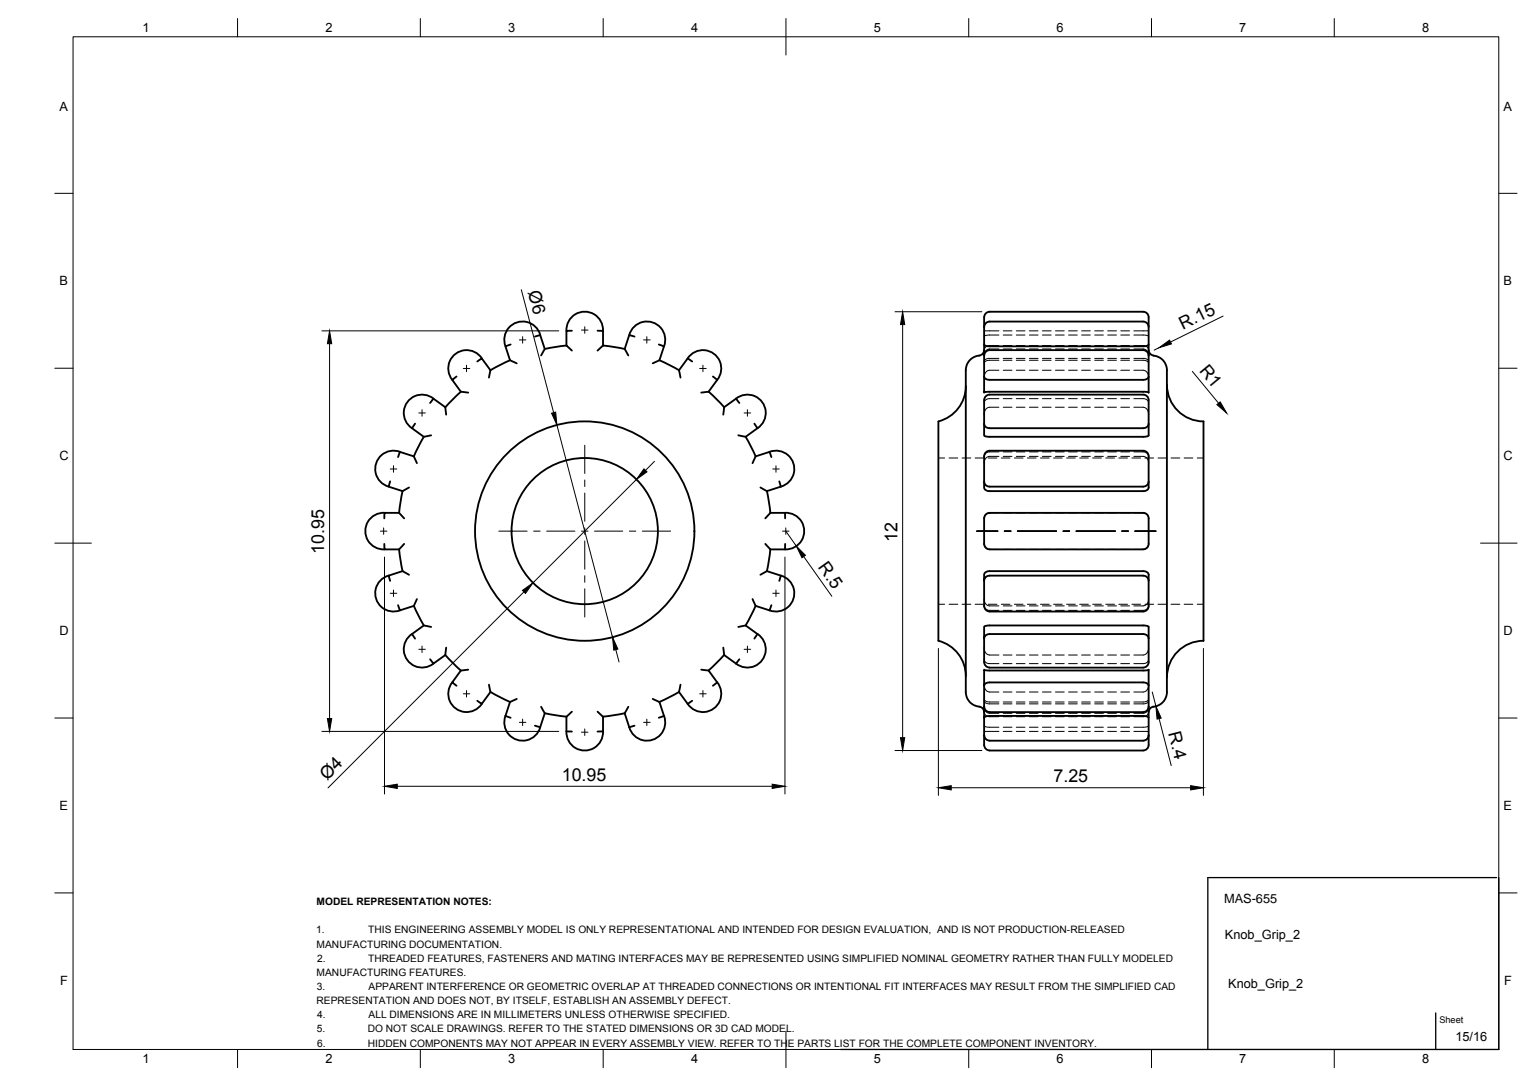
ISO-10303-21;
HEADER;
FILE_DESCRIPTION((''),'2;1');
FILE_NAME('Knob_Grip_2.step','2026-10-09T11:34:15-07:00',(''),(''),'','','');
FILE_SCHEMA (('AUTOMOTIVE_DESIGN { 1 0 10303 214 3 1 1 }'));
ENDSEC;
DATA;
#10=MECHANICAL_DESIGN_GEOMETRIC_PRESENTATION_REPRESENTATION('',(#647),#117170);
#605=SHAPE_REPRESENTATION_RELATIONSHIP('SRR','None',#117260,#626) ;
#626=ADVANCED_BREP_SHAPE_REPRESENTATION('',(#668),#117168) ;
#647=STYLED_ITEM('',(#117355),#668) ;
#668=MANIFOLD_SOLID_BREP('Body1',#49076) ;
#766=FACE_BOUND('',#16715,.T.) ;
#767=FACE_BOUND('',#16718,.T.) ;
#768=FACE_BOUND('',#16720,.T.) ;
#769=FACE_BOUND('',#16722,.T.) ;
#1529=B_SPLINE_CURVE_WITH_KNOTS('',3,(#105473,#105474,#105475,#105476,#105477,
#105478,#105479,#105480,#105481,#105482,#105483,#105484,#105485,#105486,
#105487,#105488,#105489),.UNSPECIFIED.,.T.,.F.,(4,1,1,1,1,1,1,1,1,1,1,1,
1,1,4),(-1.37470975898194,-1.17832265055595,-0.981935542129957,-0.785548433703966,
-0.589161325277974,-0.392774216851983,-0.196387108425991,0.,0.196387108425991,
0.392774216851983,0.589161325277974,0.785548433703966,0.981935542129957,
1.17832265055595,1.37470975898194),.UNSPECIFIED.) ;
#1530=B_SPLINE_CURVE_WITH_KNOTS('',3,(#105498,#105499,#105500,#105501,#105502,
#105503,#105504,#105505,#105506,#105507,#105508,#105509,#105510,#105511,
#105512,#105513,#105514),.UNSPECIFIED.,.T.,.F.,(4,1,1,1,1,1,1,1,1,1,1,1,
1,1,4),(-1.37470975898194,-1.17832265055595,-0.981935542129957,-0.785548433703966,
-0.589161325277974,-0.392774216851983,-0.196387108425991,0.,0.196387108425991,
0.392774216851983,0.589161325277974,0.785548433703966,0.981935542129957,
1.17832265055595,1.37470975898194),.UNSPECIFIED.) ;
#1531=B_SPLINE_CURVE_WITH_KNOTS('',3,(#105607,#105608,#105609,#105610,#105611),
 .UNSPECIFIED.,.F.,.F.,(4,1,4),(-1.,-0.5,0.),.UNSPECIFIED.) ;
#1532=B_SPLINE_CURVE_WITH_KNOTS('',3,(#105613,#105614,#105615,#105616,#105617,
#105618,#105619),.UNSPECIFIED.,.F.,.F.,(4,1,1,1,4),(-1.37470975898194,-1.17832265055595,
-0.981935542129957,-0.785548433703966,-0.687133244560913),.UNSPECIFIED.) ;
#1533=B_SPLINE_CURVE_WITH_KNOTS('',3,(#105620,#105621,#105622,#105623,#105624,
#105625,#105626,#105627,#105628,#105629,#105630,#105631,#105632,#105633),
 .UNSPECIFIED.,.F.,.F.,(4,1,1,1,1,1,1,1,1,1,1,4),(-0.687133244560913,-0.589161325277974,
-0.392774216851983,-0.196387108425991,0.,0.196387108425991,0.392774216851983,
0.589161325277974,0.785548433703966,0.981935542129957,1.17832265055595,
1.37470975898194),.UNSPECIFIED.) ;
#1534=B_SPLINE_CURVE_WITH_KNOTS('',3,(#105720,#105721,#105722,#105723,#105724),
 .UNSPECIFIED.,.F.,.F.,(4,1,4),(-1.,-0.5,0.),.UNSPECIFIED.) ;
#1535=B_SPLINE_CURVE_WITH_KNOTS('',3,(#105726,#105727,#105728,#105729,#105730,
#105731,#105732),.UNSPECIFIED.,.F.,.F.,(4,1,1,1,4),(-1.37470975898194,-1.17832265055595,
-0.981935542129957,-0.785548433703966,-0.687210817221059),.UNSPECIFIED.) ;
#1536=B_SPLINE_CURVE_WITH_KNOTS('',3,(#105733,#105734,#105735,#105736,#105737,
#105738,#105739,#105740,#105741,#105742,#105743,#105744,#105745,#105746),
 .UNSPECIFIED.,.F.,.F.,(4,1,1,1,1,1,1,1,1,1,1,4),(-0.687210817221059,-0.589161325277974,
-0.392774216851983,-0.196387108425991,0.,0.196387108425991,0.392774216851983,
0.589161325277974,0.785548433703966,0.981935542129957,1.17832265055595,
1.37470975898194),.UNSPECIFIED.) ;
#1537=B_SPLINE_CURVE_WITH_KNOTS('',3,(#105752,#105753,#105754,#105755,#105756,
#105757,#105758,#105759,#105760,#105761,#105762,#105763,#105764,#105765),
 .UNSPECIFIED.,.F.,.F.,(4,2,2,2,2,2,4),(-0.0559250143496373,-0.0556883945460747,
-0.0495906031992305,-0.0437546843030053,-0.0372885759081072,-0.0322854917709823,
-0.0278441972730634),.UNSPECIFIED.) ;
#1538=B_SPLINE_CURVE_WITH_KNOTS('',3,(#105768,#105769,#105770,#105771,#105772,
#105773,#105774,#105775,#105776,#105777,#105778,#105779,#105780,#105781),
 .UNSPECIFIED.,.F.,.F.,(4,2,2,2,2,2,4),(-0.000236619804093,0.,0.0060977913471935,
0.0119337102438738,0.018399818639261,0.0234029027767472,0.0278441972749678),
 .UNSPECIFIED.) ;
#1539=B_SPLINE_CURVE_WITH_KNOTS('',3,(#105786,#105787,#105788,#105789,#105790,
#105791,#105792,#105793,#105794,#105795,#105796,#105797,#105798,#105799,
#105800,#105801),.UNSPECIFIED.,.F.,.F.,(4,3,3,3,3,4),(-0.000437598556087367,
0.,0.00562170475705654,0.0114823251607832,0.0173413775084489,0.0231997078489075),
 .UNSPECIFIED.) ;
#1540=B_SPLINE_CURVE_WITH_KNOTS('',3,(#105807,#105808,#105809,#105810,#105811,
#105812,#105813,#105814,#105815,#105816,#105817,#105818,#105819,#105820,
#105821,#105822),.UNSPECIFIED.,.F.,.F.,(4,3,3,3,3,4),(-0.046837014255361,
-0.046399415699481,-0.0407777109422933,-0.0349170905383532,-0.0290580381904547,
-0.0231997078497599),.UNSPECIFIED.) ;
#1541=B_SPLINE_CURVE_WITH_KNOTS('',3,(#105828,#105829,#105830,#105831,#105832,
#105833,#105834,#105835,#105836,#105837,#105838,#105839,#105840,#105841),
 .UNSPECIFIED.,.F.,.F.,(4,2,2,2,2,2,4),(-0.000236619803146698,0.,0.00609779134724104,
0.0119337102438844,0.0183998186389394,0.0234029027761802,0.0278441972742087),
 .UNSPECIFIED.) ;
#1542=B_SPLINE_CURVE_WITH_KNOTS('',3,(#105847,#105848,#105849,#105850,#105851,
#105852,#105853,#105854,#105855,#105856,#105857,#105858,#105859,#105860),
 .UNSPECIFIED.,.F.,.F.,(4,2,2,2,2,2,4),(-0.0559250143496986,-0.0556883945465552,
-0.0495906031994403,-0.0437546843028884,-0.0372885759079096,-0.0322854917707418,
-0.0278441972727803),.UNSPECIFIED.) ;
#1543=B_SPLINE_CURVE_WITH_KNOTS('',3,(#105866,#105867,#105868,#105869,#105870,
#105871,#105872,#105873,#105874,#105875,#105876,#105877,#105878,#105879,
#105880,#105881),.UNSPECIFIED.,.F.,.F.,(4,3,3,3,3,4),(-0.000437598556095027,
0.,0.00562170475708189,0.0114823251608833,0.0173413775086171,0.0231997078491342),
 .UNSPECIFIED.) ;
#1544=B_SPLINE_CURVE_WITH_KNOTS('',3,(#105887,#105888,#105889,#105890,#105891,
#105892,#105893,#105894,#105895,#105896,#105897,#105898,#105899,#105900,
#105901,#105902),.UNSPECIFIED.,.F.,.F.,(4,3,3,3,3,4),(-0.0468370142541051,
-0.0463994156980201,-0.0407777109409428,-0.0349170905371886,-0.0290580381894966,
-0.0231997078490079),.UNSPECIFIED.) ;
#1545=B_SPLINE_CURVE_WITH_KNOTS('',3,(#105908,#105909,#105910,#105911,#105912,
#105913,#105914,#105915,#105916,#105917,#105918,#105919,#105920,#105921),
 .UNSPECIFIED.,.F.,.F.,(4,2,2,2,2,2,4),(-0.000236619803558265,0.,0.00609779134685418,
0.0119337102431074,0.0183998186379772,0.023402902775095,0.0278441972730209),
 .UNSPECIFIED.) ;
#1546=B_SPLINE_CURVE_WITH_KNOTS('',3,(#105927,#105928,#105929,#105930,#105931,
#105932,#105933,#105934,#105935,#105936,#105937,#105938,#105939,#105940),
 .UNSPECIFIED.,.F.,.F.,(4,2,2,2,2,2,4),(-0.0559250143504567,-0.0556883945473107,
-0.0495906032000867,-0.0437546843034773,-0.0372885759084374,-0.0322854917711889,
-0.0278441972731474),.UNSPECIFIED.) ;
#1547=B_SPLINE_CURVE_WITH_KNOTS('',3,(#105946,#105947,#105948,#105949,#105950,
#105951,#105952,#105953,#105954,#105955,#105956,#105957,#105958,#105959,
#105960,#105961),.UNSPECIFIED.,.F.,.F.,(4,3,3,3,3,4),(-0.000437598556114517,
0.,0.00562170475723958,0.0114823251612343,0.0173413775091901,0.0231997078499022),
 .UNSPECIFIED.) ;
#1548=B_SPLINE_CURVE_WITH_KNOTS('',3,(#105967,#105968,#105969,#105970,#105971,
#105972,#105973,#105974,#105975,#105976,#105977,#105978,#105979,#105980,
#105981,#105982),.UNSPECIFIED.,.F.,.F.,(4,3,3,3,3,4),(-0.0468370142517104,
-0.046399415695612,-0.0407777109388244,-0.034917090535398,-0.0290580381880315,
-0.0231997078478665),.UNSPECIFIED.) ;
#1549=B_SPLINE_CURVE_WITH_KNOTS('',3,(#105988,#105989,#105990,#105991,#105992,
#105993,#105994,#105995,#105996,#105997,#105998,#105999,#106000,#106001),
 .UNSPECIFIED.,.F.,.F.,(4,2,2,2,2,2,4),(-0.000236619803559768,0.,0.00609779134686269,
0.0119337102430971,0.0183998186379832,0.0234029027750867,0.0278441972729811),
 .UNSPECIFIED.) ;
#1550=B_SPLINE_CURVE_WITH_KNOTS('',3,(#106007,#106008,#106009,#106010,#106011,
#106012,#106013,#106014,#106015,#106016,#106017,#106018,#106019,#106020),
 .UNSPECIFIED.,.F.,.F.,(4,2,2,2,2,2,4),(-0.0559250143524368,-0.0556883945478243,
-0.0495906032010392,-0.0437546843047665,-0.0372885759096309,-0.0322854917723447,
-0.0278441972742818),.UNSPECIFIED.) ;
#1551=B_SPLINE_CURVE_WITH_KNOTS('',3,(#106026,#106027,#106028,#106029,#106030,
#106031,#106032,#106033,#106034,#106035,#106036,#106037,#106038,#106039,
#106040,#106041),.UNSPECIFIED.,.F.,.F.,(4,3,3,3,3,4),(-0.000437598556131605,
0.,0.00562170475733242,0.0114823251614144,0.0173413775094361,0.0231997078502398),
 .UNSPECIFIED.) ;
#1552=B_SPLINE_CURVE_WITH_KNOTS('',3,(#106047,#106048,#106049,#106050,#106051,
#106052,#106053,#106054,#106055,#106056,#106057,#106058,#106059,#106060,
#106061,#106062),.UNSPECIFIED.,.F.,.F.,(4,3,3,3,3,4),(-0.046837014258247,
-0.0463994157019922,-0.0407777109444557,-0.0349170905401249,-0.0290580381918459,
-0.0231997078507989),.UNSPECIFIED.) ;
#1553=B_SPLINE_CURVE_WITH_KNOTS('',3,(#106068,#106069,#106070,#106071,#106072,
#106073,#106074,#106075,#106076,#106077,#106078,#106079,#106080,#106081),
 .UNSPECIFIED.,.F.,.F.,(4,2,2,2,2,2,4),(-0.000236619803154501,0.,0.00609779134749395,
0.0119337102444787,0.0183998186399401,0.0234029027774939,0.0278441972757804),
 .UNSPECIFIED.) ;
#1554=B_SPLINE_CURVE_WITH_KNOTS('',3,(#106087,#106088,#106089,#106090,#106091,
#106092,#106093,#106094,#106095,#106096,#106097,#106098,#106099,#106100),
 .UNSPECIFIED.,.F.,.F.,(4,2,2,2,2,2,4),(-0.0559250143516698,-0.055688394548102,
-0.0495906032010132,-0.0437546843045191,-0.0372885759093257,-0.0322854917720022,
-0.0278441972739074),.UNSPECIFIED.) ;
#1555=B_SPLINE_CURVE_WITH_KNOTS('',3,(#106106,#106107,#106108,#106109,#106110,
#106111,#106112,#106113,#106114,#106115,#106116,#106117,#106118,#106119,
#106120,#106121),.UNSPECIFIED.,.F.,.F.,(4,3,3,3,3,4),(-0.000437598556150276,
0.,0.00562170475744494,0.0114823251616921,0.0173413775098778,0.0231997078508276),
 .UNSPECIFIED.) ;
#1556=B_SPLINE_CURVE_WITH_KNOTS('',3,(#106127,#106128,#106129,#106130,#106131,
#106132,#106133,#106134,#106135,#106136,#106137,#106138,#106139,#106140,
#106141,#106142),.UNSPECIFIED.,.F.,.F.,(4,3,3,3,3,4),(-0.0468370142569828,
-0.0463994157014635,-0.0407777109440522,-0.0349170905398014,-0.0290580381915951,
-0.0231997078506218),.UNSPECIFIED.) ;
#1557=B_SPLINE_CURVE_WITH_KNOTS('',3,(#106148,#106149,#106150,#106151,#106152,
#106153,#106154,#106155,#106156,#106157,#106158,#106159,#106160,#106161),
 .UNSPECIFIED.,.F.,.F.,(4,2,2,2,2,2,4),(-0.000236619804616541,0.,0.00609779134700319,
0.0119337102434886,0.0183998186388943,0.0234029027763847,0.0278441972746185),
 .UNSPECIFIED.) ;
#1558=B_SPLINE_CURVE_WITH_KNOTS('',3,(#106167,#106168,#106169,#106170,#106171,
#106172,#106173,#106174,#106175,#106176,#106177,#106178,#106179,#106180),
 .UNSPECIFIED.,.F.,.F.,(4,2,2,2,2,2,4),(-0.0559250143475551,-0.0556883945439973,
-0.049590603197355,-0.0437546843013896,-0.037288575906807,-0.0322854917699323,
-0.0278441972722247),.UNSPECIFIED.) ;
#1559=B_SPLINE_CURVE_WITH_KNOTS('',3,(#106186,#106187,#106188,#106189,#106190,
#106191,#106192,#106193,#106194,#106195,#106196,#106197,#106198,#106199,
#106200,#106201),.UNSPECIFIED.,.F.,.F.,(4,3,3,3,3,4),(-0.000437598556056009,
0.,0.00562170475686937,0.0114823251603833,0.0173413775078316,0.0231997078480834),
 .UNSPECIFIED.) ;
#1560=B_SPLINE_CURVE_WITH_KNOTS('',3,(#106207,#106208,#106209,#106210,#106211,
#106212,#106213,#106214,#106215,#106216,#106217,#106218,#106219,#106220,
#106221,#106222),.UNSPECIFIED.,.F.,.F.,(4,3,3,3,3,4),(-0.0468370142561097,
-0.0463994157004828,-0.0407777109431283,-0.034917090538975,-0.0290580381908889,
-0.0231997078500392),.UNSPECIFIED.) ;
#1561=B_SPLINE_CURVE_WITH_KNOTS('',3,(#106228,#106229,#106230,#106231,#106232,
#106233,#106234,#106235,#106236,#106237,#106238,#106239,#106240,#106241),
 .UNSPECIFIED.,.F.,.F.,(4,2,2,2,2,2,4),(-0.000236619804206572,0.,0.00609779134739848,
0.0119337102443252,0.0183998186399927,0.023402902777706,0.0278441972760964),
 .UNSPECIFIED.) ;
#1562=B_SPLINE_CURVE_WITH_KNOTS('',3,(#106247,#106248,#106249,#106250,#106251,
#106252,#106253,#106254,#106255,#106256,#106257,#106258,#106259,#106260),
 .UNSPECIFIED.,.F.,.F.,(4,2,2,2,2,2,4),(-0.0559250143503367,-0.0556883945467745,
-0.0495906031998185,-0.0437546843034772,-0.0372885759085197,-0.0322854917713411,
-0.0278441972733722),.UNSPECIFIED.) ;
#1563=B_SPLINE_CURVE_WITH_KNOTS('',3,(#106266,#106267,#106268,#106269,#106270,
#106271,#106272,#106273,#106274,#106275,#106276,#106277,#106278,#106279,
#106280,#106281),.UNSPECIFIED.,.F.,.F.,(4,3,3,3,3,4),(-0.000437598556095159,
0.,0.00562170475710087,0.0114823251609001,0.0173413775086179,0.0231997078491324),
 .UNSPECIFIED.) ;
#1564=B_SPLINE_CURVE_WITH_KNOTS('',3,(#106287,#106288,#106289,#106290,#106291,
#106292,#106293,#106294,#106295,#106296,#106297,#106298,#106299,#106300,
#106301,#106302),.UNSPECIFIED.,.F.,.F.,(4,3,3,3,3,4),(-0.0468370142542446,
-0.0463994156981747,-0.0407777109410807,-0.0349170905373078,-0.0290580381895938,
-0.0231997078490836),.UNSPECIFIED.) ;
#1565=B_SPLINE_CURVE_WITH_KNOTS('',3,(#106308,#106309,#106310,#106311,#106312,
#106313,#106314,#106315,#106316,#106317,#106318,#106319,#106320,#106321),
 .UNSPECIFIED.,.F.,.F.,(4,2,2,2,2,2,4),(-0.000236619803563725,0.,0.00609779134693619,
0.0119337102432759,0.0183998186382373,0.0234029027754271,0.027844197273412),
 .UNSPECIFIED.) ;
#1566=B_SPLINE_CURVE_WITH_KNOTS('',3,(#106327,#106328,#106329,#106330,#106331,
#106332,#106333,#106334,#106335,#106336,#106337,#106338,#106339,#106340),
 .UNSPECIFIED.,.F.,.F.,(4,2,2,2,2,2,4),(-0.0559250143564113,-0.0556883945522011,
-0.0495906032047249,-0.0437546843077159,-0.0372885759119513,-0.0322854917741759,
-0.0278441972757216),.UNSPECIFIED.) ;
#1567=B_SPLINE_CURVE_WITH_KNOTS('',3,(#106346,#106347,#106348,#106349,#106350,
#106351,#106352,#106353,#106354,#106355,#106356,#106357,#106358,#106359,
#106360,#106361),.UNSPECIFIED.,.F.,.F.,(4,3,3,3,3,4),(-0.000437598556252948,
0.,0.00562170475756358,0.0114823251619473,0.0173413775102792,0.023199707851373),
 .UNSPECIFIED.) ;
#1568=B_SPLINE_CURVE_WITH_KNOTS('',3,(#106367,#106368,#106369,#106370,#106371,
#106372,#106373,#106374,#106375,#106376,#106377,#106378,#106379,#106380,
#106381,#106382),.UNSPECIFIED.,.F.,.F.,(4,3,3,3,3,4),(-0.0468370142435449,
-0.0463994156880452,-0.0407777109322271,-0.0349170905298351,-0.0290580381834779,
-0.0231997078443083),.UNSPECIFIED.) ;
#1569=B_SPLINE_CURVE_WITH_KNOTS('',3,(#106388,#106389,#106390,#106391,#106392,
#106393,#106394,#106395,#106396,#106397,#106398,#106399,#106400,#106401),
 .UNSPECIFIED.,.F.,.F.,(4,2,2,2,2,2,4),(-0.000236619803545348,0.,0.00609779134648851,
0.0119337102422953,0.0183998186366923,0.0234029027734222,0.0278441972710204),
 .UNSPECIFIED.) ;
#1570=B_SPLINE_CURVE_WITH_KNOTS('',3,(#106407,#106408,#106409,#106410,#106411,
#106412,#106413,#106414,#106415,#106416,#106417,#106418,#106419,#106420),
 .UNSPECIFIED.,.F.,.F.,(4,2,2,2,2,2,4),(-0.0559250143495547,-0.0556883945459923,
-0.0495906031991245,-0.0437546843029074,-0.0372885759080479,-0.0322854917709575,
-0.027844197273083),.UNSPECIFIED.) ;
#1571=B_SPLINE_CURVE_WITH_KNOTS('',3,(#106426,#106427,#106428,#106429,#106430,
#106431,#106432,#106433,#106434,#106435,#106436,#106437,#106438,#106439,
#106440,#106441),.UNSPECIFIED.,.F.,.F.,(4,3,3,3,3,4),(-0.000437598556080383,
0.,0.00562170475701161,0.0114823251606741,0.0173413775082905,0.0231997078487108),
 .UNSPECIFIED.) ;
#1572=B_SPLINE_CURVE_WITH_KNOTS('',3,(#106447,#106448,#106449,#106450,#106451,
#106452,#106453,#106454,#106455,#106456,#106457,#106458,#106459,#106460,
#106461,#106462),.UNSPECIFIED.,.F.,.F.,(4,3,3,3,3,4),(-0.0468370142410635,
-0.046399415685515,-0.0407777109299654,-0.0349170905279156,-0.0290580381819153,
-0.0231997078430871),.UNSPECIFIED.) ;
#1573=B_SPLINE_CURVE_WITH_KNOTS('',3,(#106468,#106469,#106470,#106471,#106472,
#106473,#106474,#106475,#106476,#106477,#106478,#106479,#106480,#106481),
 .UNSPECIFIED.,.F.,.F.,(4,2,2,2,2,2,4),(-0.000236619803553881,0.,0.00609779134648714,
0.0119337102422593,0.0183998186365944,0.0234029027733178,0.0278441972709114),
 .UNSPECIFIED.) ;
#1574=B_SPLINE_CURVE_WITH_KNOTS('',3,(#106487,#106488,#106489,#106490,#106491,
#106492,#106493,#106494,#106495,#106496,#106497,#106498,#106499,#106500),
 .UNSPECIFIED.,.F.,.F.,(4,2,2,2,2,2,4),(-0.0559250143458346,-0.0556883945427038,
-0.0495906031960554,-0.043754684300065,-0.0372885759056522,-0.0322854917688908,
-0.0278441972712752),.UNSPECIFIED.) ;
#1575=B_SPLINE_CURVE_WITH_KNOTS('',3,(#106506,#106507,#106508,#106509,#106510,
#106511,#106512,#106513,#106514,#106515,#106516,#106517,#106518,#106519,
#106520,#106521),.UNSPECIFIED.,.F.,.F.,(4,3,3,3,3,4),(-0.000437598556037642,
0.,0.00562170475676515,0.0114823251601515,0.0173413775075229,0.0231997078477011),
 .UNSPECIFIED.) ;
#1576=B_SPLINE_CURVE_WITH_KNOTS('',3,(#106527,#106528,#106529,#106530,#106531,
#106532,#106533,#106534,#106535,#106536,#106537,#106538,#106539,#106540,
#106541,#106542),.UNSPECIFIED.,.F.,.F.,(4,3,3,3,3,4),(-0.0468370142550307,
-0.046399415699245,-0.0407777109420836,-0.0349170905381485,-0.0290580381902572,
-0.023199707849583),.UNSPECIFIED.) ;
#1577=B_SPLINE_CURVE_WITH_KNOTS('',3,(#106548,#106549,#106550,#106551,#106552,
#106553,#106554,#106555,#106556,#106557,#106558,#106559,#106560,#106561),
 .UNSPECIFIED.,.F.,.F.,(4,2,2,2,2,2,4),(-0.000236619803565948,0.,0.00609779134700125,
0.0119337102434307,0.0183998186384978,0.0234029027757452,0.0278441972737845),
 .UNSPECIFIED.) ;
#1578=B_SPLINE_CURVE_WITH_KNOTS('',3,(#106567,#106568,#106569,#106570,#106571,
#106572,#106573,#106574,#106575,#106576,#106577,#106578,#106579,#106580),
 .UNSPECIFIED.,.F.,.F.,(4,2,2,2,2,2,4),(-0.0559250143492506,-0.0556883945457476,
-0.049590603198939,-0.0437546843027145,-0.0372885759078682,-0.032285491770796,
-0.0278441972729179),.UNSPECIFIED.) ;
#1579=B_SPLINE_CURVE_WITH_KNOTS('',3,(#106587,#106588,#106589,#106590,#106591,
#106592,#106593,#106594,#106595,#106596,#106597,#106598,#106599,#106600,
#106601,#106602),.UNSPECIFIED.,.F.,.F.,(4,3,3,3,3,4),(-0.000437598556107252,
0.,0.00562170475708925,0.0114823251608564,0.0173413775085622,0.0231997078490661),
 .UNSPECIFIED.) ;
#1580=B_SPLINE_CURVE_WITH_KNOTS('',3,(#106608,#106609,#106610,#106611,#106612,
#106613,#106614,#106615,#106616,#106617,#106618,#106619,#106620,#106621,
#106622,#106623),.UNSPECIFIED.,.F.,.F.,(4,3,3,3,3,4),(-0.0468370142553995,
-0.0463994157003126,-0.0407777109430307,-0.0349170905389541,-0.0290580381909493,
-0.0231997078501516),.UNSPECIFIED.) ;
#1581=B_SPLINE_CURVE_WITH_KNOTS('',3,(#106629,#106630,#106631,#106632,#106633,
#106634,#106635,#106636,#106637,#106638,#106639,#106640,#106641,#106642),
 .UNSPECIFIED.,.F.,.F.,(4,2,2,2,2,2,4),(-0.000236619803559952,0.,0.00609779134694098,
0.0119337102432763,0.0183998186382272,0.0234029027754186,0.0278441972733939),
 .UNSPECIFIED.) ;
#1582=B_SPLINE_CURVE_WITH_KNOTS('',3,(#106648,#106649,#106650,#106651,#106652,
#106653,#106654,#106655,#106656,#106657,#106658,#106659,#106660,#106661),
 .UNSPECIFIED.,.F.,.F.,(4,2,2,2,2,2,4),(-0.0559250143507825,-0.0556883945467992,
-0.0495906032001226,-0.043754684304009,-0.0372885759090493,-0.032285491771857,
-0.0278441972738728),.UNSPECIFIED.) ;
#1583=B_SPLINE_CURVE_WITH_KNOTS('',3,(#106667,#106668,#106669,#106670,#106671,
#106672,#106673,#106674,#106675,#106676,#106677,#106678,#106679,#106680,
#106681,#106682),.UNSPECIFIED.,.F.,.F.,(4,3,3,3,3,4),(-0.000437598556095639,
0.,0.00562170475706734,0.0114823251608502,0.0173413775085488,0.0231997078490271),
 .UNSPECIFIED.) ;
#1584=B_SPLINE_CURVE_WITH_KNOTS('',3,(#106688,#106689,#106690,#106691,#106692,
#106693,#106694,#106695,#106696,#106697,#106698,#106699,#106700,#106701,
#106702,#106703),.UNSPECIFIED.,.F.,.F.,(4,3,3,3,3,4),(-0.0468370142543074,
-0.0463994156982126,-0.0407777109411238,-0.0349170905373201,-0.0290580381896051,
-0.0231997078491063),.UNSPECIFIED.) ;
#1585=B_SPLINE_CURVE_WITH_KNOTS('',3,(#106709,#106710,#106711,#106712,#106713,
#106714,#106715,#106716,#106717,#106718,#106719,#106720,#106721,#106722),
 .UNSPECIFIED.,.F.,.F.,(4,2,2,2,2,2,4),(-0.000236619803981649,0.,0.00609779134664719,
0.0119337102427236,0.0183998186376455,0.0234029027747974,0.0278441972727449),
 .UNSPECIFIED.) ;
#1586=B_SPLINE_CURVE_WITH_KNOTS('',3,(#106728,#106729,#106730,#106731,#106732,
#106733,#106734,#106735,#106736,#106737,#106738,#106739,#106740,#106741),
 .UNSPECIFIED.,.F.,.F.,(4,2,2,2,2,2,4),(-0.055925014352087,-0.0556883945480977,
-0.0495906032012405,-0.0437546843049561,-0.0372885759098064,-0.0322854917724869,
-0.0278441972743996),.UNSPECIFIED.) ;
#1587=B_SPLINE_CURVE_WITH_KNOTS('',3,(#106747,#106748,#106749,#106750,#106751,
#106752,#106753,#106754,#106755,#106756,#106757,#106758,#106759,#106760,
#106761,#106762),.UNSPECIFIED.,.F.,.F.,(4,3,3,3,3,4),(-0.000437598556128711,
0.,0.00562170475726701,0.0114823251612751,0.0173413775092439,0.0231997078500064),
 .UNSPECIFIED.) ;
#1588=B_SPLINE_CURVE_WITH_KNOTS('',3,(#106768,#106769,#106770,#106771,#106772,
#106773,#106774,#106775,#106776,#106777,#106778,#106779,#106780,#106781,
#106782,#106783),.UNSPECIFIED.,.F.,.F.,(4,3,3,3,3,4),(-0.0468370142525421,
-0.046399415696666,-0.0407777109397685,-0.0349170905362003,-0.029058038188693,
-0.0231997078483865),.UNSPECIFIED.) ;
#1589=B_SPLINE_CURVE_WITH_KNOTS('',3,(#106789,#106790,#106791,#106792,#106793,
#106794,#106795,#106796,#106797,#106798,#106799,#106800,#106801,#106802),
 .UNSPECIFIED.,.F.,.F.,(4,2,2,2,2,2,4),(-0.000236619803982414,0.,0.00609779134661,
0.0119337102426289,0.0183998186375097,0.0234029027746178,0.0278441972725225),
 .UNSPECIFIED.) ;
#1590=B_SPLINE_CURVE_WITH_KNOTS('',3,(#106808,#106809,#106810,#106811,#106812,
#106813,#106814,#106815,#106816,#106817,#106818,#106819,#106820,#106821),
 .UNSPECIFIED.,.F.,.F.,(4,2,2,2,2,2,4),(-0.0559250143493171,-0.0556883945461739,
-0.0495906031990541,-0.0437546843026118,-0.037288575907723,-0.0322854917706097,
-0.0278441972727174),.UNSPECIFIED.) ;
#1591=B_SPLINE_CURVE_WITH_KNOTS('',3,(#106827,#106828,#106829,#106830,#106831,
#106832,#106833,#106834,#106835,#106836,#106837,#106838,#106839,#106840,
#106841,#106842),.UNSPECIFIED.,.F.,.F.,(4,3,3,3,3,4),(-0.000437598556087196,
0.,0.00562170475699019,0.0114823251606472,0.0173413775082489,0.0231997078486377),
 .UNSPECIFIED.) ;
#1592=B_SPLINE_CURVE_WITH_KNOTS('',3,(#106848,#106849,#106850,#106851,#106852,
#106853,#106854,#106855,#106856,#106857,#106858,#106859,#106860,#106861,
#106862,#106863),.UNSPECIFIED.,.F.,.F.,(4,3,3,3,3,4),(-0.0468370142500863,
-0.0463994156945211,-0.0407777109379294,-0.0349170905346585,-0.0290580381874365,
-0.0231997078474141),.UNSPECIFIED.) ;
#1593=B_SPLINE_CURVE_WITH_KNOTS('',3,(#106869,#106870,#106871,#106872,#106873,
#106874,#106875,#106876,#106877,#106878,#106879,#106880,#106881,#106882),
 .UNSPECIFIED.,.F.,.F.,(4,2,2,2,2,2,4),(-0.000236619803560014,0.,0.00609779134678491,
0.0119337102429536,0.0183998186377476,0.0234029027747679,0.0278441972725981),
 .UNSPECIFIED.) ;
#1594=B_SPLINE_CURVE_WITH_KNOTS('',3,(#106888,#106889,#106890,#106891,#106892,
#106893,#106894,#106895,#106896,#106897,#106898,#106899,#106900,#106901),
 .UNSPECIFIED.,.F.,.F.,(4,2,2,2,2,2,4),(-0.0559250143548778,-0.0556883945506748,
-0.0495906032033264,-0.0437546843064839,-0.0372885759109464,-0.0322854917733345,
-0.0278441972750097),.UNSPECIFIED.) ;
#1595=B_SPLINE_CURVE_WITH_KNOTS('',3,(#106907,#106908,#106909,#106910,#106911,
#106912,#106913,#106914,#106915,#106916,#106917,#106918,#106919,#106920,
#106921,#106922),.UNSPECIFIED.,.F.,.F.,(4,3,3,3,3,4),(-0.000437598556223204,
0.,0.00562170475783914,0.0114823251625445,0.0173413775111918,0.0231997078526027),
 .UNSPECIFIED.) ;
#1596=B_SPLINE_CURVE_WITH_KNOTS('',3,(#106928,#106929,#106930,#106931,#106932,
#106933,#106934,#106935,#106936,#106937,#106938,#106939,#106940,#106941,
#106942,#106943),.UNSPECIFIED.,.F.,.F.,(4,3,3,3,3,4),(-0.0468370142563843,
-0.046399415700489,-0.0407777109431322,-0.0349170905389995,-0.0290580381909307,
-0.0231997078501088),.UNSPECIFIED.) ;
#1597=B_SPLINE_CURVE_WITH_KNOTS('',3,(#106949,#106950,#106951,#106952,#106953,
#106954,#106955,#106956,#106957,#106958,#106959,#106960,#106961,#106962),
 .UNSPECIFIED.,.F.,.F.,(4,2,2,2,2,2,4),(-0.000236619804200277,0.,0.00609779134716414,
0.0119337102438048,0.0183998186391783,0.0234029027766296,0.0278441972748296),
 .UNSPECIFIED.) ;
#1598=B_SPLINE_CURVE_WITH_KNOTS('',3,(#106968,#106969,#106970,#106971,#106972,
#106973,#106974,#106975,#106976,#106977,#106978,#106979,#106980,#106981),
 .UNSPECIFIED.,.F.,.F.,(4,2,2,2,2,2,4),(-0.0559250143496621,-0.0556883945461033,
-0.0495906031992651,-0.0437546843029983,-0.0372885759081094,-0.032285491771005,
-0.02784419727311),.UNSPECIFIED.) ;
#1599=B_SPLINE_CURVE_WITH_KNOTS('',3,(#106987,#106988,#106989,#106990,#106991,
#106992,#106993,#106994,#106995,#106996,#106997,#106998,#106999,#107000,
#107001,#107002),.UNSPECIFIED.,.F.,.F.,(4,3,3,3,3,4),(-0.000437598556084584,
0.,0.00562170475697965,0.0114823251606079,0.0173413775081775,0.0231997078485472),
 .UNSPECIFIED.) ;
#1600=B_SPLINE_CURVE_WITH_KNOTS('',3,(#107008,#107009,#107010,#107011,#107012,
#107013,#107014,#107015,#107016,#107017,#107018,#107019,#107020,#107021,
#107022,#107023),.UNSPECIFIED.,.F.,.F.,(4,3,3,3,3,4),(-0.0468370142549382,
-0.0463994156994604,-0.0407777109422707,-0.0349170905383382,-0.0290580381904463,
-0.023199707849757),.UNSPECIFIED.) ;
#1601=B_SPLINE_CURVE_WITH_KNOTS('',3,(#107029,#107030,#107031,#107032,#107033,
#107034,#107035,#107036,#107037,#107038,#107039,#107040,#107041,#107042),
 .UNSPECIFIED.,.F.,.F.,(4,2,2,2,2,2,4),(-0.000236619803568316,0.,0.00609779134701837,
0.0119337102434465,0.0183998186385035,0.0234029027757473,0.0278441972737745),
 .UNSPECIFIED.) ;
#1602=B_SPLINE_CURVE_WITH_KNOTS('',3,(#107048,#107049,#107050,#107051,#107052,
#107053,#107054,#107055,#107056,#107057,#107058,#107059,#107060,#107061),
 .UNSPECIFIED.,.F.,.F.,(4,2,2,2,2,2,4),(-0.0559250143499934,-0.0556883945464304,
-0.0495906031995064,-0.0437546843032007,-0.037288575908277,-0.032285491771123,
-0.0278441972731808),.UNSPECIFIED.) ;
#1603=B_SPLINE_CURVE_WITH_KNOTS('',3,(#107067,#107068,#107069,#107070,#107071,
#107072,#107073,#107074,#107075,#107076,#107077,#107078,#107079,#107080,
#107081,#107082),.UNSPECIFIED.,.F.,.F.,(4,3,3,3,3,4),(-0.000437598556092419,
0.,0.00562170475702671,0.0114823251607112,0.0173413775083605,0.0231997078487915),
 .UNSPECIFIED.) ;
#1604=B_SPLINE_CURVE_WITH_KNOTS('',3,(#107088,#107089,#107090,#107091,#107092,
#107093,#107094,#107095,#107096,#107097,#107098,#107099,#107100,#107101,
#107102,#107103),.UNSPECIFIED.,.F.,.F.,(4,3,3,3,3,4),(-0.0468370142548351,
-0.0463994156987323,-0.0407777109416122,-0.0349170905377609,-0.0290580381899607,
-0.0231997078493697),.UNSPECIFIED.) ;
#1605=B_SPLINE_CURVE_WITH_KNOTS('',3,(#107109,#107110,#107111,#107112,#107113,
#107114,#107115,#107116,#107117,#107118,#107119,#107120,#107121,#107122),
 .UNSPECIFIED.,.F.,.F.,(4,2,2,2,2,2,4),(-0.000236619803562033,0.,0.00609779134691358,
0.0119337102432247,0.0183998186381566,0.0234029027753094,0.027844197273255),
 .UNSPECIFIED.) ;
#1606=B_SPLINE_CURVE_WITH_KNOTS('',3,(#107128,#107129,#107130,#107131,#107132,
#107133,#107134,#107135,#107136,#107137,#107138,#107139,#107140,#107141),
 .UNSPECIFIED.,.F.,.F.,(4,2,2,2,2,2,4),(-0.0559250143503813,-0.0556883945472345,
-0.0495906032000065,-0.0437546843033907,-0.0372885759083472,-0.0322854917711086,
-0.027844197273083),.UNSPECIFIED.) ;
#1607=B_SPLINE_CURVE_WITH_KNOTS('',3,(#107147,#107148,#107149,#107150,#107151,
#107152,#107153,#107154,#107155,#107156,#107157,#107158,#107159,#107160,
#107161,#107162),.UNSPECIFIED.,.F.,.F.,(4,3,3,3,3,4),(-0.000437598556129241,
0.,0.00562170475730571,0.0114823251613513,0.0173413775093445,0.0231997078501172),
 .UNSPECIFIED.) ;
#1608=B_SPLINE_CURVE_WITH_KNOTS('',3,(#107168,#107169,#107170,#107171,#107172,
#107173,#107174,#107175,#107176,#107177,#107178,#107179,#107180,#107181,
#107182,#107183),.UNSPECIFIED.,.F.,.F.,(4,3,3,3,3,4),(-0.0468370142515845,
-0.0463994156955989,-0.0407777109388572,-0.0349170905354382,-0.0290580381880585,
-0.0231997078478789),.UNSPECIFIED.) ;
#1609=B_SPLINE_CURVE_WITH_KNOTS('',3,(#107189,#107190,#107191,#107192,#107193,
#107194,#107195,#107196,#107197,#107198,#107199,#107200,#107201,#107202),
 .UNSPECIFIED.,.F.,.F.,(4,2,2,2,2,2,4),(-0.000236619803559663,0.,0.0060977913468164,
0.0119337102430072,0.0183998186378663,0.0234029027749556,0.0278441972728503),
 .UNSPECIFIED.) ;
#1610=B_SPLINE_CURVE_WITH_KNOTS('',3,(#107208,#107209,#107210,#107211,#107212,
#107213,#107214,#107215,#107216,#107217,#107218,#107219,#107220,#107221),
 .UNSPECIFIED.,.F.,.F.,(4,2,2,2,2,2,4),(-0.0559250143533661,-0.0556883945491649,
-0.0495906032019838,-0.0437546843053393,-0.0372885759099808,-0.0322854917725361,
-0.0278441972743507),.UNSPECIFIED.) ;
#1611=B_SPLINE_CURVE_WITH_KNOTS('',3,(#107227,#107228,#107229,#107230,#107231,
#107232,#107233,#107234,#107235,#107236,#107237,#107238,#107239,#107240,
#107241,#107242),.UNSPECIFIED.,.F.,.F.,(4,3,3,3,3,4),(-0.00043759855615984,
0.,0.00562170475737693,0.011482325161534,0.017341377509665,0.0231997078505602),
 .UNSPECIFIED.) ;
#1612=B_SPLINE_CURVE_WITH_KNOTS('',3,(#107248,#107249,#107250,#107251,#107252,
#107253,#107254,#107255,#107256,#107257,#107258,#107259,#107260,#107261,
#107262,#107263),.UNSPECIFIED.,.F.,.F.,(4,3,3,3,3,4),(-0.0468370142504407,
-0.0463994156944377,-0.0407777109378315,-0.0349170905345851,-0.0290580381873817,
-0.0231997078473671),.UNSPECIFIED.) ;
#1613=B_SPLINE_CURVE_WITH_KNOTS('',3,(#107269,#107270,#107271,#107272,#107273,
#107274,#107275,#107276,#107277,#107278,#107279,#107280,#107281,#107282),
 .UNSPECIFIED.,.F.,.F.,(4,2,2,2,2,2,4),(-0.000236619803559426,0.,0.00609779134674399,
0.0119337102428204,0.0183998186375428,0.0234029027745216,0.0278441972723019),
 .UNSPECIFIED.) ;
#1614=B_SPLINE_CURVE_WITH_KNOTS('',3,(#107288,#107289,#107290,#107291,#107292,
#107293,#107294,#107295,#107296,#107297,#107298,#107299,#107300,#107301),
 .UNSPECIFIED.,.F.,.F.,(4,2,2,2,2,2,4),(-0.0559250143520313,-0.0556883945484605,
-0.0495906032013131,-0.0437546843047777,-0.037288575909542,-0.0322854917721873,
-0.0278441972740755),.UNSPECIFIED.) ;
#1615=B_SPLINE_CURVE_WITH_KNOTS('',3,(#107307,#107308,#107309,#107310,#107311,
#107312,#107313,#107314,#107315,#107316,#107317,#107318,#107319,#107320,
#107321,#107322),.UNSPECIFIED.,.F.,.F.,(4,3,3,3,3,4),(-0.000437598556142791,
0.,0.00562170475737048,0.011482325161532,0.0173413775096432,0.0231997078505159),
 .UNSPECIFIED.) ;
#1616=B_SPLINE_CURVE_WITH_KNOTS('',3,(#107328,#107329,#107330,#107331,#107332,
#107333,#107334,#107335,#107336,#107337,#107338,#107339,#107340,#107341,
#107342,#107343),.UNSPECIFIED.,.F.,.F.,(4,3,3,3,3,4),(-0.046837014256793,
-0.0463994157012118,-0.0407777109438107,-0.0349170905396121,-0.0290580381914533,
-0.0231997078505249),.UNSPECIFIED.) ;
#1617=B_SPLINE_CURVE_WITH_KNOTS('',3,(#107759,#107760,#107761,#107762,#107763,
#107764,#107765,#107766,#107767,#107768,#107769,#107770,#107771,#107772),
 .UNSPECIFIED.,.F.,.F.,(4,2,2,2,2,2,4),(-0.0559250143525619,-0.0556883945479474,
-0.0495906032011524,-0.0437546843048812,-0.037288575909754,-0.0322854917724513,
-0.027844197274366),.UNSPECIFIED.) ;
#1618=B_SPLINE_CURVE_WITH_KNOTS('',3,(#107775,#107776,#107777,#107778,#107779,
#107780,#107781,#107782,#107783,#107784,#107785,#107786,#107787,#107788),
 .UNSPECIFIED.,.F.,.F.,(4,2,2,2,2,2,4),(-0.000236619803144863,0.,0.00609779134711087,
0.0119337102436339,0.0183998186386153,0.0234029027758149,0.0278441972738027),
 .UNSPECIFIED.) ;
#1619=B_SPLINE_CURVE_WITH_KNOTS('',3,(#107791,#107792,#107793,#107794,#107795,
#107796,#107797,#107798,#107799,#107800,#107801,#107802,#107803,#107804,
#107805,#107806),.UNSPECIFIED.,.F.,.F.,(4,3,3,3,3,4),(-0.000437598556136612,
0.,0.00562170475739987,0.0114823251615695,0.0173413775096577,0.0231997078505359),
 .UNSPECIFIED.) ;
#1620=B_SPLINE_CURVE_WITH_KNOTS('',3,(#107811,#107812,#107813,#107814,#107815,
#107816,#107817,#107818,#107819,#107820,#107821,#107822,#107823,#107824,
#107825,#107826),.UNSPECIFIED.,.F.,.F.,(4,3,3,3,3,4),(0.,0.00585824217054478,
0.0117172063374487,0.0175777385368331,0.0231993586852603,0.0236369506553383),
 .UNSPECIFIED.) ;
#1621=B_SPLINE_CURVE_WITH_KNOTS('',3,(#107828,#107829,#107830,#107831,#107832,
#107833,#107834,#107835,#107836,#107837,#107838,#107839,#107840,#107841),
 .UNSPECIFIED.,.F.,.F.,(4,2,2,2,2,2,4),(-0.000236619803563006,0.,0.00609779134689459,
0.0119337102432047,0.0183998186381472,0.0234029027752928,0.027844197273235),
 .UNSPECIFIED.) ;
#1622=B_SPLINE_CURVE_WITH_KNOTS('',3,(#107844,#107845,#107846,#107847,#107848,
#107849,#107850,#107851,#107852,#107853,#107854,#107855,#107856,#107857,
#107858,#107859),.UNSPECIFIED.,.F.,.F.,(4,3,3,3,3,4),(0.,0.00585824217054169,
0.0117172063374197,0.0175777385367584,0.0231993586851914,0.0236369506552836),
 .UNSPECIFIED.) ;
#1623=B_SPLINE_CURVE_WITH_KNOTS('',3,(#107861,#107862,#107863,#107864,#107865,
#107866,#107867,#107868,#107869,#107870,#107871,#107872,#107873,#107874),
 .UNSPECIFIED.,.F.,.F.,(4,2,2,2,2,2,4),(-0.055925014352618,-0.0556883945495578,
-0.049590603202043,-0.0437546843051378,-0.0372885759097438,-0.032285491772261,
-0.0278441972740487),.UNSPECIFIED.) ;
#1624=B_SPLINE_CURVE_WITH_KNOTS('',3,(#107876,#107877,#107878,#107879,#107880,
#107881,#107882,#107883,#107884,#107885,#107886,#107887,#107888,#107889,
#107890,#107891),.UNSPECIFIED.,.F.,.F.,(4,3,3,3,3,4),(-0.000437598556173687,
0.,0.00562170475743059,0.0114823251616519,0.0173413775098334,0.0231997078507748),
 .UNSPECIFIED.) ;
#1625=B_SPLINE_CURVE_WITH_KNOTS('',3,(#107896,#107897,#107898,#107899,#107900,
#107901,#107902,#107903,#107904,#107905,#107906,#107907,#107908,#107909,
#107910,#107911),.UNSPECIFIED.,.F.,.F.,(4,3,3,3,3,4),(0.,0.0058582421705496,
0.0117172063374621,0.01757773853685,0.0231993586852295,0.0236369506553315),
 .UNSPECIFIED.) ;
#1626=B_SPLINE_CURVE_WITH_KNOTS('',3,(#107912,#107913,#107914,#107915,#107916,
#107917,#107918,#107919,#107920,#107921,#107922,#107923,#107924,#107925),
 .UNSPECIFIED.,.F.,.F.,(4,2,2,2,2,2,4),(-0.000236619803562956,0.,0.00609779134697842,
0.0119337102433575,0.0183998186383507,0.0234029027755715,0.027844197273593),
 .UNSPECIFIED.) ;
#1627=B_SPLINE_CURVE_WITH_KNOTS('',3,(#107927,#107928,#107929,#107930,#107931,
#107932,#107933,#107934,#107935,#107936,#107937,#107938,#107939,#107940),
 .UNSPECIFIED.,.F.,.F.,(4,2,2,2,2,2,4),(-0.00023661980356627,0.,0.0060977913470113,
0.0119337102434447,0.0183998186385308,0.0234029027758003,0.027844197273845),
 .UNSPECIFIED.) ;
#1628=B_SPLINE_CURVE_WITH_KNOTS('',3,(#107941,#107942,#107943,#107944,#107945,
#107946,#107947,#107948,#107949,#107950,#107951,#107952,#107953,#107954,
#107955,#107956),.UNSPECIFIED.,.F.,.F.,(4,3,3,3,3,4),(0.,0.00585824217053873,
0.0117172063374278,0.0175777385368055,0.023199358685178,0.0236369506552736),
 .UNSPECIFIED.) ;
#1629=B_SPLINE_CURVE_WITH_KNOTS('',3,(#107958,#107959,#107960,#107961,#107962,
#107963,#107964,#107965,#107966,#107967,#107968,#107969,#107970,#107971),
 .UNSPECIFIED.,.F.,.F.,(4,2,2,2,2,2,4),(-0.055925014347253,-0.0556883945436994,
-0.0495906031970911,-0.0437546843011451,-0.0372885759065727,-0.0322854917697116,
-0.0278441972720297),.UNSPECIFIED.) ;
#1630=B_SPLINE_CURVE_WITH_KNOTS('',3,(#107973,#107974,#107975,#107976,#107977,
#107978,#107979,#107980,#107981,#107982,#107983,#107984,#107985,#107986,
#107987,#107988),.UNSPECIFIED.,.F.,.F.,(4,3,3,3,3,4),(-0.000437598556065294,
0.,0.00562170475696129,0.0114823251605729,0.0173413775081186,0.0231997078484631),
 .UNSPECIFIED.) ;
#1631=B_SPLINE_CURVE_WITH_KNOTS('',3,(#107993,#107994,#107995,#107996,#107997,
#107998,#107999,#108000,#108001,#108002,#108003,#108004,#108005,#108006,
#108007,#108008),.UNSPECIFIED.,.F.,.F.,(4,3,3,3,3,4),(0.,0.00585824217053423,
0.0117172063374038,0.0175777385367393,0.0231993586850723,0.0236369506551701),
 .UNSPECIFIED.) ;
#1632=B_SPLINE_CURVE_WITH_KNOTS('',3,(#108009,#108010,#108011,#108012,#108013,
#108014,#108015,#108016,#108017,#108018,#108019,#108020,#108021,#108022),
 .UNSPECIFIED.,.F.,.F.,(4,2,2,2,2,2,4),(-0.00023661980315042,0.,0.00609779134723154,
0.0119337102438925,0.0183998186390206,0.0234029027763186,0.027844197274388),
 .UNSPECIFIED.) ;
#1633=B_SPLINE_CURVE_WITH_KNOTS('',3,(#108024,#108025,#108026,#108027,#108028,
#108029,#108030,#108031,#108032,#108033,#108034,#108035,#108036,#108037),
 .UNSPECIFIED.,.F.,.F.,(4,2,2,2,2,2,4),(-0.000236619803568179,0.,0.00609779134706943,
0.011933710243561,0.0183998186387449,0.0234029027760718,0.0278441972741583),
 .UNSPECIFIED.) ;
#1634=B_SPLINE_CURVE_WITH_KNOTS('',3,(#108038,#108039,#108040,#108041,#108042,
#108043,#108044,#108045,#108046,#108047,#108048,#108049,#108050,#108051,
#108052,#108053),.UNSPECIFIED.,.F.,.F.,(4,3,3,3,3,4),(0.,0.00585824217054849,
0.0117172063374606,0.0175777385368388,0.0231993586852149,0.0236369506553345),
 .UNSPECIFIED.) ;
#1635=B_SPLINE_CURVE_WITH_KNOTS('',3,(#108055,#108056,#108057,#108058,#108059,
#108060,#108061,#108062,#108063,#108064,#108065,#108066,#108067,#108068),
 .UNSPECIFIED.,.F.,.F.,(4,2,2,2,2,2,4),(-0.0559250143497057,-0.0556883945461452,
-0.0495906031993172,-0.0437546843030612,-0.0372885759081806,-0.0322854917710824,
-0.0278441972731839),.UNSPECIFIED.) ;
#1636=B_SPLINE_CURVE_WITH_KNOTS('',3,(#108070,#108071,#108072,#108073,#108074,
#108075,#108076,#108077,#108078,#108079,#108080,#108081,#108082,#108083,
#108084,#108085),.UNSPECIFIED.,.F.,.F.,(4,3,3,3,3,4),(-0.000437598556084839,
0.,0.00562170475699754,0.0114823251606981,0.0173413775083502,0.0231997078487964),
 .UNSPECIFIED.) ;
#1637=B_SPLINE_CURVE_WITH_KNOTS('',3,(#108090,#108091,#108092,#108093,#108094,
#108095,#108096,#108097,#108098,#108099,#108100,#108101,#108102,#108103,
#108104,#108105),.UNSPECIFIED.,.F.,.F.,(4,3,3,3,3,4),(0.,0.00585824217054277,
0.0117172063374441,0.0175777385368182,0.0231993586851572,0.0236369506552668),
 .UNSPECIFIED.) ;
#1638=B_SPLINE_CURVE_WITH_KNOTS('',3,(#108106,#108107,#108108,#108109,#108110,
#108111,#108112,#108113,#108114,#108115,#108116,#108117,#108118,#108119),
 .UNSPECIFIED.,.F.,.F.,(4,2,2,2,2,2,4),(-0.00023661980356187,0.,0.00609779134698056,
0.0119337102433812,0.0183998186384326,0.0234029027756759,0.0278441972736905),
 .UNSPECIFIED.) ;
#1639=B_SPLINE_CURVE_WITH_KNOTS('',3,(#108121,#108122,#108123,#108124,#108125,
#108126,#108127,#108128,#108129,#108130,#108131,#108132,#108133,#108134),
 .UNSPECIFIED.,.F.,.F.,(4,2,2,2,2,2,4),(-0.000236619803566785,0.,0.00609779134702904,
0.0119337102434475,0.0183998186384865,0.0234029027757207,0.0278441972737459),
 .UNSPECIFIED.) ;
#1640=B_SPLINE_CURVE_WITH_KNOTS('',3,(#108135,#108136,#108137,#108138,#108139,
#108140,#108141,#108142,#108143,#108144,#108145,#108146,#108147,#108148,
#108149,#108150),.UNSPECIFIED.,.F.,.F.,(4,3,3,3,3,4),(0.,0.00585824217054034,
0.0117172063374279,0.0175777385367946,0.0231993586851777,0.0236369506552812),
 .UNSPECIFIED.) ;
#1641=B_SPLINE_CURVE_WITH_KNOTS('',3,(#108152,#108153,#108154,#108155,#108156,
#108157,#108158,#108159,#108160,#108161,#108162,#108163,#108164,#108165),
 .UNSPECIFIED.,.F.,.F.,(4,2,2,2,2,2,4),(-0.0559250143501053,-0.0556883945465432,
-0.0495906031996281,-0.0437546843033128,-0.0372885759083777,-0.0322854917712189,
-0.0278441972732712),.UNSPECIFIED.) ;
#1642=B_SPLINE_CURVE_WITH_KNOTS('',3,(#108167,#108168,#108169,#108170,#108171,
#108172,#108173,#108174,#108175,#108176,#108177,#108178,#108179,#108180,
#108181,#108182),.UNSPECIFIED.,.F.,.F.,(4,3,3,3,3,4),(-0.000437598556096447,
0.,0.00562170475713416,0.0114823251609764,0.0173413775087778,0.0231997078493597),
 .UNSPECIFIED.) ;
#1643=B_SPLINE_CURVE_WITH_KNOTS('',3,(#108187,#108188,#108189,#108190,#108191,
#108192,#108193,#108194,#108195,#108196,#108197,#108198,#108199,#108200,
#108201,#108202),.UNSPECIFIED.,.F.,.F.,(4,3,3,3,3,4),(0.,0.00585824217053087,
0.0117172063373846,0.0175777385366825,0.0231993586850888,0.0236369506551764),
 .UNSPECIFIED.) ;
#1644=B_SPLINE_CURVE_WITH_KNOTS('',3,(#108203,#108204,#108205,#108206,#108207,
#108208,#108209,#108210,#108211,#108212,#108213,#108214,#108215,#108216),
 .UNSPECIFIED.,.F.,.F.,(4,2,2,2,2,2,4),(-0.000236619803975554,0.,0.00609779134645292,
0.0119337102422305,0.0183998186368445,0.0234029027737468,0.0278441972714777),
 .UNSPECIFIED.) ;
#1645=B_SPLINE_CURVE_WITH_KNOTS('',3,(#108218,#108219,#108220,#108221,#108222,
#108223,#108224,#108225,#108226,#108227,#108228,#108229,#108230,#108231),
 .UNSPECIFIED.,.F.,.F.,(4,2,2,2,2,2,4),(-0.000236619803145561,0.,0.00609779134719067,
0.0119337102437602,0.0183998186387406,0.0234029027759312,0.0278441972739105),
 .UNSPECIFIED.) ;
#1646=B_SPLINE_CURVE_WITH_KNOTS('',3,(#108232,#108233,#108234,#108235,#108236,
#108237,#108238,#108239,#108240,#108241,#108242,#108243,#108244,#108245,
#108246,#108247),.UNSPECIFIED.,.F.,.F.,(4,3,3,3,3,4),(0.,0.00585824217053935,
0.0117172063374137,0.0175777385367471,0.0231993586851797,0.0236369506552624),
 .UNSPECIFIED.) ;
#1647=B_SPLINE_CURVE_WITH_KNOTS('',3,(#108249,#108250,#108251,#108252,#108253,
#108254,#108255,#108256,#108257,#108258,#108259,#108260,#108261,#108262),
 .UNSPECIFIED.,.F.,.F.,(4,2,2,2,2,2,4),(-0.0559250143516561,-0.0556883945480848,
-0.0495906032009887,-0.0437546843044866,-0.0372885759093485,-0.032285491772039,
-0.0278441972739555),.UNSPECIFIED.) ;
#1648=B_SPLINE_CURVE_WITH_KNOTS('',3,(#108264,#108265,#108266,#108267,#108268,
#108269,#108270,#108271,#108272,#108273,#108274,#108275,#108276,#108277,
#108278,#108279),.UNSPECIFIED.,.F.,.F.,(4,3,3,3,3,4),(-0.000437598556137922,
0.,0.00562170475738925,0.0114823251615342,0.0173413775096173,0.0231997078504894),
 .UNSPECIFIED.) ;
#1649=B_SPLINE_CURVE_WITH_KNOTS('',3,(#108284,#108285,#108286,#108287,#108288,
#108289,#108290,#108291,#108292,#108293,#108294,#108295,#108296,#108297,
#108298,#108299),.UNSPECIFIED.,.F.,.F.,(4,3,3,3,3,4),(0.,0.00585824217054286,
0.0117172063374258,0.0175777385367681,0.0231993586851975,0.0236369506552776),
 .UNSPECIFIED.) ;
#1650=B_SPLINE_CURVE_WITH_KNOTS('',3,(#108300,#108301,#108302,#108303,#108304,
#108305,#108306,#108307,#108308,#108309,#108310,#108311,#108312,#108313),
 .UNSPECIFIED.,.F.,.F.,(4,2,2,2,2,2,4),(-0.000236619803141347,0.,0.00609779134719742,
0.0119337102437761,0.0183998186387667,0.0234029027759622,0.0278441972739489),
 .UNSPECIFIED.) ;
#1651=B_SPLINE_CURVE_WITH_KNOTS('',3,(#108315,#108316,#108317,#108318,#108319,
#108320,#108321,#108322,#108323,#108324,#108325,#108326,#108327,#108328),
 .UNSPECIFIED.,.F.,.F.,(4,2,2,2,2,2,4),(-0.000236619803560324,0.,0.00609779134688203,
0.0119337102431469,0.0183998186380461,0.0234029027751694,0.0278441972730812),
 .UNSPECIFIED.) ;
#1652=B_SPLINE_CURVE_WITH_KNOTS('',3,(#108329,#108330,#108331,#108332,#108333,
#108334,#108335,#108336,#108337,#108338,#108339,#108340,#108341,#108342,
#108343,#108344),.UNSPECIFIED.,.F.,.F.,(4,3,3,3,3,4),(0.,0.00585824217053624,
0.0117172063373978,0.017577738536714,0.0231993586851339,0.0236369506552253),
 .UNSPECIFIED.) ;
#1653=B_SPLINE_CURVE_WITH_KNOTS('',3,(#108346,#108347,#108348,#108349,#108350,
#108351,#108352,#108353,#108354,#108355,#108356,#108357,#108358,#108359),
 .UNSPECIFIED.,.F.,.F.,(4,2,2,2,2,2,4),(-0.0559250143527569,-0.0556883945491825,
-0.0495906032019952,-0.0437546843053732,-0.0372885759100185,-0.0322854917725816,
-0.0278441972744026),.UNSPECIFIED.) ;
#1654=B_SPLINE_CURVE_WITH_KNOTS('',3,(#108361,#108362,#108363,#108364,#108365,
#108366,#108367,#108368,#108369,#108370,#108371,#108372,#108373,#108374,
#108375,#108376),.UNSPECIFIED.,.F.,.F.,(4,3,3,3,3,4),(-0.000437598556170072,
0.,0.00562170475739005,0.0114823251615356,0.0173413775096278,0.0231997078504878),
 .UNSPECIFIED.) ;
#1655=B_SPLINE_CURVE_WITH_KNOTS('',3,(#108381,#108382,#108383,#108384,#108385,
#108386,#108387,#108388,#108389,#108390,#108391,#108392,#108393,#108394,
#108395,#108396),.UNSPECIFIED.,.F.,.F.,(4,3,3,3,3,4),(0.,0.00585824217054469,
0.0117172063374513,0.0175777385368039,0.0231993586851361,0.0236369506553527),
 .UNSPECIFIED.) ;
#1656=B_SPLINE_CURVE_WITH_KNOTS('',3,(#108397,#108398,#108399,#108400,#108401,
#108402,#108403,#108404,#108405,#108406,#108407,#108408,#108409,#108410),
 .UNSPECIFIED.,.F.,.F.,(4,2,2,2,2,2,4),(-0.000236619804202799,0.,0.00609779134737763,
0.0119337102442503,0.0183998186398358,0.0234029027774637,0.0278441972757869),
 .UNSPECIFIED.) ;
#1657=B_SPLINE_CURVE_WITH_KNOTS('',3,(#108412,#108413,#108414,#108415,#108416,
#108417,#108418,#108419,#108420,#108421,#108422,#108423,#108424,#108425),
 .UNSPECIFIED.,.F.,.F.,(4,2,2,2,2,2,4),(-0.0002366198042002,0.,0.00609779134724177,
0.0119337102439773,0.0183998186394422,0.0234029027769713,0.027844197275244),
 .UNSPECIFIED.) ;
#1658=B_SPLINE_CURVE_WITH_KNOTS('',3,(#108426,#108427,#108428,#108429,#108430,
#108431,#108432,#108433,#108434,#108435,#108436,#108437,#108438,#108439,
#108440,#108441),.UNSPECIFIED.,.F.,.F.,(4,3,3,3,3,4),(0.,0.00585824217054219,
0.0117172063374448,0.0175777385367976,0.0231993586850719,0.0236369506552122),
 .UNSPECIFIED.) ;
#1659=B_SPLINE_CURVE_WITH_KNOTS('',3,(#108443,#108444,#108445,#108446,#108447,
#108448,#108449,#108450,#108451,#108452,#108453,#108454,#108455,#108456),
 .UNSPECIFIED.,.F.,.F.,(4,2,2,2,2,2,4),(-0.0559250143475747,-0.0556883945440193,
-0.0495906031973805,-0.0437546843014019,-0.0372885759067931,-0.0322854917699036,
-0.0278441972721905),.UNSPECIFIED.) ;
#1660=B_SPLINE_CURVE_WITH_KNOTS('',3,(#108458,#108459,#108460,#108461,#108462,
#108463,#108464,#108465,#108466,#108467,#108468,#108469,#108470,#108471,
#108472,#108473),.UNSPECIFIED.,.F.,.F.,(4,3,3,3,3,4),(-0.000437598556074084,
0.,0.00562170475694653,0.0114823251605845,0.0173413775081531,0.0231997078485162),
 .UNSPECIFIED.) ;
#1661=B_SPLINE_CURVE_WITH_KNOTS('',3,(#108478,#108479,#108480,#108481,#108482,
#108483,#108484,#108485,#108486,#108487,#108488,#108489,#108490,#108491,
#108492,#108493),.UNSPECIFIED.,.F.,.F.,(4,3,3,3,3,4),(0.,0.00585824217053932,
0.0117172063374163,0.0175777385367554,0.0231993586851953,0.0236369506552652),
 .UNSPECIFIED.) ;
#1662=B_SPLINE_CURVE_WITH_KNOTS('',3,(#108494,#108495,#108496,#108497,#108498,
#108499,#108500,#108501,#108502,#108503,#108504,#108505,#108506,#108507),
 .UNSPECIFIED.,.F.,.F.,(4,2,2,2,2,2,4),(-0.000236619803563584,0.,0.00609779134684538,
0.0119337102430664,0.0183998186379667,0.0234029027750871,0.0278441972729952),
 .UNSPECIFIED.) ;
#1663=B_SPLINE_CURVE_WITH_KNOTS('',3,(#108509,#108510,#108511,#108512,#108513,
#108514,#108515,#108516,#108517,#108518,#108519,#108520,#108521,#108522),
 .UNSPECIFIED.,.F.,.F.,(4,2,2,2,2,2,4),(-0.000236619803559064,0.,0.00609779134682761,
0.0119337102430243,0.0183998186378634,0.0234029027749327,0.0278441972727837),
 .UNSPECIFIED.) ;
#1664=B_SPLINE_CURVE_WITH_KNOTS('',3,(#108523,#108524,#108525,#108526,#108527,
#108528,#108529,#108530,#108531,#108532,#108533,#108534,#108535,#108536,
#108537,#108538),.UNSPECIFIED.,.F.,.F.,(4,3,3,3,3,4),(0.,0.00585824217053403,
0.0117172063373908,0.0175777385367026,0.0231993586851274,0.0236369506551984),
 .UNSPECIFIED.) ;
#1665=B_SPLINE_CURVE_WITH_KNOTS('',3,(#108540,#108541,#108542,#108543,#108544,
#108545,#108546,#108547,#108548,#108549,#108550,#108551,#108552,#108553),
 .UNSPECIFIED.,.F.,.F.,(4,2,2,2,2,2,4),(-0.0559250143495183,-0.0556883945459582,
-0.0495906031991357,-0.0437546843029003,-0.0372885759080418,-0.0322854917709563,
-0.0278441972730646),.UNSPECIFIED.) ;
#1666=B_SPLINE_CURVE_WITH_KNOTS('',3,(#108555,#108556,#108557,#108558,#108559,
#108560,#108561,#108562,#108563,#108564,#108565,#108566,#108567,#108568,
#108569,#108570),.UNSPECIFIED.,.F.,.F.,(4,3,3,3,3,4),(-0.000437598556092783,
0.,0.00562170475708721,0.0114823251608936,0.0173413775086511,0.0231997078492032),
 .UNSPECIFIED.) ;
#1667=B_SPLINE_CURVE_WITH_KNOTS('',3,(#108575,#108576,#108577,#108578,#108579,
#108580,#108581,#108582,#108583,#108584,#108585,#108586,#108587,#108588,
#108589,#108590),.UNSPECIFIED.,.F.,.F.,(4,3,3,3,3,4),(0.,0.00585824217054838,
0.0117172063374519,0.0175777385368119,0.0231993586852536,0.0236369506553148),
 .UNSPECIFIED.) ;
#1668=B_SPLINE_CURVE_WITH_KNOTS('',3,(#108591,#108592,#108593,#108594,#108595,
#108596,#108597,#108598,#108599,#108600,#108601,#108602,#108603,#108604),
 .UNSPECIFIED.,.F.,.F.,(4,2,2,2,2,2,4),(-0.000236619803558096,0.,0.00609779134681664,
0.0119337102430081,0.0183998186378316,0.0234029027748886,0.0278441972727373),
 .UNSPECIFIED.) ;
#1669=B_SPLINE_CURVE_WITH_KNOTS('',3,(#108606,#108607,#108608,#108609,#108610,
#108611,#108612,#108613,#108614,#108615,#108616,#108617,#108618,#108619),
 .UNSPECIFIED.,.F.,.F.,(4,2,2,2,2,2,4),(-0.000236619803562333,0.,0.00609779134692135,
0.0119337102432951,0.0183998186383094,0.0234029027755172,0.0278441972735094),
 .UNSPECIFIED.) ;
#1670=B_SPLINE_CURVE_WITH_KNOTS('',3,(#108620,#108621,#108622,#108623,#108624,
#108625,#108626,#108627,#108628,#108629,#108630,#108631,#108632,#108633,
#108634,#108635),.UNSPECIFIED.,.F.,.F.,(4,3,3,3,3,4),(0.,0.00585824217054129,
0.0117172063374373,0.0175777385368199,0.023199358685217,0.0236369506553186),
 .UNSPECIFIED.) ;
#1671=B_SPLINE_CURVE_WITH_KNOTS('',3,(#108637,#108638,#108639,#108640,#108641,
#108642,#108643,#108644,#108645,#108646,#108647,#108648,#108649,#108650),
 .UNSPECIFIED.,.F.,.F.,(4,2,2,2,2,2,4),(-0.0559250143502032,-0.0556883945466394,
-0.0495906031997328,-0.0437546843034414,-0.0372885759084786,-0.0322854917713055,
-0.0278441972733409),.UNSPECIFIED.) ;
#1672=B_SPLINE_CURVE_WITH_KNOTS('',3,(#108652,#108653,#108654,#108655,#108656,
#108657,#108658,#108659,#108660,#108661,#108662,#108663,#108664,#108665,
#108666,#108667),.UNSPECIFIED.,.F.,.F.,(4,3,3,3,3,4),(-0.000437598556094846,
0.,0.00562170475708876,0.0114823251608924,0.0173413775086073,0.0231997078491061),
 .UNSPECIFIED.) ;
#1673=B_SPLINE_CURVE_WITH_KNOTS('',3,(#108669,#108670,#108671,#108672,#108673,
#108674,#108675,#108676,#108677,#108678,#108679,#108680,#108681,#108682,
#108683,#108684),.UNSPECIFIED.,.F.,.F.,(4,3,3,3,3,4),(0.,0.00585824217053639,
0.0117172063374152,0.0175777385367772,0.0231993586851953,0.0236369506552933),
 .UNSPECIFIED.) ;
#1674=B_SPLINE_CURVE_WITH_KNOTS('',3,(#108685,#108686,#108687,#108688,#108689,
#108690,#108691,#108692,#108693,#108694,#108695,#108696,#108697,#108698),
 .UNSPECIFIED.,.F.,.F.,(4,2,2,2,2,2,4),(-0.000236619803922217,0.,0.00609779134654128,
0.0119337102425373,0.018399818637407,0.0234029027744858,0.0278441972723643),
 .UNSPECIFIED.) ;
#1675=B_SPLINE_CURVE_WITH_KNOTS('',3,(#108700,#108701,#108702,#108703,#108704,
#108705,#108706,#108707,#108708,#108709,#108710,#108711,#108712,#108713),
 .UNSPECIFIED.,.F.,.F.,(4,2,2,2,2,2,4),(-0.000236619803561269,0.,0.00609779134692068,
0.0119337102432194,0.0183998186381382,0.02340290277528,0.0278441972732167),
 .UNSPECIFIED.) ;
#1676=B_SPLINE_CURVE_WITH_KNOTS('',3,(#108714,#108715,#108716,#108717,#108718,
#108719,#108720,#108721,#108722,#108723,#108724,#108725,#108726,#108727,
#108728,#108729),.UNSPECIFIED.,.F.,.F.,(4,3,3,3,3,4),(0.,0.00585824217053491,
0.0117172063374156,0.0175777385367886,0.0231993586852222,0.0236369506553088),
 .UNSPECIFIED.) ;
#1677=B_SPLINE_CURVE_WITH_KNOTS('',3,(#108731,#108732,#108733,#108734,#108735,
#108736,#108737,#108738,#108739,#108740,#108741,#108742,#108743,#108744),
 .UNSPECIFIED.,.F.,.F.,(4,2,2,2,2,2,4),(-0.0559250143500672,-0.0556883945469228,
-0.049590603199785,-0.0437546843032336,-0.0372885759082228,-0.0322854917710044,
-0.0278441972729959),.UNSPECIFIED.) ;
#1678=B_SPLINE_CURVE_WITH_KNOTS('',3,(#108746,#108747,#108748,#108749,#108750,
#108751,#108752,#108753,#108754,#108755,#108756,#108757,#108758,#108759,
#108760,#108761),.UNSPECIFIED.,.F.,.F.,(4,3,3,3,3,4),(-0.000437598556138437,
0.,0.00562170475741228,0.0114823251616098,0.0173413775097521,0.0231997078506926),
 .UNSPECIFIED.) ;
#1679=B_SPLINE_CURVE_WITH_KNOTS('',3,(#108767,#108768,#108769,#108770,#108771,
#108772,#108773,#108774,#108775,#108776,#108777,#108778,#108779,#108780),
 .UNSPECIFIED.,.F.,.F.,(4,2,2,2,2,2,4),(-0.0559250143516994,-0.0556883945481287,
-0.0495906032010545,-0.0437546843045533,-0.0372885759093916,-0.0322854917720808,
-0.0278441972739919),.UNSPECIFIED.) ;
#1680=B_SPLINE_CURVE_WITH_KNOTS('',3,(#108784,#108785,#108786,#108787,#108788,
#108789,#108790,#108791,#108792,#108793,#108794,#108795,#108796,#108797,
#108798,#108799),.UNSPECIFIED.,.F.,.F.,(4,3,3,3,3,4),(-0.000437598556144422,
0.,0.00562170475740183,0.0114823251615895,0.0173413775097444,0.0231997078506806),
 .UNSPECIFIED.) ;
#1681=B_SPLINE_CURVE_WITH_KNOTS('',3,(#108806,#108807,#108808,#108809,#108810,
#108811,#108812,#108813,#108814,#108815,#108816,#108817,#108818,#108819),
 .UNSPECIFIED.,.F.,.F.,(4,2,2,2,2,2,4),(-0.0559250143435119,-0.0556883945403911,
-0.0495906031940201,-0.0437546842982849,-0.0372885759042276,-0.0322854917677294,
-0.0278441972703399),.UNSPECIFIED.) ;
#1682=B_SPLINE_CURVE_WITH_KNOTS('',3,(#108823,#108824,#108825,#108826,#108827,
#108828,#108829,#108830,#108831,#108832,#108833,#108834,#108835,#108836,
#108837,#108838),.UNSPECIFIED.,.F.,.F.,(4,3,3,3,3,4),(-0.000437598556018984,
0.,0.00562170475658728,0.0114823251597353,0.0173413775068133,0.0231997078467154),
 .UNSPECIFIED.) ;
#1683=B_SPLINE_CURVE_WITH_KNOTS('',3,(#108845,#108846,#108847,#108848,#108849,
#108850,#108851,#108852,#108853,#108854,#108855,#108856,#108857,#108858),
 .UNSPECIFIED.,.F.,.F.,(4,2,2,2,2,2,4),(-0.0559250143454541,-0.055688394541913,
-0.0495906031955341,-0.0437546842998321,-0.0372885759055476,-0.0322854917689083,
-0.0278441972713927),.UNSPECIFIED.) ;
#1684=B_SPLINE_CURVE_WITH_KNOTS('',3,(#108862,#108863,#108864,#108865,#108866,
#108867,#108868,#108869,#108870,#108871,#108872,#108873,#108874,#108875,
#108876,#108877),.UNSPECIFIED.,.F.,.F.,(4,3,3,3,3,4),(-0.000437598556040506,
0.,0.00562170475667276,0.0114823251599514,0.0173413775071961,0.0231997078472458),
 .UNSPECIFIED.) ;
#1685=B_SPLINE_CURVE_WITH_KNOTS('',3,(#108884,#108885,#108886,#108887,#108888,
#108889,#108890,#108891,#108892,#108893,#108894,#108895,#108896,#108897),
 .UNSPECIFIED.,.F.,.F.,(4,2,2,2,2,2,4),(-0.0559250143503411,-0.0556883945467744,
-0.0495906031998412,-0.0437546843035047,-0.0372885759085466,-0.0322854917713593,
-0.0278441972733858),.UNSPECIFIED.) ;
#1686=B_SPLINE_CURVE_WITH_KNOTS('',3,(#108901,#108902,#108903,#108904,#108905,
#108906,#108907,#108908,#108909,#108910,#108911,#108912,#108913,#108914,
#108915,#108916),.UNSPECIFIED.,.F.,.F.,(4,3,3,3,3,4),(-0.00043759855609295,
0.,0.00562170475705494,0.0114823251608269,0.0173413775085459,0.0231997078490585),
 .UNSPECIFIED.) ;
#1687=B_SPLINE_CURVE_WITH_KNOTS('',3,(#108923,#108924,#108925,#108926,#108927,
#108928,#108929,#108930,#108931,#108932,#108933,#108934,#108935,#108936),
 .UNSPECIFIED.,.F.,.F.,(4,2,2,2,2,2,4),(-0.0559250143576788,-0.0556883945534629,
-0.0495906032058708,-0.0437546843087237,-0.0372885759128067,-0.0322854917749087,
-0.027844197276348),.UNSPECIFIED.) ;
#1688=B_SPLINE_CURVE_WITH_KNOTS('',3,(#108940,#108941,#108942,#108943,#108944,
#108945,#108946,#108947,#108948,#108949,#108950,#108951,#108952,#108953,
#108954,#108955),.UNSPECIFIED.,.F.,.F.,(4,3,3,3,3,4),(-0.000437598556265556,
0.,0.00562170475766576,0.0114823251621366,0.0173413775105401,0.0231997078516975),
 .UNSPECIFIED.) ;
#1689=B_SPLINE_CURVE_WITH_KNOTS('',3,(#108962,#108963,#108964,#108965,#108966,
#108967,#108968,#108969,#108970,#108971,#108972,#108973,#108974,#108975),
 .UNSPECIFIED.,.F.,.F.,(4,2,2,2,2,2,4),(-0.0559250143546525,-0.0556883945504525,
-0.0495906032031384,-0.0437546843063546,-0.0372885759108327,-0.0322854917732639,
-0.0278441972749651),.UNSPECIFIED.) ;
#1690=B_SPLINE_CURVE_WITH_KNOTS('',3,(#108979,#108980,#108981,#108982,#108983,
#108984,#108985,#108986,#108987,#108988,#108989,#108990,#108991,#108992,
#108993,#108994),.UNSPECIFIED.,.F.,.F.,(4,3,3,3,3,4),(-0.000437598556211791,
0.,0.00562170475765983,0.011482325162167,0.0173413775106296,0.0231997078518591),
 .UNSPECIFIED.) ;
#1691=B_SPLINE_CURVE_WITH_KNOTS('',3,(#109001,#109002,#109003,#109004,#109005,
#109006,#109007,#109008,#109009,#109010,#109011,#109012,#109013,#109014),
 .UNSPECIFIED.,.F.,.F.,(4,2,2,2,2,2,4),(-0.0559250143563362,-0.055688394551709,
-0.0495906032045639,-0.0437546843078355,-0.0372885759121675,-0.0322854917744538,
-0.0278441972760254),.UNSPECIFIED.) ;
#1692=B_SPLINE_CURVE_WITH_KNOTS('',3,(#109018,#109019,#109020,#109021,#109022,
#109023,#109024,#109025,#109026,#109027,#109028,#109029,#109030,#109031,
#109032,#109033),.UNSPECIFIED.,.F.,.F.,(4,3,3,3,3,4),(-0.000437598556225459,
0.,0.00562170475744369,0.0114823251616755,0.0173413775098568,0.0231997078508077),
 .UNSPECIFIED.) ;
#1693=B_SPLINE_CURVE_WITH_KNOTS('',3,(#109040,#109041,#109042,#109043,#109044,
#109045,#109046,#109047,#109048,#109049,#109050,#109051,#109052,#109053),
 .UNSPECIFIED.,.F.,.F.,(4,2,2,2,2,2,4),(-0.0559250143492567,-0.0556883945456972,
-0.0495906031988905,-0.0437546843027083,-0.0372885759078583,-0.0322854917707879,
-0.0278441972729168),.UNSPECIFIED.) ;
#1694=B_SPLINE_CURVE_WITH_KNOTS('',3,(#109057,#109058,#109059,#109060,#109061,
#109062,#109063,#109064,#109065,#109066,#109067,#109068,#109069,#109070,
#109071,#109072),.UNSPECIFIED.,.F.,.F.,(4,3,3,3,3,4),(-0.000437598556080345,
0.,0.00562170475697672,0.0114823251606002,0.0173413775081636,0.0231997078485257),
 .UNSPECIFIED.) ;
#1695=B_SPLINE_CURVE_WITH_KNOTS('',3,(#109079,#109080,#109081,#109082,#109083,
#109084,#109085,#109086,#109087,#109088,#109089,#109090,#109091,#109092),
 .UNSPECIFIED.,.F.,.F.,(4,2,2,2,2,2,4),(-0.055925014349952,-0.0556883945463912,
-0.0495906031994983,-0.0437546843032064,-0.0372885759082967,-0.0322854917711481,
-0.0278441972731949),.UNSPECIFIED.) ;
#1696=B_SPLINE_CURVE_WITH_KNOTS('',3,(#109096,#109097,#109098,#109099,#109100,
#109101,#109102,#109103,#109104,#109105,#109106,#109107,#109108,#109109,
#109110,#109111),.UNSPECIFIED.,.F.,.F.,(4,3,3,3,3,4),(-0.000437598556096392,
0.,0.005621704757061,0.0114823251608164,0.0173413775085336,0.0231997078490336),
 .UNSPECIFIED.) ;
#2113=B_SPLINE_SURFACE_WITH_KNOTS('',3,3,((#105521,#105522,#105523,#105524,
#105525,#105526,#105527,#105528,#105529,#105530,#105531,#105532,#105533,
#105534,#105535,#105536,#105537),(#105538,#105539,#105540,#105541,#105542,
#105543,#105544,#105545,#105546,#105547,#105548,#105549,#105550,#105551,
#105552,#105553,#105554),(#105555,#105556,#105557,#105558,#105559,#105560,
#105561,#105562,#105563,#105564,#105565,#105566,#105567,#105568,#105569,
#105570,#105571),(#105572,#105573,#105574,#105575,#105576,#105577,#105578,
#105579,#105580,#105581,#105582,#105583,#105584,#105585,#105586,#105587,
#105588),(#105589,#105590,#105591,#105592,#105593,#105594,#105595,#105596,
#105597,#105598,#105599,#105600,#105601,#105602,#105603,#105604,#105605)),
 .UNSPECIFIED.,.F.,.T.,.F.,(4,1,4),(4,1,1,1,1,1,1,1,1,1,1,1,1,1,4),(0.,
0.5,1.),(-1.37470975898194,-1.17832265055595,-0.981935542129957,-0.785548433703966,
-0.589161325277974,-0.392774216851983,-0.196387108425991,0.,0.196387108425991,
0.392774216851983,0.589161325277974,0.785548433703966,0.981935542129957,
1.17832265055595,1.37470975898194),.UNSPECIFIED.) ;
#2114=B_SPLINE_SURFACE_WITH_KNOTS('',3,3,((#105634,#105635,#105636,#105637,
#105638,#105639,#105640,#105641,#105642,#105643,#105644,#105645,#105646,
#105647,#105648,#105649,#105650),(#105651,#105652,#105653,#105654,#105655,
#105656,#105657,#105658,#105659,#105660,#105661,#105662,#105663,#105664,
#105665,#105666,#105667),(#105668,#105669,#105670,#105671,#105672,#105673,
#105674,#105675,#105676,#105677,#105678,#105679,#105680,#105681,#105682,
#105683,#105684),(#105685,#105686,#105687,#105688,#105689,#105690,#105691,
#105692,#105693,#105694,#105695,#105696,#105697,#105698,#105699,#105700,
#105701),(#105702,#105703,#105704,#105705,#105706,#105707,#105708,#105709,
#105710,#105711,#105712,#105713,#105714,#105715,#105716,#105717,#105718)),
 .UNSPECIFIED.,.F.,.T.,.F.,(4,1,4),(4,1,1,1,1,1,1,1,1,1,1,1,1,1,4),(0.,
0.5,1.),(-1.37470975898194,-1.17832265055595,-0.981935542129957,-0.785548433703966,
-0.589161325277974,-0.392774216851983,-0.196387108425991,0.,0.196387108425991,
0.392774216851983,0.589161325277974,0.785548433703966,0.981935542129957,
1.17832265055595,1.37470975898194),.UNSPECIFIED.) ;
#2942=PLANE('',#54549) ;
#2943=PLANE('',#54554) ;
#2944=PLANE('',#54555) ;
#2945=PLANE('',#54557) ;
#2946=PLANE('',#54719) ;
#2947=PLANE('',#54722) ;
#2948=PLANE('',#54725) ;
#2949=PLANE('',#54728) ;
#2950=PLANE('',#54731) ;
#2951=PLANE('',#54734) ;
#2952=PLANE('',#54737) ;
#2953=PLANE('',#54740) ;
#2954=PLANE('',#54743) ;
#2955=PLANE('',#54746) ;
#2956=PLANE('',#54749) ;
#2957=PLANE('',#54752) ;
#2958=PLANE('',#54755) ;
#2959=PLANE('',#54758) ;
#2960=PLANE('',#54761) ;
#2961=PLANE('',#54764) ;
#2962=PLANE('',#54767) ;
#2963=PLANE('',#54770) ;
#2964=PLANE('',#54773) ;
#2965=PLANE('',#54776) ;
#2966=PLANE('',#54779) ;
#2967=PLANE('',#54781) ;
#2968=PLANE('',#54783) ;
#2969=PLANE('',#54785) ;
#2970=PLANE('',#54787) ;
#2971=PLANE('',#54789) ;
#2972=PLANE('',#54791) ;
#2973=PLANE('',#54793) ;
#2974=PLANE('',#54795) ;
#2975=PLANE('',#54797) ;
#2976=PLANE('',#54799) ;
#2977=PLANE('',#54801) ;
#2978=PLANE('',#54803) ;
#2979=PLANE('',#54805) ;
#2980=PLANE('',#54807) ;
#2981=PLANE('',#54809) ;
#2982=PLANE('',#54811) ;
#2983=PLANE('',#54813) ;
#2984=PLANE('',#54815) ;
#2985=PLANE('',#54821) ;
#2986=PLANE('',#54865) ;
#2987=PLANE('',#54867) ;
#2988=PLANE('',#54869) ;
#2989=PLANE('',#54871) ;
#2990=PLANE('',#54873) ;
#2991=PLANE('',#54875) ;
#2992=PLANE('',#54877) ;
#2993=PLANE('',#54879) ;
#2994=PLANE('',#54881) ;
#2995=PLANE('',#54883) ;
#2996=PLANE('',#54885) ;
#2997=PLANE('',#54887) ;
#2998=PLANE('',#54889) ;
#2999=PLANE('',#54891) ;
#3000=PLANE('',#54893) ;
#3001=PLANE('',#54895) ;
#3002=PLANE('',#54897) ;
#3003=PLANE('',#54899) ;
#3004=PLANE('',#54901) ;
#3005=PLANE('',#54903) ;
#3006=PLANE('',#55006) ;
#3007=PLANE('',#55008) ;
#3008=PLANE('',#55009) ;
#3009=PLANE('',#55010) ;
#3010=PLANE('',#55012) ;
#3011=PLANE('',#55013) ;
#3012=PLANE('',#55015) ;
#3013=PLANE('',#55016) ;
#3014=PLANE('',#55018) ;
#3015=PLANE('',#55019) ;
#3016=PLANE('',#55021) ;
#3017=PLANE('',#55022) ;
#3018=PLANE('',#55024) ;
#3019=PLANE('',#55025) ;
#3020=PLANE('',#55027) ;
#3021=PLANE('',#55028) ;
#3022=PLANE('',#55030) ;
#3023=PLANE('',#55031) ;
#3024=PLANE('',#55033) ;
#3025=PLANE('',#55034) ;
#5995=LINE('',#105784,#9209) ;
#5996=LINE('',#105802,#9210) ;
#5997=LINE('',#105826,#9211) ;
#5998=LINE('',#105842,#9212) ;
#5999=LINE('',#105864,#9213) ;
#6000=LINE('',#105882,#9214) ;
#6001=LINE('',#105906,#9215) ;
#6002=LINE('',#105922,#9216) ;
#6003=LINE('',#105944,#9217) ;
#6004=LINE('',#105962,#9218) ;
#6005=LINE('',#105986,#9219) ;
#6006=LINE('',#106002,#9220) ;
#6007=LINE('',#106024,#9221) ;
#6008=LINE('',#106042,#9222) ;
#6009=LINE('',#106066,#9223) ;
#6010=LINE('',#106082,#9224) ;
#6011=LINE('',#106104,#9225) ;
#6012=LINE('',#106122,#9226) ;
#6013=LINE('',#106146,#9227) ;
#6014=LINE('',#106162,#9228) ;
#6015=LINE('',#106184,#9229) ;
#6016=LINE('',#106202,#9230) ;
#6017=LINE('',#106226,#9231) ;
#6018=LINE('',#106242,#9232) ;
#6019=LINE('',#106264,#9233) ;
#6020=LINE('',#106282,#9234) ;
#6021=LINE('',#106306,#9235) ;
#6022=LINE('',#106322,#9236) ;
#6023=LINE('',#106344,#9237) ;
#6024=LINE('',#106362,#9238) ;
#6025=LINE('',#106386,#9239) ;
#6026=LINE('',#106402,#9240) ;
#6027=LINE('',#106424,#9241) ;
#6028=LINE('',#106442,#9242) ;
#6029=LINE('',#106466,#9243) ;
#6030=LINE('',#106482,#9244) ;
#6031=LINE('',#106504,#9245) ;
#6032=LINE('',#106522,#9246) ;
#6033=LINE('',#106546,#9247) ;
#6034=LINE('',#106562,#9248) ;
#6035=LINE('',#106584,#9249) ;
#6036=LINE('',#106586,#9250) ;
#6037=LINE('',#106626,#9251) ;
#6038=LINE('',#106628,#9252) ;
#6039=LINE('',#106664,#9253) ;
#6040=LINE('',#106666,#9254) ;
#6041=LINE('',#106706,#9255) ;
#6042=LINE('',#106708,#9256) ;
#6043=LINE('',#106744,#9257) ;
#6044=LINE('',#106746,#9258) ;
#6045=LINE('',#106786,#9259) ;
#6046=LINE('',#106788,#9260) ;
#6047=LINE('',#106824,#9261) ;
#6048=LINE('',#106826,#9262) ;
#6049=LINE('',#106866,#9263) ;
#6050=LINE('',#106868,#9264) ;
#6051=LINE('',#106904,#9265) ;
#6052=LINE('',#106906,#9266) ;
#6053=LINE('',#106946,#9267) ;
#6054=LINE('',#106948,#9268) ;
#6055=LINE('',#106984,#9269) ;
#6056=LINE('',#106986,#9270) ;
#6057=LINE('',#107026,#9271) ;
#6058=LINE('',#107028,#9272) ;
#6059=LINE('',#107064,#9273) ;
#6060=LINE('',#107066,#9274) ;
#6061=LINE('',#107106,#9275) ;
#6062=LINE('',#107108,#9276) ;
#6063=LINE('',#107144,#9277) ;
#6064=LINE('',#107146,#9278) ;
#6065=LINE('',#107186,#9279) ;
#6066=LINE('',#107188,#9280) ;
#6067=LINE('',#107224,#9281) ;
#6068=LINE('',#107226,#9282) ;
#6069=LINE('',#107266,#9283) ;
#6070=LINE('',#107268,#9284) ;
#6071=LINE('',#107304,#9285) ;
#6072=LINE('',#107306,#9286) ;
#6073=LINE('',#107345,#9287) ;
#6074=LINE('',#107346,#9288) ;
#6075=LINE('',#107349,#9289) ;
#6076=LINE('',#107351,#9290) ;
#6077=LINE('',#107352,#9291) ;
#6078=LINE('',#107355,#9292) ;
#6079=LINE('',#107359,#9293) ;
#6080=LINE('',#107360,#9294) ;
#6081=LINE('',#107363,#9295) ;
#6082=LINE('',#107367,#9296) ;
#6083=LINE('',#107368,#9297) ;
#6084=LINE('',#107371,#9298) ;
#6085=LINE('',#107375,#9299) ;
#6086=LINE('',#107376,#9300) ;
#6087=LINE('',#107379,#9301) ;
#6088=LINE('',#107383,#9302) ;
#6089=LINE('',#107384,#9303) ;
#6090=LINE('',#107387,#9304) ;
#6091=LINE('',#107391,#9305) ;
#6092=LINE('',#107392,#9306) ;
#6093=LINE('',#107395,#9307) ;
#6094=LINE('',#107399,#9308) ;
#6095=LINE('',#107400,#9309) ;
#6096=LINE('',#107403,#9310) ;
#6097=LINE('',#107407,#9311) ;
#6098=LINE('',#107408,#9312) ;
#6099=LINE('',#107411,#9313) ;
#6100=LINE('',#107415,#9314) ;
#6101=LINE('',#107416,#9315) ;
#6102=LINE('',#107419,#9316) ;
#6103=LINE('',#107423,#9317) ;
#6104=LINE('',#107424,#9318) ;
#6105=LINE('',#107427,#9319) ;
#6106=LINE('',#107431,#9320) ;
#6107=LINE('',#107432,#9321) ;
#6108=LINE('',#107435,#9322) ;
#6109=LINE('',#107439,#9323) ;
#6110=LINE('',#107440,#9324) ;
#6111=LINE('',#107443,#9325) ;
#6112=LINE('',#107447,#9326) ;
#6113=LINE('',#107448,#9327) ;
#6114=LINE('',#107451,#9328) ;
#6115=LINE('',#107455,#9329) ;
#6116=LINE('',#107456,#9330) ;
#6117=LINE('',#107459,#9331) ;
#6118=LINE('',#107463,#9332) ;
#6119=LINE('',#107464,#9333) ;
#6120=LINE('',#107467,#9334) ;
#6121=LINE('',#107471,#9335) ;
#6122=LINE('',#107472,#9336) ;
#6123=LINE('',#107475,#9337) ;
#6124=LINE('',#107479,#9338) ;
#6125=LINE('',#107480,#9339) ;
#6126=LINE('',#107483,#9340) ;
#6127=LINE('',#107487,#9341) ;
#6128=LINE('',#107488,#9342) ;
#6129=LINE('',#107491,#9343) ;
#6130=LINE('',#107495,#9344) ;
#6131=LINE('',#107496,#9345) ;
#6132=LINE('',#107499,#9346) ;
#6133=LINE('',#107503,#9347) ;
#6134=LINE('',#107504,#9348) ;
#6135=LINE('',#107507,#9349) ;
#6136=LINE('',#107639,#9350) ;
#6137=LINE('',#107642,#9351) ;
#6138=LINE('',#107645,#9352) ;
#6139=LINE('',#107648,#9353) ;
#6140=LINE('',#107651,#9354) ;
#6141=LINE('',#107654,#9355) ;
#6142=LINE('',#107657,#9356) ;
#6143=LINE('',#107660,#9357) ;
#6144=LINE('',#107663,#9358) ;
#6145=LINE('',#107666,#9359) ;
#6146=LINE('',#107669,#9360) ;
#6147=LINE('',#107672,#9361) ;
#6148=LINE('',#107675,#9362) ;
#6149=LINE('',#107678,#9363) ;
#6150=LINE('',#107681,#9364) ;
#6151=LINE('',#107684,#9365) ;
#6152=LINE('',#107687,#9366) ;
#6153=LINE('',#107690,#9367) ;
#6154=LINE('',#107693,#9368) ;
#6155=LINE('',#107696,#9369) ;
#6156=LINE('',#107699,#9370) ;
#6157=LINE('',#107702,#9371) ;
#6158=LINE('',#107705,#9372) ;
#6159=LINE('',#107708,#9373) ;
#6160=LINE('',#107711,#9374) ;
#6161=LINE('',#107714,#9375) ;
#6162=LINE('',#107717,#9376) ;
#6163=LINE('',#107720,#9377) ;
#6164=LINE('',#107723,#9378) ;
#6165=LINE('',#107726,#9379) ;
#6166=LINE('',#107729,#9380) ;
#6167=LINE('',#107732,#9381) ;
#6168=LINE('',#107735,#9382) ;
#6169=LINE('',#107738,#9383) ;
#6170=LINE('',#107741,#9384) ;
#6171=LINE('',#107744,#9385) ;
#6172=LINE('',#107747,#9386) ;
#6173=LINE('',#107750,#9387) ;
#6174=LINE('',#107753,#9388) ;
#6175=LINE('',#107756,#9389) ;
#6176=LINE('',#107807,#9390) ;
#6177=LINE('',#107810,#9391) ;
#6178=LINE('',#107843,#9392) ;
#6179=LINE('',#107895,#9393) ;
#6180=LINE('',#107992,#9394) ;
#6181=LINE('',#108089,#9395) ;
#6182=LINE('',#108186,#9396) ;
#6183=LINE('',#108283,#9397) ;
#6184=LINE('',#108380,#9398) ;
#6185=LINE('',#108477,#9399) ;
#6186=LINE('',#108574,#9400) ;
#6187=LINE('',#108783,#9401) ;
#6188=LINE('',#108822,#9402) ;
#6189=LINE('',#108861,#9403) ;
#6190=LINE('',#108900,#9404) ;
#6191=LINE('',#108939,#9405) ;
#6192=LINE('',#108978,#9406) ;
#6193=LINE('',#109017,#9407) ;
#6194=LINE('',#109056,#9408) ;
#6195=LINE('',#109095,#9409) ;
#6196=LINE('',#109117,#9410) ;
#6197=LINE('',#109118,#9411) ;
#6198=LINE('',#109120,#9412) ;
#6199=LINE('',#109122,#9413) ;
#6200=LINE('',#109125,#9414) ;
#6201=LINE('',#109126,#9415) ;
#6202=LINE('',#109128,#9416) ;
#6203=LINE('',#109129,#9417) ;
#6204=LINE('',#109132,#9418) ;
#6205=LINE('',#109133,#9419) ;
#6206=LINE('',#109135,#9420) ;
#6207=LINE('',#109136,#9421) ;
#6208=LINE('',#109139,#9422) ;
#6209=LINE('',#109140,#9423) ;
#6210=LINE('',#109142,#9424) ;
#6211=LINE('',#109143,#9425) ;
#6212=LINE('',#109146,#9426) ;
#6213=LINE('',#109147,#9427) ;
#6214=LINE('',#109149,#9428) ;
#6215=LINE('',#109150,#9429) ;
#6216=LINE('',#109153,#9430) ;
#6217=LINE('',#109154,#9431) ;
#6218=LINE('',#109156,#9432) ;
#6219=LINE('',#109157,#9433) ;
#6220=LINE('',#109160,#9434) ;
#6221=LINE('',#109161,#9435) ;
#6222=LINE('',#109163,#9436) ;
#6223=LINE('',#109164,#9437) ;
#6224=LINE('',#109167,#9438) ;
#6225=LINE('',#109168,#9439) ;
#6226=LINE('',#109170,#9440) ;
#6227=LINE('',#109171,#9441) ;
#6228=LINE('',#109174,#9442) ;
#6229=LINE('',#109175,#9443) ;
#6230=LINE('',#109177,#9444) ;
#6231=LINE('',#109178,#9445) ;
#6232=LINE('',#109181,#9446) ;
#6233=LINE('',#109182,#9447) ;
#6234=LINE('',#109184,#9448) ;
#6235=LINE('',#109196,#9449) ;
#9209=VECTOR('',#68566,10.) ;
#9210=VECTOR('',#68567,10.) ;
#9211=VECTOR('',#68576,10.) ;
#9212=VECTOR('',#68577,10.) ;
#9213=VECTOR('',#68586,10.) ;
#9214=VECTOR('',#68587,10.) ;
#9215=VECTOR('',#68596,10.) ;
#9216=VECTOR('',#68597,10.) ;
#9217=VECTOR('',#68606,10.) ;
#9218=VECTOR('',#68607,10.) ;
#9219=VECTOR('',#68616,10.) ;
#9220=VECTOR('',#68617,10.) ;
#9221=VECTOR('',#68626,10.) ;
#9222=VECTOR('',#68627,9.99999999999999) ;
#9223=VECTOR('',#68636,9.99999999999999) ;
#9224=VECTOR('',#68637,9.99999999999999) ;
#9225=VECTOR('',#68646,9.99999999999999) ;
#9226=VECTOR('',#68647,9.99999999999999) ;
#9227=VECTOR('',#68656,9.99999999999999) ;
#9228=VECTOR('',#68657,9.99999999999999) ;
#9229=VECTOR('',#68666,10.) ;
#9230=VECTOR('',#68667,10.) ;
#9231=VECTOR('',#68676,10.) ;
#9232=VECTOR('',#68677,10.) ;
#9233=VECTOR('',#68686,10.) ;
#9234=VECTOR('',#68687,10.) ;
#9235=VECTOR('',#68696,10.) ;
#9236=VECTOR('',#68697,10.) ;
#9237=VECTOR('',#68706,10.) ;
#9238=VECTOR('',#68707,10.) ;
#9239=VECTOR('',#68716,10.) ;
#9240=VECTOR('',#68717,10.) ;
#9241=VECTOR('',#68726,10.) ;
#9242=VECTOR('',#68727,10.) ;
#9243=VECTOR('',#68736,10.) ;
#9244=VECTOR('',#68737,10.) ;
#9245=VECTOR('',#68746,9.99999999999999) ;
#9246=VECTOR('',#68747,9.99999999999999) ;
#9247=VECTOR('',#68756,9.99999999999999) ;
#9248=VECTOR('',#68757,9.99999999999999) ;
#9249=VECTOR('',#68766,10.) ;
#9250=VECTOR('',#68767,10.) ;
#9251=VECTOR('',#68776,10.) ;
#9252=VECTOR('',#68777,10.) ;
#9253=VECTOR('',#68786,10.) ;
#9254=VECTOR('',#68787,10.) ;
#9255=VECTOR('',#68796,10.) ;
#9256=VECTOR('',#68797,10.) ;
#9257=VECTOR('',#68806,10.) ;
#9258=VECTOR('',#68807,10.) ;
#9259=VECTOR('',#68816,10.) ;
#9260=VECTOR('',#68817,10.) ;
#9261=VECTOR('',#68826,9.99999999999999) ;
#9262=VECTOR('',#68827,9.99999999999999) ;
#9263=VECTOR('',#68836,9.99999999999999) ;
#9264=VECTOR('',#68837,9.99999999999999) ;
#9265=VECTOR('',#68846,9.99999999999999) ;
#9266=VECTOR('',#68847,9.99999999999999) ;
#9267=VECTOR('',#68856,9.99999999999999) ;
#9268=VECTOR('',#68857,9.99999999999999) ;
#9269=VECTOR('',#68866,10.) ;
#9270=VECTOR('',#68867,10.) ;
#9271=VECTOR('',#68876,10.) ;
#9272=VECTOR('',#68877,10.) ;
#9273=VECTOR('',#68886,10.) ;
#9274=VECTOR('',#68887,10.) ;
#9275=VECTOR('',#68896,10.) ;
#9276=VECTOR('',#68897,10.) ;
#9277=VECTOR('',#68906,10.) ;
#9278=VECTOR('',#68907,10.) ;
#9279=VECTOR('',#68916,10.) ;
#9280=VECTOR('',#68917,10.) ;
#9281=VECTOR('',#68926,9.99999999999999) ;
#9282=VECTOR('',#68927,9.99999999999999) ;
#9283=VECTOR('',#68936,9.99999999999999) ;
#9284=VECTOR('',#68937,9.99999999999999) ;
#9285=VECTOR('',#68946,9.99999999999999) ;
#9286=VECTOR('',#68947,9.99999999999999) ;
#9287=VECTOR('',#68956,9.99999999999999) ;
#9288=VECTOR('',#68957,9.99999999999999) ;
#9289=VECTOR('',#68960,10.) ;
#9290=VECTOR('',#68961,10.) ;
#9291=VECTOR('',#68962,10.) ;
#9292=VECTOR('',#68965,10.) ;
#9293=VECTOR('',#68970,10.) ;
#9294=VECTOR('',#68971,10.) ;
#9295=VECTOR('',#68974,10.) ;
#9296=VECTOR('',#68979,10.) ;
#9297=VECTOR('',#68980,10.) ;
#9298=VECTOR('',#68983,10.) ;
#9299=VECTOR('',#68988,10.) ;
#9300=VECTOR('',#68989,10.) ;
#9301=VECTOR('',#68992,10.) ;
#9302=VECTOR('',#68997,10.) ;
#9303=VECTOR('',#68998,10.) ;
#9304=VECTOR('',#69001,10.) ;
#9305=VECTOR('',#69006,10.) ;
#9306=VECTOR('',#69007,10.) ;
#9307=VECTOR('',#69010,10.) ;
#9308=VECTOR('',#69015,10.) ;
#9309=VECTOR('',#69016,9.99999999999999) ;
#9310=VECTOR('',#69019,10.) ;
#9311=VECTOR('',#69024,10.) ;
#9312=VECTOR('',#69025,9.99999999999999) ;
#9313=VECTOR('',#69028,10.) ;
#9314=VECTOR('',#69033,10.) ;
#9315=VECTOR('',#69034,9.99999999999999) ;
#9316=VECTOR('',#69037,10.) ;
#9317=VECTOR('',#69042,10.) ;
#9318=VECTOR('',#69043,9.99999999999999) ;
#9319=VECTOR('',#69046,10.) ;
#9320=VECTOR('',#69051,10.) ;
#9321=VECTOR('',#69052,10.) ;
#9322=VECTOR('',#69055,10.) ;
#9323=VECTOR('',#69060,10.) ;
#9324=VECTOR('',#69061,10.) ;
#9325=VECTOR('',#69064,10.) ;
#9326=VECTOR('',#69069,10.) ;
#9327=VECTOR('',#69070,10.) ;
#9328=VECTOR('',#69073,10.) ;
#9329=VECTOR('',#69078,10.) ;
#9330=VECTOR('',#69079,10.) ;
#9331=VECTOR('',#69082,10.) ;
#9332=VECTOR('',#69087,10.) ;
#9333=VECTOR('',#69088,10.) ;
#9334=VECTOR('',#69091,10.) ;
#9335=VECTOR('',#69096,10.) ;
#9336=VECTOR('',#69097,10.) ;
#9337=VECTOR('',#69100,10.) ;
#9338=VECTOR('',#69105,10.) ;
#9339=VECTOR('',#69106,9.99999999999999) ;
#9340=VECTOR('',#69109,10.) ;
#9341=VECTOR('',#69114,10.) ;
#9342=VECTOR('',#69115,9.99999999999999) ;
#9343=VECTOR('',#69118,10.) ;
#9344=VECTOR('',#69123,10.) ;
#9345=VECTOR('',#69124,9.99999999999999) ;
#9346=VECTOR('',#69127,10.) ;
#9347=VECTOR('',#69132,10.) ;
#9348=VECTOR('',#69133,9.99999999999999) ;
#9349=VECTOR('',#69136,10.) ;
#9350=VECTOR('',#69313,10.) ;
#9351=VECTOR('',#69316,10.) ;
#9352=VECTOR('',#69319,9.99999999999999) ;
#9353=VECTOR('',#69322,9.99999999999999) ;
#9354=VECTOR('',#69325,10.) ;
#9355=VECTOR('',#69328,10.) ;
#9356=VECTOR('',#69331,10.) ;
#9357=VECTOR('',#69334,10.) ;
#9358=VECTOR('',#69337,10.) ;
#9359=VECTOR('',#69340,10.) ;
#9360=VECTOR('',#69343,10.) ;
#9361=VECTOR('',#69346,10.) ;
#9362=VECTOR('',#69349,9.99999999999999) ;
#9363=VECTOR('',#69352,9.99999999999999) ;
#9364=VECTOR('',#69355,9.99999999999999) ;
#9365=VECTOR('',#69358,9.99999999999999) ;
#9366=VECTOR('',#69361,10.) ;
#9367=VECTOR('',#69364,10.) ;
#9368=VECTOR('',#69367,10.) ;
#9369=VECTOR('',#69370,10.) ;
#9370=VECTOR('',#69373,10.) ;
#9371=VECTOR('',#69376,10.) ;
#9372=VECTOR('',#69379,9.99999999999999) ;
#9373=VECTOR('',#69382,9.99999999999999) ;
#9374=VECTOR('',#69385,9.99999999999999) ;
#9375=VECTOR('',#69388,9.99999999999999) ;
#9376=VECTOR('',#69391,10.) ;
#9377=VECTOR('',#69394,10.) ;
#9378=VECTOR('',#69397,10.) ;
#9379=VECTOR('',#69400,10.) ;
#9380=VECTOR('',#69403,10.) ;
#9381=VECTOR('',#69406,10.) ;
#9382=VECTOR('',#69409,9.99999999999999) ;
#9383=VECTOR('',#69412,9.99999999999999) ;
#9384=VECTOR('',#69415,9.99999999999999) ;
#9385=VECTOR('',#69418,9.99999999999999) ;
#9386=VECTOR('',#69421,10.) ;
#9387=VECTOR('',#69424,10.) ;
#9388=VECTOR('',#69427,10.) ;
#9389=VECTOR('',#69430,10.) ;
#9390=VECTOR('',#69437,10.) ;
#9391=VECTOR('',#69440,10.) ;
#9392=VECTOR('',#69443,10.) ;
#9393=VECTOR('',#69450,10.) ;
#9394=VECTOR('',#69459,9.99999999999999) ;
#9395=VECTOR('',#69468,9.99999999999999) ;
#9396=VECTOR('',#69477,10.) ;
#9397=VECTOR('',#69486,10.) ;
#9398=VECTOR('',#69495,10.) ;
#9399=VECTOR('',#69504,10.) ;
#9400=VECTOR('',#69513,9.99999999999999) ;
#9401=VECTOR('',#69538,9.99999999999999) ;
#9402=VECTOR('',#69551,10.) ;
#9403=VECTOR('',#69564,10.) ;
#9404=VECTOR('',#69577,10.) ;
#9405=VECTOR('',#69590,10.) ;
#9406=VECTOR('',#69603,9.99999999999999) ;
#9407=VECTOR('',#69616,9.99999999999999) ;
#9408=VECTOR('',#69629,10.) ;
#9409=VECTOR('',#69642,10.) ;
#9410=VECTOR('',#69653,10.) ;
#9411=VECTOR('',#69654,10.) ;
#9412=VECTOR('',#69657,10.) ;
#9413=VECTOR('',#69660,10.) ;
#9414=VECTOR('',#69665,10.) ;
#9415=VECTOR('',#69666,10.) ;
#9416=VECTOR('',#69669,10.) ;
#9417=VECTOR('',#69670,10.) ;
#9418=VECTOR('',#69675,10.) ;
#9419=VECTOR('',#69676,10.) ;
#9420=VECTOR('',#69679,10.) ;
#9421=VECTOR('',#69680,10.) ;
#9422=VECTOR('',#69685,10.) ;
#9423=VECTOR('',#69686,10.) ;
#9424=VECTOR('',#69689,10.) ;
#9425=VECTOR('',#69690,10.) ;
#9426=VECTOR('',#69695,10.) ;
#9427=VECTOR('',#69696,10.) ;
#9428=VECTOR('',#69699,10.) ;
#9429=VECTOR('',#69700,10.) ;
#9430=VECTOR('',#69705,10.) ;
#9431=VECTOR('',#69706,10.) ;
#9432=VECTOR('',#69709,10.) ;
#9433=VECTOR('',#69710,10.) ;
#9434=VECTOR('',#69715,10.) ;
#9435=VECTOR('',#69716,10.) ;
#9436=VECTOR('',#69719,10.) ;
#9437=VECTOR('',#69720,10.) ;
#9438=VECTOR('',#69725,10.) ;
#9439=VECTOR('',#69726,10.) ;
#9440=VECTOR('',#69729,10.) ;
#9441=VECTOR('',#69730,10.) ;
#9442=VECTOR('',#69735,10.) ;
#9443=VECTOR('',#69736,10.) ;
#9444=VECTOR('',#69739,10.) ;
#9445=VECTOR('',#69740,10.) ;
#9446=VECTOR('',#69745,10.) ;
#9447=VECTOR('',#69746,10.) ;
#9448=VECTOR('',#69749,10.) ;
#9449=VECTOR('',#69772,2.) ;
#10613=CYLINDRICAL_SURFACE('',#54562,0.15) ;
#10614=CYLINDRICAL_SURFACE('',#54566,0.15) ;
#10615=CYLINDRICAL_SURFACE('',#54570,0.15) ;
#10616=CYLINDRICAL_SURFACE('',#54574,0.15) ;
#10617=CYLINDRICAL_SURFACE('',#54578,0.15) ;
#10618=CYLINDRICAL_SURFACE('',#54582,0.15) ;
#10619=CYLINDRICAL_SURFACE('',#54586,0.15) ;
#10620=CYLINDRICAL_SURFACE('',#54590,0.15) ;
#10621=CYLINDRICAL_SURFACE('',#54594,0.15) ;
#10622=CYLINDRICAL_SURFACE('',#54598,0.15) ;
#10623=CYLINDRICAL_SURFACE('',#54602,0.15) ;
#10624=CYLINDRICAL_SURFACE('',#54606,0.15) ;
#10625=CYLINDRICAL_SURFACE('',#54610,0.15) ;
#10626=CYLINDRICAL_SURFACE('',#54614,0.15) ;
#10627=CYLINDRICAL_SURFACE('',#54618,0.15) ;
#10628=CYLINDRICAL_SURFACE('',#54622,0.15) ;
#10629=CYLINDRICAL_SURFACE('',#54626,0.15) ;
#10630=CYLINDRICAL_SURFACE('',#54630,0.15) ;
#10631=CYLINDRICAL_SURFACE('',#54634,0.15) ;
#10632=CYLINDRICAL_SURFACE('',#54638,0.15) ;
#10633=CYLINDRICAL_SURFACE('',#54642,0.15) ;
#10634=CYLINDRICAL_SURFACE('',#54646,0.15) ;
#10635=CYLINDRICAL_SURFACE('',#54650,0.15) ;
#10636=CYLINDRICAL_SURFACE('',#54654,0.15) ;
#10637=CYLINDRICAL_SURFACE('',#54658,0.15) ;
#10638=CYLINDRICAL_SURFACE('',#54662,0.15) ;
#10639=CYLINDRICAL_SURFACE('',#54666,0.15) ;
#10640=CYLINDRICAL_SURFACE('',#54670,0.15) ;
#10641=CYLINDRICAL_SURFACE('',#54674,0.15) ;
#10642=CYLINDRICAL_SURFACE('',#54678,0.15) ;
#10643=CYLINDRICAL_SURFACE('',#54682,0.15) ;
#10644=CYLINDRICAL_SURFACE('',#54686,0.15) ;
#10645=CYLINDRICAL_SURFACE('',#54690,0.15) ;
#10646=CYLINDRICAL_SURFACE('',#54694,0.15) ;
#10647=CYLINDRICAL_SURFACE('',#54698,0.15) ;
#10648=CYLINDRICAL_SURFACE('',#54702,0.15) ;
#10649=CYLINDRICAL_SURFACE('',#54706,0.15) ;
#10650=CYLINDRICAL_SURFACE('',#54710,0.15) ;
#10651=CYLINDRICAL_SURFACE('',#54714,0.15) ;
#10652=CYLINDRICAL_SURFACE('',#54718,0.15) ;
#10653=CYLINDRICAL_SURFACE('',#54720,0.500000000000003) ;
#10654=CYLINDRICAL_SURFACE('',#54723,5.1) ;
#10655=CYLINDRICAL_SURFACE('',#54726,0.500000000000003) ;
#10656=CYLINDRICAL_SURFACE('',#54729,5.1) ;
#10657=CYLINDRICAL_SURFACE('',#54732,0.500000000000003) ;
#10658=CYLINDRICAL_SURFACE('',#54735,5.1) ;
#10659=CYLINDRICAL_SURFACE('',#54738,0.500000000000003) ;
#10660=CYLINDRICAL_SURFACE('',#54741,5.1) ;
#10661=CYLINDRICAL_SURFACE('',#54744,0.500000000000003) ;
#10662=CYLINDRICAL_SURFACE('',#54747,5.1) ;
#10663=CYLINDRICAL_SURFACE('',#54750,0.500000000000003) ;
#10664=CYLINDRICAL_SURFACE('',#54753,5.1) ;
#10665=CYLINDRICAL_SURFACE('',#54756,0.500000000000003) ;
#10666=CYLINDRICAL_SURFACE('',#54759,5.1) ;
#10667=CYLINDRICAL_SURFACE('',#54762,0.500000000000003) ;
#10668=CYLINDRICAL_SURFACE('',#54765,5.1) ;
#10669=CYLINDRICAL_SURFACE('',#54768,0.500000000000003) ;
#10670=CYLINDRICAL_SURFACE('',#54771,5.1) ;
#10671=CYLINDRICAL_SURFACE('',#54774,0.500000000000003) ;
#10672=CYLINDRICAL_SURFACE('',#54777,5.1) ;
#10673=CYLINDRICAL_SURFACE('',#54907,0.15) ;
#10674=CYLINDRICAL_SURFACE('',#54908,0.15) ;
#10675=CYLINDRICAL_SURFACE('',#54909,0.15) ;
#10676=CYLINDRICAL_SURFACE('',#54911,0.15) ;
#10677=CYLINDRICAL_SURFACE('',#54912,0.15) ;
#10678=CYLINDRICAL_SURFACE('',#54913,0.15) ;
#10679=CYLINDRICAL_SURFACE('',#54915,0.15) ;
#10680=CYLINDRICAL_SURFACE('',#54916,0.15) ;
#10681=CYLINDRICAL_SURFACE('',#54917,0.15) ;
#10682=CYLINDRICAL_SURFACE('',#54919,0.15) ;
#10683=CYLINDRICAL_SURFACE('',#54920,0.15) ;
#10684=CYLINDRICAL_SURFACE('',#54921,0.15) ;
#10685=CYLINDRICAL_SURFACE('',#54923,0.15) ;
#10686=CYLINDRICAL_SURFACE('',#54924,0.15) ;
#10687=CYLINDRICAL_SURFACE('',#54925,0.15) ;
#10688=CYLINDRICAL_SURFACE('',#54927,0.15) ;
#10689=CYLINDRICAL_SURFACE('',#54928,0.15) ;
#10690=CYLINDRICAL_SURFACE('',#54929,0.15) ;
#10691=CYLINDRICAL_SURFACE('',#54931,0.15) ;
#10692=CYLINDRICAL_SURFACE('',#54932,0.15) ;
#10693=CYLINDRICAL_SURFACE('',#54933,0.15) ;
#10694=CYLINDRICAL_SURFACE('',#54935,0.15) ;
#10695=CYLINDRICAL_SURFACE('',#54936,0.15) ;
#10696=CYLINDRICAL_SURFACE('',#54937,0.15) ;
#10697=CYLINDRICAL_SURFACE('',#54939,0.15) ;
#10698=CYLINDRICAL_SURFACE('',#54940,0.15) ;
#10699=CYLINDRICAL_SURFACE('',#54941,0.15) ;
#10700=CYLINDRICAL_SURFACE('',#54943,0.15) ;
#10701=CYLINDRICAL_SURFACE('',#54944,0.15) ;
#10702=CYLINDRICAL_SURFACE('',#54945,0.15) ;
#10703=CYLINDRICAL_SURFACE('',#54947,0.15) ;
#10704=CYLINDRICAL_SURFACE('',#54952,0.15) ;
#10705=CYLINDRICAL_SURFACE('',#54958,0.15) ;
#10706=CYLINDRICAL_SURFACE('',#54964,0.15) ;
#10707=CYLINDRICAL_SURFACE('',#54970,0.15) ;
#10708=CYLINDRICAL_SURFACE('',#54976,0.15) ;
#10709=CYLINDRICAL_SURFACE('',#54982,0.15) ;
#10710=CYLINDRICAL_SURFACE('',#54988,0.15) ;
#10711=CYLINDRICAL_SURFACE('',#54994,0.15) ;
#10712=CYLINDRICAL_SURFACE('',#55000,0.15) ;
#10713=CYLINDRICAL_SURFACE('',#55005,5.1) ;
#10714=CYLINDRICAL_SURFACE('',#55007,0.500000000000003) ;
#10715=CYLINDRICAL_SURFACE('',#55011,0.500000000000003) ;
#10716=CYLINDRICAL_SURFACE('',#55014,0.500000000000003) ;
#10717=CYLINDRICAL_SURFACE('',#55017,0.500000000000003) ;
#10718=CYLINDRICAL_SURFACE('',#55020,0.500000000000003) ;
#10719=CYLINDRICAL_SURFACE('',#55023,0.500000000000003) ;
#10720=CYLINDRICAL_SURFACE('',#55026,0.500000000000003) ;
#10721=CYLINDRICAL_SURFACE('',#55029,0.500000000000003) ;
#10722=CYLINDRICAL_SURFACE('',#55032,0.500000000000003) ;
#10723=CYLINDRICAL_SURFACE('',#55035,0.500000000000003) ;
#10724=CYLINDRICAL_SURFACE('',#55036,5.1) ;
#10725=CYLINDRICAL_SURFACE('',#55037,5.1) ;
#10726=CYLINDRICAL_SURFACE('',#55038,5.1) ;
#10727=CYLINDRICAL_SURFACE('',#55039,5.1) ;
#10728=CYLINDRICAL_SURFACE('',#55040,5.1) ;
#10729=CYLINDRICAL_SURFACE('',#55041,5.1) ;
#10730=CYLINDRICAL_SURFACE('',#55042,5.1) ;
#10731=CYLINDRICAL_SURFACE('',#55043,5.1) ;
#10732=CYLINDRICAL_SURFACE('',#55044,5.1) ;
#10733=CYLINDRICAL_SURFACE('',#55045,2.) ;
#13525=FACE_OUTER_BOUND('',#16713,.T.) ;
#13526=FACE_OUTER_BOUND('',#16714,.T.) ;
#13527=FACE_OUTER_BOUND('',#16716,.T.) ;
#13528=FACE_OUTER_BOUND('',#16717,.T.) ;
#13529=FACE_OUTER_BOUND('',#16719,.T.) ;
#13530=FACE_OUTER_BOUND('',#16721,.T.) ;
#13531=FACE_OUTER_BOUND('',#16723,.T.) ;
#13532=FACE_OUTER_BOUND('',#16724,.T.) ;
#13533=FACE_OUTER_BOUND('',#16725,.T.) ;
#13534=FACE_OUTER_BOUND('',#16726,.T.) ;
#13535=FACE_OUTER_BOUND('',#16727,.T.) ;
#13536=FACE_OUTER_BOUND('',#16728,.T.) ;
#13537=FACE_OUTER_BOUND('',#16729,.T.) ;
#13538=FACE_OUTER_BOUND('',#16730,.T.) ;
#13539=FACE_OUTER_BOUND('',#16731,.T.) ;
#13540=FACE_OUTER_BOUND('',#16732,.T.) ;
#13541=FACE_OUTER_BOUND('',#16733,.T.) ;
#13542=FACE_OUTER_BOUND('',#16734,.T.) ;
#13543=FACE_OUTER_BOUND('',#16735,.T.) ;
#13544=FACE_OUTER_BOUND('',#16736,.T.) ;
#13545=FACE_OUTER_BOUND('',#16737,.T.) ;
#13546=FACE_OUTER_BOUND('',#16738,.T.) ;
#13547=FACE_OUTER_BOUND('',#16739,.T.) ;
#13548=FACE_OUTER_BOUND('',#16740,.T.) ;
#13549=FACE_OUTER_BOUND('',#16741,.T.) ;
#13550=FACE_OUTER_BOUND('',#16742,.T.) ;
#13551=FACE_OUTER_BOUND('',#16743,.T.) ;
#13552=FACE_OUTER_BOUND('',#16744,.T.) ;
#13553=FACE_OUTER_BOUND('',#16745,.T.) ;
#13554=FACE_OUTER_BOUND('',#16746,.T.) ;
#13555=FACE_OUTER_BOUND('',#16747,.T.) ;
#13556=FACE_OUTER_BOUND('',#16748,.T.) ;
#13557=FACE_OUTER_BOUND('',#16749,.T.) ;
#13558=FACE_OUTER_BOUND('',#16750,.T.) ;
#13559=FACE_OUTER_BOUND('',#16751,.T.) ;
#13560=FACE_OUTER_BOUND('',#16752,.T.) ;
#13561=FACE_OUTER_BOUND('',#16753,.T.) ;
#13562=FACE_OUTER_BOUND('',#16754,.T.) ;
#13563=FACE_OUTER_BOUND('',#16755,.T.) ;
#13564=FACE_OUTER_BOUND('',#16756,.T.) ;
#13565=FACE_OUTER_BOUND('',#16757,.T.) ;
#13566=FACE_OUTER_BOUND('',#16758,.T.) ;
#13567=FACE_OUTER_BOUND('',#16759,.T.) ;
#13568=FACE_OUTER_BOUND('',#16760,.T.) ;
#13569=FACE_OUTER_BOUND('',#16761,.T.) ;
#13570=FACE_OUTER_BOUND('',#16762,.T.) ;
#13571=FACE_OUTER_BOUND('',#16763,.T.) ;
#13572=FACE_OUTER_BOUND('',#16764,.T.) ;
#13573=FACE_OUTER_BOUND('',#16765,.T.) ;
#13574=FACE_OUTER_BOUND('',#16766,.T.) ;
#13575=FACE_OUTER_BOUND('',#16767,.T.) ;
#13576=FACE_OUTER_BOUND('',#16768,.T.) ;
#13577=FACE_OUTER_BOUND('',#16769,.T.) ;
#13578=FACE_OUTER_BOUND('',#16770,.T.) ;
#13579=FACE_OUTER_BOUND('',#16771,.T.) ;
#13580=FACE_OUTER_BOUND('',#16772,.T.) ;
#13581=FACE_OUTER_BOUND('',#16773,.T.) ;
#13582=FACE_OUTER_BOUND('',#16774,.T.) ;
#13583=FACE_OUTER_BOUND('',#16775,.T.) ;
#13584=FACE_OUTER_BOUND('',#16776,.T.) ;
#13585=FACE_OUTER_BOUND('',#16777,.T.) ;
#13586=FACE_OUTER_BOUND('',#16778,.T.) ;
#13587=FACE_OUTER_BOUND('',#16779,.T.) ;
#13588=FACE_OUTER_BOUND('',#16780,.T.) ;
#13589=FACE_OUTER_BOUND('',#16781,.T.) ;
#13590=FACE_OUTER_BOUND('',#16782,.T.) ;
#13591=FACE_OUTER_BOUND('',#16783,.T.) ;
#13592=FACE_OUTER_BOUND('',#16784,.T.) ;
#13593=FACE_OUTER_BOUND('',#16785,.T.) ;
#13594=FACE_OUTER_BOUND('',#16786,.T.) ;
#13595=FACE_OUTER_BOUND('',#16787,.T.) ;
#13596=FACE_OUTER_BOUND('',#16788,.T.) ;
#13597=FACE_OUTER_BOUND('',#16789,.T.) ;
#13598=FACE_OUTER_BOUND('',#16790,.T.) ;
#13599=FACE_OUTER_BOUND('',#16791,.T.) ;
#13600=FACE_OUTER_BOUND('',#16792,.T.) ;
#13601=FACE_OUTER_BOUND('',#16793,.T.) ;
#13602=FACE_OUTER_BOUND('',#16794,.T.) ;
#13603=FACE_OUTER_BOUND('',#16795,.T.) ;
#13604=FACE_OUTER_BOUND('',#16796,.T.) ;
#13605=FACE_OUTER_BOUND('',#16797,.T.) ;
#13606=FACE_OUTER_BOUND('',#16798,.T.) ;
#13607=FACE_OUTER_BOUND('',#16799,.T.) ;
#13608=FACE_OUTER_BOUND('',#16800,.T.) ;
#13609=FACE_OUTER_BOUND('',#16801,.T.) ;
#13610=FACE_OUTER_BOUND('',#16802,.T.) ;
#13611=FACE_OUTER_BOUND('',#16803,.T.) ;
#13612=FACE_OUTER_BOUND('',#16804,.T.) ;
#13613=FACE_OUTER_BOUND('',#16805,.T.) ;
#13614=FACE_OUTER_BOUND('',#16806,.T.) ;
#13615=FACE_OUTER_BOUND('',#16807,.T.) ;
#13616=FACE_OUTER_BOUND('',#16808,.T.) ;
#13617=FACE_OUTER_BOUND('',#16809,.T.) ;
#13618=FACE_OUTER_BOUND('',#16810,.T.) ;
#13619=FACE_OUTER_BOUND('',#16811,.T.) ;
#13620=FACE_OUTER_BOUND('',#16812,.T.) ;
#13621=FACE_OUTER_BOUND('',#16813,.T.) ;
#13622=FACE_OUTER_BOUND('',#16814,.T.) ;
#13623=FACE_OUTER_BOUND('',#16815,.T.) ;
#13624=FACE_OUTER_BOUND('',#16816,.T.) ;
#13625=FACE_OUTER_BOUND('',#16817,.T.) ;
#13626=FACE_OUTER_BOUND('',#16818,.T.) ;
#13627=FACE_OUTER_BOUND('',#16819,.T.) ;
#13628=FACE_OUTER_BOUND('',#16820,.T.) ;
#13629=FACE_OUTER_BOUND('',#16821,.T.) ;
#13630=FACE_OUTER_BOUND('',#16822,.T.) ;
#13631=FACE_OUTER_BOUND('',#16823,.T.) ;
#13632=FACE_OUTER_BOUND('',#16824,.T.) ;
#13633=FACE_OUTER_BOUND('',#16825,.T.) ;
#13634=FACE_OUTER_BOUND('',#16826,.T.) ;
#13635=FACE_OUTER_BOUND('',#16827,.T.) ;
#13636=FACE_OUTER_BOUND('',#16828,.T.) ;
#13637=FACE_OUTER_BOUND('',#16829,.T.) ;
#13638=FACE_OUTER_BOUND('',#16830,.T.) ;
#13639=FACE_OUTER_BOUND('',#16831,.T.) ;
#13640=FACE_OUTER_BOUND('',#16832,.T.) ;
#13641=FACE_OUTER_BOUND('',#16833,.T.) ;
#13642=FACE_OUTER_BOUND('',#16834,.T.) ;
#13643=FACE_OUTER_BOUND('',#16835,.T.) ;
#13644=FACE_OUTER_BOUND('',#16836,.T.) ;
#13645=FACE_OUTER_BOUND('',#16837,.T.) ;
#13646=FACE_OUTER_BOUND('',#16838,.T.) ;
#13647=FACE_OUTER_BOUND('',#16839,.T.) ;
#13648=FACE_OUTER_BOUND('',#16840,.T.) ;
#13649=FACE_OUTER_BOUND('',#16841,.T.) ;
#13650=FACE_OUTER_BOUND('',#16842,.T.) ;
#13651=FACE_OUTER_BOUND('',#16843,.T.) ;
#13652=FACE_OUTER_BOUND('',#16844,.T.) ;
#13653=FACE_OUTER_BOUND('',#16845,.T.) ;
#13654=FACE_OUTER_BOUND('',#16846,.T.) ;
#13655=FACE_OUTER_BOUND('',#16847,.T.) ;
#13656=FACE_OUTER_BOUND('',#16848,.T.) ;
#13657=FACE_OUTER_BOUND('',#16849,.T.) ;
#13658=FACE_OUTER_BOUND('',#16850,.T.) ;
#13659=FACE_OUTER_BOUND('',#16851,.T.) ;
#13660=FACE_OUTER_BOUND('',#16852,.T.) ;
#13661=FACE_OUTER_BOUND('',#16853,.T.) ;
#13662=FACE_OUTER_BOUND('',#16854,.T.) ;
#13663=FACE_OUTER_BOUND('',#16855,.T.) ;
#13664=FACE_OUTER_BOUND('',#16856,.T.) ;
#13665=FACE_OUTER_BOUND('',#16857,.T.) ;
#13666=FACE_OUTER_BOUND('',#16858,.T.) ;
#13667=FACE_OUTER_BOUND('',#16859,.T.) ;
#13668=FACE_OUTER_BOUND('',#16860,.T.) ;
#13669=FACE_OUTER_BOUND('',#16861,.T.) ;
#13670=FACE_OUTER_BOUND('',#16862,.T.) ;
#13671=FACE_OUTER_BOUND('',#16863,.T.) ;
#13672=FACE_OUTER_BOUND('',#16864,.T.) ;
#13673=FACE_OUTER_BOUND('',#16865,.T.) ;
#13674=FACE_OUTER_BOUND('',#16866,.T.) ;
#13675=FACE_OUTER_BOUND('',#16867,.T.) ;
#13676=FACE_OUTER_BOUND('',#16868,.T.) ;
#13677=FACE_OUTER_BOUND('',#16869,.T.) ;
#13678=FACE_OUTER_BOUND('',#16870,.T.) ;
#13679=FACE_OUTER_BOUND('',#16871,.T.) ;
#13680=FACE_OUTER_BOUND('',#16872,.T.) ;
#13681=FACE_OUTER_BOUND('',#16873,.T.) ;
#13682=FACE_OUTER_BOUND('',#16874,.T.) ;
#13683=FACE_OUTER_BOUND('',#16875,.T.) ;
#13684=FACE_OUTER_BOUND('',#16876,.T.) ;
#13685=FACE_OUTER_BOUND('',#16877,.T.) ;
#13686=FACE_OUTER_BOUND('',#16878,.T.) ;
#13687=FACE_OUTER_BOUND('',#16879,.T.) ;
#13688=FACE_OUTER_BOUND('',#16880,.T.) ;
#13689=FACE_OUTER_BOUND('',#16881,.T.) ;
#13690=FACE_OUTER_BOUND('',#16882,.T.) ;
#13691=FACE_OUTER_BOUND('',#16883,.T.) ;
#13692=FACE_OUTER_BOUND('',#16884,.T.) ;
#13693=FACE_OUTER_BOUND('',#16885,.T.) ;
#13694=FACE_OUTER_BOUND('',#16886,.T.) ;
#13695=FACE_OUTER_BOUND('',#16887,.T.) ;
#13696=FACE_OUTER_BOUND('',#16888,.T.) ;
#13697=FACE_OUTER_BOUND('',#16889,.T.) ;
#13698=FACE_OUTER_BOUND('',#16890,.T.) ;
#13699=FACE_OUTER_BOUND('',#16891,.T.) ;
#13700=FACE_OUTER_BOUND('',#16892,.T.) ;
#13701=FACE_OUTER_BOUND('',#16893,.T.) ;
#13702=FACE_OUTER_BOUND('',#16894,.T.) ;
#13703=FACE_OUTER_BOUND('',#16895,.T.) ;
#13704=FACE_OUTER_BOUND('',#16896,.T.) ;
#13705=FACE_OUTER_BOUND('',#16897,.T.) ;
#13706=FACE_OUTER_BOUND('',#16898,.T.) ;
#13707=FACE_OUTER_BOUND('',#16899,.T.) ;
#13708=FACE_OUTER_BOUND('',#16900,.T.) ;
#13709=FACE_OUTER_BOUND('',#16901,.T.) ;
#13710=FACE_OUTER_BOUND('',#16902,.T.) ;
#13711=FACE_OUTER_BOUND('',#16903,.T.) ;
#13712=FACE_OUTER_BOUND('',#16904,.T.) ;
#13713=FACE_OUTER_BOUND('',#16905,.T.) ;
#13714=FACE_OUTER_BOUND('',#16906,.T.) ;
#13715=FACE_OUTER_BOUND('',#16907,.T.) ;
#13716=FACE_OUTER_BOUND('',#16908,.T.) ;
#13717=FACE_OUTER_BOUND('',#16909,.T.) ;
#13718=FACE_OUTER_BOUND('',#16910,.T.) ;
#13719=FACE_OUTER_BOUND('',#16911,.T.) ;
#13720=FACE_OUTER_BOUND('',#16912,.T.) ;
#13721=FACE_OUTER_BOUND('',#16913,.T.) ;
#13722=FACE_OUTER_BOUND('',#16914,.T.) ;
#13723=FACE_OUTER_BOUND('',#16915,.T.) ;
#13724=FACE_OUTER_BOUND('',#16916,.T.) ;
#13725=FACE_OUTER_BOUND('',#16917,.T.) ;
#13726=FACE_OUTER_BOUND('',#16918,.T.) ;
#13727=FACE_OUTER_BOUND('',#16919,.T.) ;
#13728=FACE_OUTER_BOUND('',#16920,.T.) ;
#13729=FACE_OUTER_BOUND('',#16921,.T.) ;
#13730=FACE_OUTER_BOUND('',#16922,.T.) ;
#13731=FACE_OUTER_BOUND('',#16923,.T.) ;
#13732=FACE_OUTER_BOUND('',#16924,.T.) ;
#13733=FACE_OUTER_BOUND('',#16925,.T.) ;
#13734=FACE_OUTER_BOUND('',#16926,.T.) ;
#13735=FACE_OUTER_BOUND('',#16927,.T.) ;
#13736=FACE_OUTER_BOUND('',#16928,.T.) ;
#13737=FACE_OUTER_BOUND('',#16929,.T.) ;
#13738=FACE_OUTER_BOUND('',#16930,.T.) ;
#13739=FACE_OUTER_BOUND('',#16931,.T.) ;
#13740=FACE_OUTER_BOUND('',#16932,.T.) ;
#13741=FACE_OUTER_BOUND('',#16933,.T.) ;
#13742=FACE_OUTER_BOUND('',#16934,.T.) ;
#13743=FACE_OUTER_BOUND('',#16935,.T.) ;
#13744=FACE_OUTER_BOUND('',#16936,.T.) ;
#13745=FACE_OUTER_BOUND('',#16937,.T.) ;
#13746=FACE_OUTER_BOUND('',#16938,.T.) ;
#13747=FACE_OUTER_BOUND('',#16939,.T.) ;
#13748=FACE_OUTER_BOUND('',#16940,.T.) ;
#13749=FACE_OUTER_BOUND('',#16941,.T.) ;
#13750=FACE_OUTER_BOUND('',#16942,.T.) ;
#13751=FACE_OUTER_BOUND('',#16943,.T.) ;
#13752=FACE_OUTER_BOUND('',#16944,.T.) ;
#13753=FACE_OUTER_BOUND('',#16945,.T.) ;
#13754=FACE_OUTER_BOUND('',#16946,.T.) ;
#13755=FACE_OUTER_BOUND('',#16947,.T.) ;
#13756=FACE_OUTER_BOUND('',#16948,.T.) ;
#13757=FACE_OUTER_BOUND('',#16949,.T.) ;
#13758=FACE_OUTER_BOUND('',#16950,.T.) ;
#13759=FACE_OUTER_BOUND('',#16951,.T.) ;
#13760=FACE_OUTER_BOUND('',#16952,.T.) ;
#13761=FACE_OUTER_BOUND('',#16953,.T.) ;
#13762=FACE_OUTER_BOUND('',#16954,.T.) ;
#13763=FACE_OUTER_BOUND('',#16955,.T.) ;
#13764=FACE_OUTER_BOUND('',#16956,.T.) ;
#13765=FACE_OUTER_BOUND('',#16957,.T.) ;
#13766=FACE_OUTER_BOUND('',#16958,.T.) ;
#13767=FACE_OUTER_BOUND('',#16959,.T.) ;
#13768=FACE_OUTER_BOUND('',#16960,.T.) ;
#13769=FACE_OUTER_BOUND('',#16961,.T.) ;
#13770=FACE_OUTER_BOUND('',#16962,.T.) ;
#13771=FACE_OUTER_BOUND('',#16963,.T.) ;
#13772=FACE_OUTER_BOUND('',#16964,.T.) ;
#13773=FACE_OUTER_BOUND('',#16965,.T.) ;
#13774=FACE_OUTER_BOUND('',#16966,.T.) ;
#13775=FACE_OUTER_BOUND('',#16967,.T.) ;
#13776=FACE_OUTER_BOUND('',#16968,.T.) ;
#13777=FACE_OUTER_BOUND('',#16969,.T.) ;
#13778=FACE_OUTER_BOUND('',#16970,.T.) ;
#13779=FACE_OUTER_BOUND('',#16971,.T.) ;
#13780=FACE_OUTER_BOUND('',#16972,.T.) ;
#13781=FACE_OUTER_BOUND('',#16973,.T.) ;
#13782=FACE_OUTER_BOUND('',#16974,.T.) ;
#13783=FACE_OUTER_BOUND('',#16975,.T.) ;
#13784=FACE_OUTER_BOUND('',#16976,.T.) ;
#13785=FACE_OUTER_BOUND('',#16977,.T.) ;
#13786=FACE_OUTER_BOUND('',#16978,.T.) ;
#13787=FACE_OUTER_BOUND('',#16979,.T.) ;
#13788=FACE_OUTER_BOUND('',#16980,.T.) ;
#13789=FACE_OUTER_BOUND('',#16981,.T.) ;
#13790=FACE_OUTER_BOUND('',#16982,.T.) ;
#13791=FACE_OUTER_BOUND('',#16983,.T.) ;
#13792=FACE_OUTER_BOUND('',#16984,.T.) ;
#13793=FACE_OUTER_BOUND('',#16985,.T.) ;
#13794=FACE_OUTER_BOUND('',#16986,.T.) ;
#13795=FACE_OUTER_BOUND('',#16987,.T.) ;
#13796=FACE_OUTER_BOUND('',#16988,.T.) ;
#13797=FACE_OUTER_BOUND('',#16989,.T.) ;
#13798=FACE_OUTER_BOUND('',#16990,.T.) ;
#13799=FACE_OUTER_BOUND('',#16991,.T.) ;
#13800=FACE_OUTER_BOUND('',#16992,.T.) ;
#13801=FACE_OUTER_BOUND('',#16993,.T.) ;
#13802=FACE_OUTER_BOUND('',#16994,.T.) ;
#13803=FACE_OUTER_BOUND('',#16995,.T.) ;
#13804=FACE_OUTER_BOUND('',#16996,.T.) ;
#13805=FACE_OUTER_BOUND('',#16997,.T.) ;
#13806=FACE_OUTER_BOUND('',#16998,.T.) ;
#13807=FACE_OUTER_BOUND('',#16999,.T.) ;
#13808=FACE_OUTER_BOUND('',#17000,.T.) ;
#13809=FACE_OUTER_BOUND('',#17001,.T.) ;
#13810=FACE_OUTER_BOUND('',#17002,.T.) ;
#13811=FACE_OUTER_BOUND('',#17003,.T.) ;
#13812=FACE_OUTER_BOUND('',#17004,.T.) ;
#13813=FACE_OUTER_BOUND('',#17005,.T.) ;
#13814=FACE_OUTER_BOUND('',#17006,.T.) ;
#13815=FACE_OUTER_BOUND('',#17007,.T.) ;
#16713=EDGE_LOOP('',(#44006,#44007,#44008,#44009)) ;
#16714=EDGE_LOOP('',(#44010)) ;
#16715=EDGE_LOOP('',(#44011)) ;
#16716=EDGE_LOOP('',(#44012,#44013,#44014,#44015)) ;
#16717=EDGE_LOOP('',(#44016)) ;
#16718=EDGE_LOOP('',(#44017)) ;
#16719=EDGE_LOOP('',(#44018)) ;
#16720=EDGE_LOOP('',(#44019)) ;
#16721=EDGE_LOOP('',(#44020)) ;
#16722=EDGE_LOOP('',(#44021)) ;
#16723=EDGE_LOOP('',(#44022,#44023,#44024,#44025,#44026)) ;
#16724=EDGE_LOOP('',(#44027,#44028,#44029,#44030,#44031)) ;
#16725=EDGE_LOOP('',(#44032,#44033,#44034,#44035)) ;
#16726=EDGE_LOOP('',(#44036,#44037,#44038,#44039)) ;
#16727=EDGE_LOOP('',(#44040,#44041,#44042,#44043)) ;
#16728=EDGE_LOOP('',(#44044,#44045,#44046,#44047)) ;
#16729=EDGE_LOOP('',(#44048,#44049,#44050,#44051)) ;
#16730=EDGE_LOOP('',(#44052,#44053,#44054,#44055)) ;
#16731=EDGE_LOOP('',(#44056,#44057,#44058,#44059)) ;
#16732=EDGE_LOOP('',(#44060,#44061,#44062,#44063)) ;
#16733=EDGE_LOOP('',(#44064,#44065,#44066,#44067)) ;
#16734=EDGE_LOOP('',(#44068,#44069,#44070,#44071)) ;
#16735=EDGE_LOOP('',(#44072,#44073,#44074,#44075)) ;
#16736=EDGE_LOOP('',(#44076,#44077,#44078,#44079)) ;
#16737=EDGE_LOOP('',(#44080,#44081,#44082,#44083)) ;
#16738=EDGE_LOOP('',(#44084,#44085,#44086,#44087)) ;
#16739=EDGE_LOOP('',(#44088,#44089,#44090,#44091)) ;
#16740=EDGE_LOOP('',(#44092,#44093,#44094,#44095)) ;
#16741=EDGE_LOOP('',(#44096,#44097,#44098,#44099)) ;
#16742=EDGE_LOOP('',(#44100,#44101,#44102,#44103)) ;
#16743=EDGE_LOOP('',(#44104,#44105,#44106,#44107)) ;
#16744=EDGE_LOOP('',(#44108,#44109,#44110,#44111)) ;
#16745=EDGE_LOOP('',(#44112,#44113,#44114,#44115)) ;
#16746=EDGE_LOOP('',(#44116,#44117,#44118,#44119)) ;
#16747=EDGE_LOOP('',(#44120,#44121,#44122,#44123)) ;
#16748=EDGE_LOOP('',(#44124,#44125,#44126,#44127)) ;
#16749=EDGE_LOOP('',(#44128,#44129,#44130,#44131)) ;
#16750=EDGE_LOOP('',(#44132,#44133,#44134,#44135)) ;
#16751=EDGE_LOOP('',(#44136,#44137,#44138,#44139)) ;
#16752=EDGE_LOOP('',(#44140,#44141,#44142,#44143)) ;
#16753=EDGE_LOOP('',(#44144,#44145,#44146,#44147)) ;
#16754=EDGE_LOOP('',(#44148,#44149,#44150,#44151)) ;
#16755=EDGE_LOOP('',(#44152,#44153,#44154,#44155)) ;
#16756=EDGE_LOOP('',(#44156,#44157,#44158,#44159)) ;
#16757=EDGE_LOOP('',(#44160,#44161,#44162,#44163)) ;
#16758=EDGE_LOOP('',(#44164,#44165,#44166,#44167)) ;
#16759=EDGE_LOOP('',(#44168,#44169,#44170,#44171)) ;
#16760=EDGE_LOOP('',(#44172,#44173,#44174,#44175)) ;
#16761=EDGE_LOOP('',(#44176,#44177,#44178,#44179)) ;
#16762=EDGE_LOOP('',(#44180,#44181,#44182,#44183)) ;
#16763=EDGE_LOOP('',(#44184,#44185,#44186,#44187)) ;
#16764=EDGE_LOOP('',(#44188,#44189,#44190,#44191)) ;
#16765=EDGE_LOOP('',(#44192,#44193,#44194,#44195)) ;
#16766=EDGE_LOOP('',(#44196,#44197,#44198,#44199)) ;
#16767=EDGE_LOOP('',(#44200,#44201,#44202,#44203)) ;
#16768=EDGE_LOOP('',(#44204,#44205,#44206,#44207)) ;
#16769=EDGE_LOOP('',(#44208,#44209,#44210,#44211)) ;
#16770=EDGE_LOOP('',(#44212,#44213,#44214,#44215)) ;
#16771=EDGE_LOOP('',(#44216,#44217,#44218,#44219)) ;
#16772=EDGE_LOOP('',(#44220,#44221,#44222,#44223)) ;
#16773=EDGE_LOOP('',(#44224,#44225,#44226,#44227)) ;
#16774=EDGE_LOOP('',(#44228,#44229,#44230,#44231)) ;
#16775=EDGE_LOOP('',(#44232,#44233,#44234,#44235)) ;
#16776=EDGE_LOOP('',(#44236,#44237,#44238,#44239)) ;
#16777=EDGE_LOOP('',(#44240,#44241,#44242,#44243)) ;
#16778=EDGE_LOOP('',(#44244,#44245,#44246,#44247)) ;
#16779=EDGE_LOOP('',(#44248,#44249,#44250,#44251)) ;
#16780=EDGE_LOOP('',(#44252,#44253,#44254,#44255)) ;
#16781=EDGE_LOOP('',(#44256,#44257,#44258,#44259)) ;
#16782=EDGE_LOOP('',(#44260,#44261,#44262,#44263)) ;
#16783=EDGE_LOOP('',(#44264,#44265,#44266,#44267)) ;
#16784=EDGE_LOOP('',(#44268,#44269,#44270,#44271)) ;
#16785=EDGE_LOOP('',(#44272,#44273,#44274,#44275)) ;
#16786=EDGE_LOOP('',(#44276,#44277,#44278,#44279)) ;
#16787=EDGE_LOOP('',(#44280,#44281,#44282,#44283)) ;
#16788=EDGE_LOOP('',(#44284,#44285,#44286,#44287)) ;
#16789=EDGE_LOOP('',(#44288,#44289,#44290,#44291)) ;
#16790=EDGE_LOOP('',(#44292,#44293,#44294,#44295)) ;
#16791=EDGE_LOOP('',(#44296,#44297,#44298,#44299)) ;
#16792=EDGE_LOOP('',(#44300,#44301,#44302,#44303)) ;
#16793=EDGE_LOOP('',(#44304,#44305,#44306,#44307)) ;
#16794=EDGE_LOOP('',(#44308,#44309,#44310,#44311)) ;
#16795=EDGE_LOOP('',(#44312,#44313,#44314,#44315)) ;
#16796=EDGE_LOOP('',(#44316,#44317,#44318,#44319)) ;
#16797=EDGE_LOOP('',(#44320,#44321,#44322,#44323)) ;
#16798=EDGE_LOOP('',(#44324,#44325,#44326,#44327)) ;
#16799=EDGE_LOOP('',(#44328,#44329,#44330,#44331)) ;
#16800=EDGE_LOOP('',(#44332,#44333,#44334,#44335)) ;
#16801=EDGE_LOOP('',(#44336,#44337,#44338,#44339)) ;
#16802=EDGE_LOOP('',(#44340,#44341,#44342,#44343)) ;
#16803=EDGE_LOOP('',(#44344,#44345,#44346,#44347)) ;
#16804=EDGE_LOOP('',(#44348,#44349,#44350,#44351)) ;
#16805=EDGE_LOOP('',(#44352,#44353,#44354,#44355)) ;
#16806=EDGE_LOOP('',(#44356,#44357,#44358,#44359)) ;
#16807=EDGE_LOOP('',(#44360,#44361,#44362,#44363)) ;
#16808=EDGE_LOOP('',(#44364,#44365,#44366,#44367)) ;
#16809=EDGE_LOOP('',(#44368,#44369,#44370,#44371)) ;
#16810=EDGE_LOOP('',(#44372,#44373,#44374,#44375)) ;
#16811=EDGE_LOOP('',(#44376,#44377,#44378,#44379)) ;
#16812=EDGE_LOOP('',(#44380,#44381,#44382,#44383)) ;
#16813=EDGE_LOOP('',(#44384,#44385,#44386,#44387)) ;
#16814=EDGE_LOOP('',(#44388,#44389,#44390,#44391)) ;
#16815=EDGE_LOOP('',(#44392,#44393,#44394,#44395)) ;
#16816=EDGE_LOOP('',(#44396,#44397,#44398,#44399)) ;
#16817=EDGE_LOOP('',(#44400,#44401,#44402,#44403)) ;
#16818=EDGE_LOOP('',(#44404,#44405,#44406,#44407)) ;
#16819=EDGE_LOOP('',(#44408,#44409,#44410,#44411)) ;
#16820=EDGE_LOOP('',(#44412,#44413,#44414,#44415)) ;
#16821=EDGE_LOOP('',(#44416,#44417,#44418,#44419)) ;
#16822=EDGE_LOOP('',(#44420,#44421,#44422,#44423)) ;
#16823=EDGE_LOOP('',(#44424,#44425,#44426,#44427)) ;
#16824=EDGE_LOOP('',(#44428,#44429,#44430,#44431)) ;
#16825=EDGE_LOOP('',(#44432,#44433,#44434,#44435)) ;
#16826=EDGE_LOOP('',(#44436,#44437,#44438,#44439)) ;
#16827=EDGE_LOOP('',(#44440,#44441,#44442,#44443)) ;
#16828=EDGE_LOOP('',(#44444,#44445,#44446,#44447)) ;
#16829=EDGE_LOOP('',(#44448,#44449,#44450,#44451)) ;
#16830=EDGE_LOOP('',(#44452,#44453,#44454,#44455)) ;
#16831=EDGE_LOOP('',(#44456,#44457,#44458,#44459)) ;
#16832=EDGE_LOOP('',(#44460,#44461,#44462,#44463)) ;
#16833=EDGE_LOOP('',(#44464,#44465,#44466,#44467)) ;
#16834=EDGE_LOOP('',(#44468,#44469,#44470,#44471)) ;
#16835=EDGE_LOOP('',(#44472,#44473,#44474,#44475)) ;
#16836=EDGE_LOOP('',(#44476,#44477,#44478,#44479)) ;
#16837=EDGE_LOOP('',(#44480,#44481,#44482,#44483)) ;
#16838=EDGE_LOOP('',(#44484,#44485,#44486,#44487)) ;
#16839=EDGE_LOOP('',(#44488,#44489,#44490,#44491)) ;
#16840=EDGE_LOOP('',(#44492,#44493,#44494,#44495)) ;
#16841=EDGE_LOOP('',(#44496,#44497,#44498,#44499)) ;
#16842=EDGE_LOOP('',(#44500,#44501,#44502,#44503)) ;
#16843=EDGE_LOOP('',(#44504,#44505,#44506,#44507)) ;
#16844=EDGE_LOOP('',(#44508,#44509,#44510,#44511)) ;
#16845=EDGE_LOOP('',(#44512,#44513,#44514,#44515)) ;
#16846=EDGE_LOOP('',(#44516,#44517,#44518,#44519)) ;
#16847=EDGE_LOOP('',(#44520,#44521,#44522,#44523)) ;
#16848=EDGE_LOOP('',(#44524,#44525,#44526,#44527)) ;
#16849=EDGE_LOOP('',(#44528,#44529,#44530,#44531)) ;
#16850=EDGE_LOOP('',(#44532,#44533,#44534,#44535)) ;
#16851=EDGE_LOOP('',(#44536,#44537,#44538,#44539)) ;
#16852=EDGE_LOOP('',(#44540,#44541,#44542,#44543)) ;
#16853=EDGE_LOOP('',(#44544,#44545,#44546,#44547)) ;
#16854=EDGE_LOOP('',(#44548,#44549,#44550,#44551)) ;
#16855=EDGE_LOOP('',(#44552,#44553,#44554,#44555)) ;
#16856=EDGE_LOOP('',(#44556,#44557,#44558,#44559)) ;
#16857=EDGE_LOOP('',(#44560,#44561,#44562,#44563)) ;
#16858=EDGE_LOOP('',(#44564,#44565,#44566,#44567)) ;
#16859=EDGE_LOOP('',(#44568,#44569,#44570,#44571)) ;
#16860=EDGE_LOOP('',(#44572,#44573,#44574,#44575)) ;
#16861=EDGE_LOOP('',(#44576,#44577,#44578,#44579)) ;
#16862=EDGE_LOOP('',(#44580,#44581,#44582,#44583)) ;
#16863=EDGE_LOOP('',(#44584,#44585,#44586,#44587,#44588)) ;
#16864=EDGE_LOOP('',(#44589,#44590,#44591,#44592,#44593,#44594,#44595,#44596,
#44597,#44598,#44599,#44600,#44601,#44602,#44603,#44604,#44605,#44606,#44607,
#44608,#44609,#44610,#44611,#44612,#44613,#44614,#44615,#44616,#44617,#44618,
#44619,#44620,#44621,#44622,#44623,#44624,#44625,#44626,#44627,#44628,#44629,
#44630,#44631,#44632,#44633)) ;
#16865=EDGE_LOOP('',(#44634,#44635,#44636,#44637)) ;
#16866=EDGE_LOOP('',(#44638,#44639,#44640,#44641,#44642,#44643,#44644,#44645,
#44646,#44647,#44648,#44649,#44650,#44651,#44652,#44653,#44654,#44655,#44656,
#44657,#44658,#44659,#44660,#44661,#44662,#44663,#44664,#44665,#44666,#44667,
#44668,#44669,#44670,#44671,#44672,#44673,#44674,#44675,#44676,#44677,#44678,
#44679,#44680,#44681,#44682)) ;
#16867=EDGE_LOOP('',(#44683,#44684,#44685,#44686)) ;
#16868=EDGE_LOOP('',(#44687,#44688,#44689,#44690)) ;
#16869=EDGE_LOOP('',(#44691,#44692,#44693,#44694)) ;
#16870=EDGE_LOOP('',(#44695,#44696,#44697,#44698)) ;
#16871=EDGE_LOOP('',(#44699,#44700,#44701,#44702)) ;
#16872=EDGE_LOOP('',(#44703,#44704,#44705,#44706)) ;
#16873=EDGE_LOOP('',(#44707,#44708,#44709,#44710)) ;
#16874=EDGE_LOOP('',(#44711,#44712,#44713,#44714)) ;
#16875=EDGE_LOOP('',(#44715,#44716,#44717,#44718)) ;
#16876=EDGE_LOOP('',(#44719,#44720,#44721,#44722)) ;
#16877=EDGE_LOOP('',(#44723,#44724,#44725,#44726)) ;
#16878=EDGE_LOOP('',(#44727,#44728,#44729,#44730)) ;
#16879=EDGE_LOOP('',(#44731,#44732,#44733,#44734)) ;
#16880=EDGE_LOOP('',(#44735,#44736,#44737,#44738)) ;
#16881=EDGE_LOOP('',(#44739,#44740,#44741,#44742)) ;
#16882=EDGE_LOOP('',(#44743,#44744,#44745,#44746)) ;
#16883=EDGE_LOOP('',(#44747,#44748,#44749,#44750)) ;
#16884=EDGE_LOOP('',(#44751,#44752,#44753,#44754)) ;
#16885=EDGE_LOOP('',(#44755,#44756,#44757,#44758)) ;
#16886=EDGE_LOOP('',(#44759,#44760,#44761,#44762,#44763)) ;
#16887=EDGE_LOOP('',(#44764,#44765,#44766,#44767)) ;
#16888=EDGE_LOOP('',(#44768,#44769,#44770,#44771)) ;
#16889=EDGE_LOOP('',(#44772,#44773,#44774,#44775)) ;
#16890=EDGE_LOOP('',(#44776,#44777,#44778,#44779)) ;
#16891=EDGE_LOOP('',(#44780,#44781,#44782,#44783)) ;
#16892=EDGE_LOOP('',(#44784,#44785,#44786,#44787)) ;
#16893=EDGE_LOOP('',(#44788,#44789,#44790,#44791)) ;
#16894=EDGE_LOOP('',(#44792,#44793,#44794,#44795)) ;
#16895=EDGE_LOOP('',(#44796,#44797,#44798,#44799)) ;
#16896=EDGE_LOOP('',(#44800,#44801,#44802,#44803)) ;
#16897=EDGE_LOOP('',(#44804,#44805,#44806,#44807)) ;
#16898=EDGE_LOOP('',(#44808,#44809,#44810,#44811)) ;
#16899=EDGE_LOOP('',(#44812,#44813,#44814,#44815)) ;
#16900=EDGE_LOOP('',(#44816,#44817,#44818,#44819)) ;
#16901=EDGE_LOOP('',(#44820,#44821,#44822,#44823)) ;
#16902=EDGE_LOOP('',(#44824,#44825,#44826,#44827)) ;
#16903=EDGE_LOOP('',(#44828,#44829,#44830,#44831)) ;
#16904=EDGE_LOOP('',(#44832,#44833,#44834,#44835)) ;
#16905=EDGE_LOOP('',(#44836,#44837,#44838,#44839)) ;
#16906=EDGE_LOOP('',(#44840,#44841,#44842,#44843)) ;
#16907=EDGE_LOOP('',(#44844,#44845,#44846,#44847)) ;
#16908=EDGE_LOOP('',(#44848,#44849,#44850,#44851)) ;
#16909=EDGE_LOOP('',(#44852,#44853,#44854,#44855)) ;
#16910=EDGE_LOOP('',(#44856,#44857,#44858,#44859)) ;
#16911=EDGE_LOOP('',(#44860,#44861,#44862,#44863)) ;
#16912=EDGE_LOOP('',(#44864,#44865,#44866,#44867)) ;
#16913=EDGE_LOOP('',(#44868,#44869,#44870,#44871)) ;
#16914=EDGE_LOOP('',(#44872,#44873,#44874,#44875)) ;
#16915=EDGE_LOOP('',(#44876,#44877,#44878,#44879)) ;
#16916=EDGE_LOOP('',(#44880,#44881,#44882,#44883)) ;
#16917=EDGE_LOOP('',(#44884,#44885,#44886,#44887)) ;
#16918=EDGE_LOOP('',(#44888,#44889,#44890,#44891)) ;
#16919=EDGE_LOOP('',(#44892,#44893,#44894,#44895)) ;
#16920=EDGE_LOOP('',(#44896,#44897,#44898,#44899)) ;
#16921=EDGE_LOOP('',(#44900,#44901,#44902,#44903)) ;
#16922=EDGE_LOOP('',(#44904,#44905,#44906,#44907)) ;
#16923=EDGE_LOOP('',(#44908,#44909,#44910,#44911)) ;
#16924=EDGE_LOOP('',(#44912,#44913,#44914,#44915)) ;
#16925=EDGE_LOOP('',(#44916,#44917,#44918,#44919)) ;
#16926=EDGE_LOOP('',(#44920,#44921,#44922,#44923)) ;
#16927=EDGE_LOOP('',(#44924,#44925,#44926,#44927)) ;
#16928=EDGE_LOOP('',(#44928,#44929,#44930,#44931)) ;
#16929=EDGE_LOOP('',(#44932,#44933,#44934,#44935)) ;
#16930=EDGE_LOOP('',(#44936,#44937,#44938,#44939)) ;
#16931=EDGE_LOOP('',(#44940,#44941,#44942,#44943)) ;
#16932=EDGE_LOOP('',(#44944,#44945,#44946,#44947)) ;
#16933=EDGE_LOOP('',(#44948,#44949,#44950,#44951)) ;
#16934=EDGE_LOOP('',(#44952,#44953,#44954,#44955)) ;
#16935=EDGE_LOOP('',(#44956,#44957,#44958,#44959)) ;
#16936=EDGE_LOOP('',(#44960,#44961,#44962,#44963)) ;
#16937=EDGE_LOOP('',(#44964,#44965,#44966,#44967)) ;
#16938=EDGE_LOOP('',(#44968,#44969,#44970,#44971)) ;
#16939=EDGE_LOOP('',(#44972,#44973,#44974,#44975)) ;
#16940=EDGE_LOOP('',(#44976,#44977,#44978,#44979)) ;
#16941=EDGE_LOOP('',(#44980,#44981,#44982,#44983)) ;
#16942=EDGE_LOOP('',(#44984,#44985,#44986,#44987)) ;
#16943=EDGE_LOOP('',(#44988,#44989,#44990,#44991)) ;
#16944=EDGE_LOOP('',(#44992,#44993,#44994,#44995)) ;
#16945=EDGE_LOOP('',(#44996,#44997,#44998,#44999)) ;
#16946=EDGE_LOOP('',(#45000,#45001,#45002,#45003)) ;
#16947=EDGE_LOOP('',(#45004,#45005,#45006,#45007)) ;
#16948=EDGE_LOOP('',(#45008,#45009,#45010,#45011)) ;
#16949=EDGE_LOOP('',(#45012,#45013,#45014,#45015)) ;
#16950=EDGE_LOOP('',(#45016,#45017,#45018,#45019)) ;
#16951=EDGE_LOOP('',(#45020,#45021,#45022,#45023)) ;
#16952=EDGE_LOOP('',(#45024,#45025,#45026,#45027)) ;
#16953=EDGE_LOOP('',(#45028,#45029,#45030,#45031)) ;
#16954=EDGE_LOOP('',(#45032,#45033,#45034,#45035)) ;
#16955=EDGE_LOOP('',(#45036,#45037,#45038,#45039)) ;
#16956=EDGE_LOOP('',(#45040,#45041,#45042,#45043)) ;
#16957=EDGE_LOOP('',(#45044,#45045,#45046,#45047)) ;
#16958=EDGE_LOOP('',(#45048,#45049,#45050,#45051)) ;
#16959=EDGE_LOOP('',(#45052,#45053,#45054,#45055)) ;
#16960=EDGE_LOOP('',(#45056,#45057,#45058,#45059)) ;
#16961=EDGE_LOOP('',(#45060,#45061,#45062,#45063)) ;
#16962=EDGE_LOOP('',(#45064,#45065,#45066,#45067)) ;
#16963=EDGE_LOOP('',(#45068,#45069,#45070,#45071)) ;
#16964=EDGE_LOOP('',(#45072,#45073,#45074,#45075)) ;
#16965=EDGE_LOOP('',(#45076,#45077,#45078,#45079)) ;
#16966=EDGE_LOOP('',(#45080,#45081,#45082,#45083)) ;
#16967=EDGE_LOOP('',(#45084,#45085,#45086,#45087)) ;
#16968=EDGE_LOOP('',(#45088,#45089,#45090,#45091)) ;
#16969=EDGE_LOOP('',(#45092,#45093,#45094,#45095)) ;
#16970=EDGE_LOOP('',(#45096,#45097,#45098,#45099)) ;
#16971=EDGE_LOOP('',(#45100,#45101,#45102,#45103)) ;
#16972=EDGE_LOOP('',(#45104,#45105,#45106,#45107)) ;
#16973=EDGE_LOOP('',(#45108,#45109,#45110,#45111)) ;
#16974=EDGE_LOOP('',(#45112,#45113,#45114,#45115)) ;
#16975=EDGE_LOOP('',(#45116,#45117,#45118,#45119)) ;
#16976=EDGE_LOOP('',(#45120,#45121,#45122,#45123)) ;
#16977=EDGE_LOOP('',(#45124,#45125,#45126,#45127)) ;
#16978=EDGE_LOOP('',(#45128,#45129,#45130,#45131)) ;
#16979=EDGE_LOOP('',(#45132,#45133,#45134,#45135)) ;
#16980=EDGE_LOOP('',(#45136,#45137,#45138,#45139)) ;
#16981=EDGE_LOOP('',(#45140,#45141,#45142,#45143)) ;
#16982=EDGE_LOOP('',(#45144,#45145,#45146,#45147)) ;
#16983=EDGE_LOOP('',(#45148,#45149,#45150,#45151)) ;
#16984=EDGE_LOOP('',(#45152,#45153,#45154,#45155)) ;
#16985=EDGE_LOOP('',(#45156,#45157,#45158,#45159)) ;
#16986=EDGE_LOOP('',(#45160,#45161,#45162,#45163)) ;
#16987=EDGE_LOOP('',(#45164,#45165,#45166,#45167)) ;
#16988=EDGE_LOOP('',(#45168,#45169,#45170,#45171)) ;
#16989=EDGE_LOOP('',(#45172,#45173,#45174,#45175)) ;
#16990=EDGE_LOOP('',(#45176,#45177,#45178,#45179)) ;
#16991=EDGE_LOOP('',(#45180,#45181,#45182,#45183)) ;
#16992=EDGE_LOOP('',(#45184,#45185,#45186,#45187)) ;
#16993=EDGE_LOOP('',(#45188,#45189,#45190,#45191)) ;
#16994=EDGE_LOOP('',(#45192,#45193,#45194,#45195)) ;
#16995=EDGE_LOOP('',(#45196,#45197,#45198,#45199)) ;
#16996=EDGE_LOOP('',(#45200,#45201,#45202,#45203)) ;
#16997=EDGE_LOOP('',(#45204,#45205,#45206,#45207)) ;
#16998=EDGE_LOOP('',(#45208,#45209,#45210,#45211)) ;
#16999=EDGE_LOOP('',(#45212,#45213,#45214,#45215)) ;
#17000=EDGE_LOOP('',(#45216,#45217,#45218,#45219)) ;
#17001=EDGE_LOOP('',(#45220,#45221,#45222,#45223)) ;
#17002=EDGE_LOOP('',(#45224,#45225,#45226,#45227)) ;
#17003=EDGE_LOOP('',(#45228,#45229,#45230,#45231)) ;
#17004=EDGE_LOOP('',(#45232,#45233,#45234,#45235)) ;
#17005=EDGE_LOOP('',(#45236,#45237,#45238,#45239)) ;
#17006=EDGE_LOOP('',(#45240,#45241,#45242,#45243)) ;
#17007=EDGE_LOOP('',(#45244,#45245,#45246,#45247)) ;
#19339=CIRCLE('',#54546,3.) ;
#19340=CIRCLE('',#54547,1.) ;
#19341=CIRCLE('',#54548,3.96824583655185) ;
#19342=CIRCLE('',#54551,4.) ;
#19343=CIRCLE('',#54552,1.) ;
#19344=CIRCLE('',#54553,3.) ;
#19345=CIRCLE('',#54556,2.) ;
#19346=CIRCLE('',#54558,2.) ;
#19347=CIRCLE('',#54560,4.95) ;
#19348=CIRCLE('',#54561,5.1) ;
#19349=CIRCLE('',#54564,0.350000000000003) ;
#19350=CIRCLE('',#54565,0.500000000000003) ;
#19351=CIRCLE('',#54568,4.95) ;
#19352=CIRCLE('',#54569,5.1) ;
#19353=CIRCLE('',#54572,0.350000000000003) ;
#19354=CIRCLE('',#54573,0.500000000000003) ;
#19355=CIRCLE('',#54576,4.95) ;
#19356=CIRCLE('',#54577,5.1) ;
#19357=CIRCLE('',#54580,0.350000000000003) ;
#19358=CIRCLE('',#54581,0.500000000000003) ;
#19359=CIRCLE('',#54584,4.95) ;
#19360=CIRCLE('',#54585,5.1) ;
#19361=CIRCLE('',#54588,0.350000000000003) ;
#19362=CIRCLE('',#54589,0.500000000000003) ;
#19363=CIRCLE('',#54592,4.95) ;
#19364=CIRCLE('',#54593,5.1) ;
#19365=CIRCLE('',#54596,0.350000000000003) ;
#19366=CIRCLE('',#54597,0.500000000000003) ;
#19367=CIRCLE('',#54600,4.95) ;
#19368=CIRCLE('',#54601,5.1) ;
#19369=CIRCLE('',#54604,0.350000000000003) ;
#19370=CIRCLE('',#54605,0.500000000000003) ;
#19371=CIRCLE('',#54608,4.95) ;
#19372=CIRCLE('',#54609,5.1) ;
#19373=CIRCLE('',#54612,0.350000000000003) ;
#19374=CIRCLE('',#54613,0.500000000000003) ;
#19375=CIRCLE('',#54616,4.95) ;
#19376=CIRCLE('',#54617,5.1) ;
#19377=CIRCLE('',#54620,0.350000000000003) ;
#19378=CIRCLE('',#54621,0.500000000000003) ;
#19379=CIRCLE('',#54624,4.95) ;
#19380=CIRCLE('',#54625,5.1) ;
#19381=CIRCLE('',#54628,0.350000000000003) ;
#19382=CIRCLE('',#54629,0.500000000000003) ;
#19383=CIRCLE('',#54632,4.95) ;
#19384=CIRCLE('',#54633,5.1) ;
#19385=CIRCLE('',#54636,0.350000000000003) ;
#19386=CIRCLE('',#54637,0.500000000000003) ;
#19387=CIRCLE('',#54640,4.95) ;
#19388=CIRCLE('',#54641,5.1) ;
#19389=CIRCLE('',#54644,0.500000000000003) ;
#19390=CIRCLE('',#54645,0.350000000000003) ;
#19391=CIRCLE('',#54648,5.1) ;
#19392=CIRCLE('',#54649,4.95) ;
#19393=CIRCLE('',#54652,0.500000000000003) ;
#19394=CIRCLE('',#54653,0.350000000000003) ;
#19395=CIRCLE('',#54656,5.1) ;
#19396=CIRCLE('',#54657,4.95) ;
#19397=CIRCLE('',#54660,0.500000000000003) ;
#19398=CIRCLE('',#54661,0.350000000000003) ;
#19399=CIRCLE('',#54664,5.1) ;
#19400=CIRCLE('',#54665,4.95) ;
#19401=CIRCLE('',#54668,0.500000000000003) ;
#19402=CIRCLE('',#54669,0.350000000000003) ;
#19403=CIRCLE('',#54672,5.1) ;
#19404=CIRCLE('',#54673,4.95) ;
#19405=CIRCLE('',#54676,0.500000000000003) ;
#19406=CIRCLE('',#54677,0.350000000000003) ;
#19407=CIRCLE('',#54680,5.1) ;
#19408=CIRCLE('',#54681,4.95) ;
#19409=CIRCLE('',#54684,0.500000000000003) ;
#19410=CIRCLE('',#54685,0.350000000000003) ;
#19411=CIRCLE('',#54688,5.1) ;
#19412=CIRCLE('',#54689,4.95) ;
#19413=CIRCLE('',#54692,0.500000000000003) ;
#19414=CIRCLE('',#54693,0.350000000000003) ;
#19415=CIRCLE('',#54696,5.1) ;
#19416=CIRCLE('',#54697,4.95) ;
#19417=CIRCLE('',#54700,0.500000000000003) ;
#19418=CIRCLE('',#54701,0.350000000000003) ;
#19419=CIRCLE('',#54704,5.1) ;
#19420=CIRCLE('',#54705,4.95) ;
#19421=CIRCLE('',#54708,0.500000000000003) ;
#19422=CIRCLE('',#54709,0.350000000000003) ;
#19423=CIRCLE('',#54712,5.1) ;
#19424=CIRCLE('',#54713,4.95) ;
#19425=CIRCLE('',#54716,0.500000000000003) ;
#19426=CIRCLE('',#54717,0.350000000000003) ;
#19427=CIRCLE('',#54721,0.500000000000003) ;
#19428=CIRCLE('',#54724,5.1) ;
#19429=CIRCLE('',#54727,0.500000000000003) ;
#19430=CIRCLE('',#54730,5.1) ;
#19431=CIRCLE('',#54733,0.500000000000003) ;
#19432=CIRCLE('',#54736,5.1) ;
#19433=CIRCLE('',#54739,0.500000000000003) ;
#19434=CIRCLE('',#54742,5.1) ;
#19435=CIRCLE('',#54745,0.500000000000003) ;
#19436=CIRCLE('',#54748,5.1) ;
#19437=CIRCLE('',#54751,0.500000000000003) ;
#19438=CIRCLE('',#54754,5.1) ;
#19439=CIRCLE('',#54757,0.500000000000003) ;
#19440=CIRCLE('',#54760,5.1) ;
#19441=CIRCLE('',#54763,0.500000000000003) ;
#19442=CIRCLE('',#54766,5.1) ;
#19443=CIRCLE('',#54769,0.500000000000003) ;
#19444=CIRCLE('',#54772,5.1) ;
#19445=CIRCLE('',#54775,0.500000000000003) ;
#19446=CIRCLE('',#54778,5.1) ;
#19447=CIRCLE('',#54780,4.95) ;
#19448=CIRCLE('',#54782,4.95) ;
#19449=CIRCLE('',#54784,4.95) ;
#19450=CIRCLE('',#54786,4.95) ;
#19451=CIRCLE('',#54788,4.95) ;
#19452=CIRCLE('',#54790,4.95) ;
#19453=CIRCLE('',#54792,4.95) ;
#19454=CIRCLE('',#54794,4.95) ;
#19455=CIRCLE('',#54796,4.95) ;
#19456=CIRCLE('',#54798,4.95) ;
#19457=CIRCLE('',#54800,4.95) ;
#19458=CIRCLE('',#54802,4.95) ;
#19459=CIRCLE('',#54804,4.95) ;
#19460=CIRCLE('',#54806,4.95) ;
#19461=CIRCLE('',#54808,4.95) ;
#19462=CIRCLE('',#54810,4.95) ;
#19463=CIRCLE('',#54812,4.95) ;
#19464=CIRCLE('',#54814,4.95) ;
#19465=CIRCLE('',#54816,4.95) ;
#19466=CIRCLE('',#54817,4.95) ;
#19467=CIRCLE('',#54819,0.15) ;
#19468=CIRCLE('',#54820,4.95) ;
#19469=CIRCLE('',#54823,0.15) ;
#19470=CIRCLE('',#54824,4.95) ;
#19471=CIRCLE('',#54825,4.95) ;
#19472=CIRCLE('',#54826,4.95) ;
#19473=CIRCLE('',#54827,4.95) ;
#19474=CIRCLE('',#54828,4.95) ;
#19475=CIRCLE('',#54829,4.95) ;
#19476=CIRCLE('',#54830,4.95) ;
#19477=CIRCLE('',#54831,4.95) ;
#19478=CIRCLE('',#54832,4.95) ;
#19479=CIRCLE('',#54833,4.95) ;
#19480=CIRCLE('',#54834,4.95) ;
#19481=CIRCLE('',#54835,4.95) ;
#19482=CIRCLE('',#54836,4.95) ;
#19483=CIRCLE('',#54837,4.95) ;
#19484=CIRCLE('',#54838,4.95) ;
#19485=CIRCLE('',#54839,4.95) ;
#19486=CIRCLE('',#54840,4.95) ;
#19487=CIRCLE('',#54841,4.95) ;
#19488=CIRCLE('',#54842,4.95) ;
#19489=CIRCLE('',#54843,4.95) ;
#19490=CIRCLE('',#54844,4.95) ;
#19491=CIRCLE('',#54845,4.95) ;
#19492=CIRCLE('',#54846,4.95) ;
#19493=CIRCLE('',#54847,4.95) ;
#19494=CIRCLE('',#54848,4.95) ;
#19495=CIRCLE('',#54849,4.95) ;
#19496=CIRCLE('',#54850,4.95) ;
#19497=CIRCLE('',#54851,4.95) ;
#19498=CIRCLE('',#54852,4.95) ;
#19499=CIRCLE('',#54853,4.95) ;
#19500=CIRCLE('',#54854,4.95) ;
#19501=CIRCLE('',#54855,4.95) ;
#19502=CIRCLE('',#54856,4.95) ;
#19503=CIRCLE('',#54857,4.95) ;
#19504=CIRCLE('',#54858,4.95) ;
#19505=CIRCLE('',#54859,4.95) ;
#19506=CIRCLE('',#54860,4.95) ;
#19507=CIRCLE('',#54861,4.95) ;
#19508=CIRCLE('',#54862,4.95) ;
#19509=CIRCLE('',#54863,4.95) ;
#19510=CIRCLE('',#54864,4.95) ;
#19511=CIRCLE('',#54866,0.350000000000003) ;
#19512=CIRCLE('',#54868,0.350000000000003) ;
#19513=CIRCLE('',#54870,0.350000000000003) ;
#19514=CIRCLE('',#54872,0.350000000000003) ;
#19515=CIRCLE('',#54874,0.350000000000003) ;
#19516=CIRCLE('',#54876,0.350000000000003) ;
#19517=CIRCLE('',#54878,0.350000000000003) ;
#19518=CIRCLE('',#54880,0.350000000000003) ;
#19519=CIRCLE('',#54882,0.350000000000003) ;
#19520=CIRCLE('',#54884,0.350000000000003) ;
#19521=CIRCLE('',#54886,0.350000000000003) ;
#19522=CIRCLE('',#54888,0.350000000000003) ;
#19523=CIRCLE('',#54890,0.350000000000003) ;
#19524=CIRCLE('',#54892,0.350000000000003) ;
#19525=CIRCLE('',#54894,0.350000000000003) ;
#19526=CIRCLE('',#54896,0.350000000000003) ;
#19527=CIRCLE('',#54898,0.350000000000003) ;
#19528=CIRCLE('',#54900,0.350000000000003) ;
#19529=CIRCLE('',#54902,0.350000000000003) ;
#19530=CIRCLE('',#54904,0.350000000000003) ;
#19531=CIRCLE('',#54906,5.1) ;
#19532=CIRCLE('',#54951,5.1) ;
#19533=CIRCLE('',#54954,0.500000000000003) ;
#19534=CIRCLE('',#54957,5.1) ;
#19535=CIRCLE('',#54960,0.500000000000003) ;
#19536=CIRCLE('',#54963,5.1) ;
#19537=CIRCLE('',#54966,0.500000000000003) ;
#19538=CIRCLE('',#54969,5.1) ;
#19539=CIRCLE('',#54972,0.500000000000003) ;
#19540=CIRCLE('',#54975,5.1) ;
#19541=CIRCLE('',#54978,0.500000000000003) ;
#19542=CIRCLE('',#54981,5.1) ;
#19543=CIRCLE('',#54984,0.500000000000003) ;
#19544=CIRCLE('',#54987,5.1) ;
#19545=CIRCLE('',#54990,0.500000000000003) ;
#19546=CIRCLE('',#54993,5.1) ;
#19547=CIRCLE('',#54996,0.500000000000003) ;
#19548=CIRCLE('',#54999,5.1) ;
#19549=CIRCLE('',#55002,0.500000000000003) ;
#19550=CIRCLE('',#55004,0.500000000000003) ;
#23367=VERTEX_POINT('',#105466) ;
#23368=VERTEX_POINT('',#105468) ;
#23369=VERTEX_POINT('',#105472) ;
#23370=VERTEX_POINT('',#105491) ;
#23371=VERTEX_POINT('',#105493) ;
#23372=VERTEX_POINT('',#105497) ;
#23373=VERTEX_POINT('',#105516) ;
#23374=VERTEX_POINT('',#105519) ;
#23375=VERTEX_POINT('',#105606) ;
#23376=VERTEX_POINT('',#105612) ;
#23377=VERTEX_POINT('',#105719) ;
#23378=VERTEX_POINT('',#105725) ;
#23379=VERTEX_POINT('',#105748) ;
#23380=VERTEX_POINT('',#105749) ;
#23381=VERTEX_POINT('',#105751) ;
#23382=VERTEX_POINT('',#105766) ;
#23383=VERTEX_POINT('',#105783) ;
#23384=VERTEX_POINT('',#105785) ;
#23385=VERTEX_POINT('',#105804) ;
#23386=VERTEX_POINT('',#105806) ;
#23387=VERTEX_POINT('',#105825) ;
#23388=VERTEX_POINT('',#105827) ;
#23389=VERTEX_POINT('',#105844) ;
#23390=VERTEX_POINT('',#105846) ;
#23391=VERTEX_POINT('',#105863) ;
#23392=VERTEX_POINT('',#105865) ;
#23393=VERTEX_POINT('',#105884) ;
#23394=VERTEX_POINT('',#105886) ;
#23395=VERTEX_POINT('',#105905) ;
#23396=VERTEX_POINT('',#105907) ;
#23397=VERTEX_POINT('',#105924) ;
#23398=VERTEX_POINT('',#105926) ;
#23399=VERTEX_POINT('',#105943) ;
#23400=VERTEX_POINT('',#105945) ;
#23401=VERTEX_POINT('',#105964) ;
#23402=VERTEX_POINT('',#105966) ;
#23403=VERTEX_POINT('',#105985) ;
#23404=VERTEX_POINT('',#105987) ;
#23405=VERTEX_POINT('',#106004) ;
#23406=VERTEX_POINT('',#106006) ;
#23407=VERTEX_POINT('',#106023) ;
#23408=VERTEX_POINT('',#106025) ;
#23409=VERTEX_POINT('',#106044) ;
#23410=VERTEX_POINT('',#106046) ;
#23411=VERTEX_POINT('',#106065) ;
#23412=VERTEX_POINT('',#106067) ;
#23413=VERTEX_POINT('',#106084) ;
#23414=VERTEX_POINT('',#106086) ;
#23415=VERTEX_POINT('',#106103) ;
#23416=VERTEX_POINT('',#106105) ;
#23417=VERTEX_POINT('',#106124) ;
#23418=VERTEX_POINT('',#106126) ;
#23419=VERTEX_POINT('',#106145) ;
#23420=VERTEX_POINT('',#106147) ;
#23421=VERTEX_POINT('',#106164) ;
#23422=VERTEX_POINT('',#106166) ;
#23423=VERTEX_POINT('',#106183) ;
#23424=VERTEX_POINT('',#106185) ;
#23425=VERTEX_POINT('',#106204) ;
#23426=VERTEX_POINT('',#106206) ;
#23427=VERTEX_POINT('',#106225) ;
#23428=VERTEX_POINT('',#106227) ;
#23429=VERTEX_POINT('',#106244) ;
#23430=VERTEX_POINT('',#106246) ;
#23431=VERTEX_POINT('',#106263) ;
#23432=VERTEX_POINT('',#106265) ;
#23433=VERTEX_POINT('',#106284) ;
#23434=VERTEX_POINT('',#106286) ;
#23435=VERTEX_POINT('',#106305) ;
#23436=VERTEX_POINT('',#106307) ;
#23437=VERTEX_POINT('',#106324) ;
#23438=VERTEX_POINT('',#106326) ;
#23439=VERTEX_POINT('',#106343) ;
#23440=VERTEX_POINT('',#106345) ;
#23441=VERTEX_POINT('',#106364) ;
#23442=VERTEX_POINT('',#106366) ;
#23443=VERTEX_POINT('',#106385) ;
#23444=VERTEX_POINT('',#106387) ;
#23445=VERTEX_POINT('',#106404) ;
#23446=VERTEX_POINT('',#106406) ;
#23447=VERTEX_POINT('',#106423) ;
#23448=VERTEX_POINT('',#106425) ;
#23449=VERTEX_POINT('',#106444) ;
#23450=VERTEX_POINT('',#106446) ;
#23451=VERTEX_POINT('',#106465) ;
#23452=VERTEX_POINT('',#106467) ;
#23453=VERTEX_POINT('',#106484) ;
#23454=VERTEX_POINT('',#106486) ;
#23455=VERTEX_POINT('',#106503) ;
#23456=VERTEX_POINT('',#106505) ;
#23457=VERTEX_POINT('',#106524) ;
#23458=VERTEX_POINT('',#106526) ;
#23459=VERTEX_POINT('',#106545) ;
#23460=VERTEX_POINT('',#106547) ;
#23461=VERTEX_POINT('',#106564) ;
#23462=VERTEX_POINT('',#106566) ;
#23463=VERTEX_POINT('',#106583) ;
#23464=VERTEX_POINT('',#106585) ;
#23465=VERTEX_POINT('',#106604) ;
#23466=VERTEX_POINT('',#106606) ;
#23467=VERTEX_POINT('',#106625) ;
#23468=VERTEX_POINT('',#106627) ;
#23469=VERTEX_POINT('',#106644) ;
#23470=VERTEX_POINT('',#106646) ;
#23471=VERTEX_POINT('',#106663) ;
#23472=VERTEX_POINT('',#106665) ;
#23473=VERTEX_POINT('',#106684) ;
#23474=VERTEX_POINT('',#106686) ;
#23475=VERTEX_POINT('',#106705) ;
#23476=VERTEX_POINT('',#106707) ;
#23477=VERTEX_POINT('',#106724) ;
#23478=VERTEX_POINT('',#106726) ;
#23479=VERTEX_POINT('',#106743) ;
#23480=VERTEX_POINT('',#106745) ;
#23481=VERTEX_POINT('',#106764) ;
#23482=VERTEX_POINT('',#106766) ;
#23483=VERTEX_POINT('',#106785) ;
#23484=VERTEX_POINT('',#106787) ;
#23485=VERTEX_POINT('',#106804) ;
#23486=VERTEX_POINT('',#106806) ;
#23487=VERTEX_POINT('',#106823) ;
#23488=VERTEX_POINT('',#106825) ;
#23489=VERTEX_POINT('',#106844) ;
#23490=VERTEX_POINT('',#106846) ;
#23491=VERTEX_POINT('',#106865) ;
#23492=VERTEX_POINT('',#106867) ;
#23493=VERTEX_POINT('',#106884) ;
#23494=VERTEX_POINT('',#106886) ;
#23495=VERTEX_POINT('',#106903) ;
#23496=VERTEX_POINT('',#106905) ;
#23497=VERTEX_POINT('',#106924) ;
#23498=VERTEX_POINT('',#106926) ;
#23499=VERTEX_POINT('',#106945) ;
#23500=VERTEX_POINT('',#106947) ;
#23501=VERTEX_POINT('',#106964) ;
#23502=VERTEX_POINT('',#106966) ;
#23503=VERTEX_POINT('',#106983) ;
#23504=VERTEX_POINT('',#106985) ;
#23505=VERTEX_POINT('',#107004) ;
#23506=VERTEX_POINT('',#107006) ;
#23507=VERTEX_POINT('',#107025) ;
#23508=VERTEX_POINT('',#107027) ;
#23509=VERTEX_POINT('',#107044) ;
#23510=VERTEX_POINT('',#107046) ;
#23511=VERTEX_POINT('',#107063) ;
#23512=VERTEX_POINT('',#107065) ;
#23513=VERTEX_POINT('',#107084) ;
#23514=VERTEX_POINT('',#107086) ;
#23515=VERTEX_POINT('',#107105) ;
#23516=VERTEX_POINT('',#107107) ;
#23517=VERTEX_POINT('',#107124) ;
#23518=VERTEX_POINT('',#107126) ;
#23519=VERTEX_POINT('',#107143) ;
#23520=VERTEX_POINT('',#107145) ;
#23521=VERTEX_POINT('',#107164) ;
#23522=VERTEX_POINT('',#107166) ;
#23523=VERTEX_POINT('',#107185) ;
#23524=VERTEX_POINT('',#107187) ;
#23525=VERTEX_POINT('',#107204) ;
#23526=VERTEX_POINT('',#107206) ;
#23527=VERTEX_POINT('',#107223) ;
#23528=VERTEX_POINT('',#107225) ;
#23529=VERTEX_POINT('',#107244) ;
#23530=VERTEX_POINT('',#107246) ;
#23531=VERTEX_POINT('',#107265) ;
#23532=VERTEX_POINT('',#107267) ;
#23533=VERTEX_POINT('',#107284) ;
#23534=VERTEX_POINT('',#107286) ;
#23535=VERTEX_POINT('',#107303) ;
#23536=VERTEX_POINT('',#107305) ;
#23537=VERTEX_POINT('',#107324) ;
#23538=VERTEX_POINT('',#107326) ;
#23539=VERTEX_POINT('',#107348) ;
#23540=VERTEX_POINT('',#107350) ;
#23541=VERTEX_POINT('',#107354) ;
#23542=VERTEX_POINT('',#107358) ;
#23543=VERTEX_POINT('',#107362) ;
#23544=VERTEX_POINT('',#107366) ;
#23545=VERTEX_POINT('',#107370) ;
#23546=VERTEX_POINT('',#107374) ;
#23547=VERTEX_POINT('',#107378) ;
#23548=VERTEX_POINT('',#107382) ;
#23549=VERTEX_POINT('',#107386) ;
#23550=VERTEX_POINT('',#107390) ;
#23551=VERTEX_POINT('',#107394) ;
#23552=VERTEX_POINT('',#107398) ;
#23553=VERTEX_POINT('',#107402) ;
#23554=VERTEX_POINT('',#107406) ;
#23555=VERTEX_POINT('',#107410) ;
#23556=VERTEX_POINT('',#107414) ;
#23557=VERTEX_POINT('',#107418) ;
#23558=VERTEX_POINT('',#107422) ;
#23559=VERTEX_POINT('',#107426) ;
#23560=VERTEX_POINT('',#107430) ;
#23561=VERTEX_POINT('',#107434) ;
#23562=VERTEX_POINT('',#107438) ;
#23563=VERTEX_POINT('',#107442) ;
#23564=VERTEX_POINT('',#107446) ;
#23565=VERTEX_POINT('',#107450) ;
#23566=VERTEX_POINT('',#107454) ;
#23567=VERTEX_POINT('',#107458) ;
#23568=VERTEX_POINT('',#107462) ;
#23569=VERTEX_POINT('',#107466) ;
#23570=VERTEX_POINT('',#107470) ;
#23571=VERTEX_POINT('',#107474) ;
#23572=VERTEX_POINT('',#107478) ;
#23573=VERTEX_POINT('',#107482) ;
#23574=VERTEX_POINT('',#107486) ;
#23575=VERTEX_POINT('',#107490) ;
#23576=VERTEX_POINT('',#107494) ;
#23577=VERTEX_POINT('',#107498) ;
#23578=VERTEX_POINT('',#107502) ;
#23579=VERTEX_POINT('',#107506) ;
#23580=VERTEX_POINT('',#107546) ;
#23581=VERTEX_POINT('',#107554) ;
#23582=VERTEX_POINT('',#107556) ;
#23583=VERTEX_POINT('',#107558) ;
#23584=VERTEX_POINT('',#107560) ;
#23585=VERTEX_POINT('',#107562) ;
#23586=VERTEX_POINT('',#107564) ;
#23587=VERTEX_POINT('',#107566) ;
#23588=VERTEX_POINT('',#107568) ;
#23589=VERTEX_POINT('',#107570) ;
#23590=VERTEX_POINT('',#107572) ;
#23591=VERTEX_POINT('',#107574) ;
#23592=VERTEX_POINT('',#107576) ;
#23593=VERTEX_POINT('',#107578) ;
#23594=VERTEX_POINT('',#107580) ;
#23595=VERTEX_POINT('',#107582) ;
#23596=VERTEX_POINT('',#107584) ;
#23597=VERTEX_POINT('',#107586) ;
#23598=VERTEX_POINT('',#107588) ;
#23599=VERTEX_POINT('',#107590) ;
#23600=VERTEX_POINT('',#107592) ;
#23601=VERTEX_POINT('',#107594) ;
#23602=VERTEX_POINT('',#107596) ;
#23603=VERTEX_POINT('',#107598) ;
#23604=VERTEX_POINT('',#107600) ;
#23605=VERTEX_POINT('',#107602) ;
#23606=VERTEX_POINT('',#107604) ;
#23607=VERTEX_POINT('',#107606) ;
#23608=VERTEX_POINT('',#107608) ;
#23609=VERTEX_POINT('',#107610) ;
#23610=VERTEX_POINT('',#107612) ;
#23611=VERTEX_POINT('',#107614) ;
#23612=VERTEX_POINT('',#107616) ;
#23613=VERTEX_POINT('',#107618) ;
#23614=VERTEX_POINT('',#107620) ;
#23615=VERTEX_POINT('',#107622) ;
#23616=VERTEX_POINT('',#107624) ;
#23617=VERTEX_POINT('',#107626) ;
#23618=VERTEX_POINT('',#107628) ;
#23619=VERTEX_POINT('',#107630) ;
#23620=VERTEX_POINT('',#107632) ;
#23621=VERTEX_POINT('',#107634) ;
#23622=VERTEX_POINT('',#107638) ;
#23623=VERTEX_POINT('',#107640) ;
#23624=VERTEX_POINT('',#107644) ;
#23625=VERTEX_POINT('',#107646) ;
#23626=VERTEX_POINT('',#107650) ;
#23627=VERTEX_POINT('',#107652) ;
#23628=VERTEX_POINT('',#107656) ;
#23629=VERTEX_POINT('',#107658) ;
#23630=VERTEX_POINT('',#107662) ;
#23631=VERTEX_POINT('',#107664) ;
#23632=VERTEX_POINT('',#107668) ;
#23633=VERTEX_POINT('',#107670) ;
#23634=VERTEX_POINT('',#107674) ;
#23635=VERTEX_POINT('',#107676) ;
#23636=VERTEX_POINT('',#107680) ;
#23637=VERTEX_POINT('',#107682) ;
#23638=VERTEX_POINT('',#107686) ;
#23639=VERTEX_POINT('',#107688) ;
#23640=VERTEX_POINT('',#107692) ;
#23641=VERTEX_POINT('',#107694) ;
#23642=VERTEX_POINT('',#107698) ;
#23643=VERTEX_POINT('',#107700) ;
#23644=VERTEX_POINT('',#107704) ;
#23645=VERTEX_POINT('',#107706) ;
#23646=VERTEX_POINT('',#107710) ;
#23647=VERTEX_POINT('',#107712) ;
#23648=VERTEX_POINT('',#107716) ;
#23649=VERTEX_POINT('',#107718) ;
#23650=VERTEX_POINT('',#107722) ;
#23651=VERTEX_POINT('',#107724) ;
#23652=VERTEX_POINT('',#107728) ;
#23653=VERTEX_POINT('',#107730) ;
#23654=VERTEX_POINT('',#107734) ;
#23655=VERTEX_POINT('',#107736) ;
#23656=VERTEX_POINT('',#107740) ;
#23657=VERTEX_POINT('',#107742) ;
#23658=VERTEX_POINT('',#107746) ;
#23659=VERTEX_POINT('',#107748) ;
#23660=VERTEX_POINT('',#107752) ;
#23661=VERTEX_POINT('',#107754) ;
#23662=VERTEX_POINT('',#107758) ;
#23663=VERTEX_POINT('',#107773) ;
#23664=VERTEX_POINT('',#107790) ;
#23665=VERTEX_POINT('',#107809) ;
#23666=VERTEX_POINT('',#107842) ;
#23667=VERTEX_POINT('',#107893) ;
#23668=VERTEX_POINT('',#107894) ;
#23669=VERTEX_POINT('',#107990) ;
#23670=VERTEX_POINT('',#107991) ;
#23671=VERTEX_POINT('',#108087) ;
#23672=VERTEX_POINT('',#108088) ;
#23673=VERTEX_POINT('',#108184) ;
#23674=VERTEX_POINT('',#108185) ;
#23675=VERTEX_POINT('',#108281) ;
#23676=VERTEX_POINT('',#108282) ;
#23677=VERTEX_POINT('',#108378) ;
#23678=VERTEX_POINT('',#108379) ;
#23679=VERTEX_POINT('',#108475) ;
#23680=VERTEX_POINT('',#108476) ;
#23681=VERTEX_POINT('',#108572) ;
#23682=VERTEX_POINT('',#108573) ;
#23683=VERTEX_POINT('',#108765) ;
#23684=VERTEX_POINT('',#108782) ;
#23685=VERTEX_POINT('',#108804) ;
#23686=VERTEX_POINT('',#108821) ;
#23687=VERTEX_POINT('',#108843) ;
#23688=VERTEX_POINT('',#108860) ;
#23689=VERTEX_POINT('',#108882) ;
#23690=VERTEX_POINT('',#108899) ;
#23691=VERTEX_POINT('',#108921) ;
#23692=VERTEX_POINT('',#108938) ;
#23693=VERTEX_POINT('',#108960) ;
#23694=VERTEX_POINT('',#108977) ;
#23695=VERTEX_POINT('',#108999) ;
#23696=VERTEX_POINT('',#109016) ;
#23697=VERTEX_POINT('',#109038) ;
#23698=VERTEX_POINT('',#109055) ;
#23699=VERTEX_POINT('',#109077) ;
#23700=VERTEX_POINT('',#109094) ;
#30281=EDGE_CURVE('',#23367,#23367,#19339,.T.) ;
#30282=EDGE_CURVE('',#23367,#23368,#19340,.T.) ;
#30283=EDGE_CURVE('',#23368,#23368,#19341,.T.) ;
#30284=EDGE_CURVE('',#23369,#23369,#1529,.T.) ;
#30285=EDGE_CURVE('',#23370,#23370,#19342,.T.) ;
#30286=EDGE_CURVE('',#23370,#23371,#19343,.T.) ;
#30287=EDGE_CURVE('',#23371,#23371,#19344,.T.) ;
#30288=EDGE_CURVE('',#23372,#23372,#1530,.T.) ;
#30289=EDGE_CURVE('',#23373,#23373,#19345,.T.) ;
#30290=EDGE_CURVE('',#23374,#23374,#19346,.T.) ;
#30291=EDGE_CURVE('',#23369,#23375,#1531,.T.) ;
#30292=EDGE_CURVE('',#23375,#23376,#1532,.T.) ;
#30293=EDGE_CURVE('',#23376,#23375,#1533,.T.) ;
#30294=EDGE_CURVE('',#23372,#23377,#1534,.T.) ;
#30295=EDGE_CURVE('',#23377,#23378,#1535,.T.) ;
#30296=EDGE_CURVE('',#23378,#23377,#1536,.T.) ;
#30297=EDGE_CURVE('',#23379,#23380,#19347,.T.) ;
#30298=EDGE_CURVE('',#23379,#23381,#1537,.T.) ;
#30299=EDGE_CURVE('',#23381,#23382,#19348,.T.) ;
#30300=EDGE_CURVE('',#23380,#23382,#1538,.T.) ;
#30301=EDGE_CURVE('',#23379,#23383,#5995,.T.) ;
#30302=EDGE_CURVE('',#23383,#23384,#1539,.T.) ;
#30303=EDGE_CURVE('',#23384,#23381,#5996,.T.) ;
#30304=EDGE_CURVE('',#23383,#23385,#19349,.T.) ;
#30305=EDGE_CURVE('',#23385,#23386,#1540,.T.) ;
#30306=EDGE_CURVE('',#23386,#23384,#19350,.T.) ;
#30307=EDGE_CURVE('',#23385,#23387,#5997,.T.) ;
#30308=EDGE_CURVE('',#23387,#23388,#1541,.T.) ;
#30309=EDGE_CURVE('',#23388,#23386,#5998,.T.) ;
#30310=EDGE_CURVE('',#23389,#23387,#19351,.T.) ;
#30311=EDGE_CURVE('',#23389,#23390,#1542,.T.) ;
#30312=EDGE_CURVE('',#23390,#23388,#19352,.T.) ;
#30313=EDGE_CURVE('',#23389,#23391,#5999,.T.) ;
#30314=EDGE_CURVE('',#23391,#23392,#1543,.T.) ;
#30315=EDGE_CURVE('',#23392,#23390,#6000,.T.) ;
#30316=EDGE_CURVE('',#23391,#23393,#19353,.T.) ;
#30317=EDGE_CURVE('',#23393,#23394,#1544,.T.) ;
#30318=EDGE_CURVE('',#23394,#23392,#19354,.T.) ;
#30319=EDGE_CURVE('',#23393,#23395,#6001,.T.) ;
#30320=EDGE_CURVE('',#23395,#23396,#1545,.T.) ;
#30321=EDGE_CURVE('',#23396,#23394,#6002,.T.) ;
#30322=EDGE_CURVE('',#23397,#23395,#19355,.T.) ;
#30323=EDGE_CURVE('',#23397,#23398,#1546,.T.) ;
#30324=EDGE_CURVE('',#23398,#23396,#19356,.T.) ;
#30325=EDGE_CURVE('',#23397,#23399,#6003,.T.) ;
#30326=EDGE_CURVE('',#23399,#23400,#1547,.T.) ;
#30327=EDGE_CURVE('',#23400,#23398,#6004,.T.) ;
#30328=EDGE_CURVE('',#23399,#23401,#19357,.T.) ;
#30329=EDGE_CURVE('',#23401,#23402,#1548,.T.) ;
#30330=EDGE_CURVE('',#23402,#23400,#19358,.T.) ;
#30331=EDGE_CURVE('',#23401,#23403,#6005,.T.) ;
#30332=EDGE_CURVE('',#23403,#23404,#1549,.T.) ;
#30333=EDGE_CURVE('',#23404,#23402,#6006,.T.) ;
#30334=EDGE_CURVE('',#23405,#23403,#19359,.T.) ;
#30335=EDGE_CURVE('',#23405,#23406,#1550,.T.) ;
#30336=EDGE_CURVE('',#23406,#23404,#19360,.T.) ;
#30337=EDGE_CURVE('',#23405,#23407,#6007,.T.) ;
#30338=EDGE_CURVE('',#23407,#23408,#1551,.T.) ;
#30339=EDGE_CURVE('',#23408,#23406,#6008,.T.) ;
#30340=EDGE_CURVE('',#23407,#23409,#19361,.T.) ;
#30341=EDGE_CURVE('',#23409,#23410,#1552,.T.) ;
#30342=EDGE_CURVE('',#23410,#23408,#19362,.T.) ;
#30343=EDGE_CURVE('',#23409,#23411,#6009,.T.) ;
#30344=EDGE_CURVE('',#23411,#23412,#1553,.T.) ;
#30345=EDGE_CURVE('',#23412,#23410,#6010,.T.) ;
#30346=EDGE_CURVE('',#23413,#23411,#19363,.T.) ;
#30347=EDGE_CURVE('',#23413,#23414,#1554,.T.) ;
#30348=EDGE_CURVE('',#23414,#23412,#19364,.T.) ;
#30349=EDGE_CURVE('',#23413,#23415,#6011,.T.) ;
#30350=EDGE_CURVE('',#23415,#23416,#1555,.T.) ;
#30351=EDGE_CURVE('',#23416,#23414,#6012,.T.) ;
#30352=EDGE_CURVE('',#23415,#23417,#19365,.T.) ;
#30353=EDGE_CURVE('',#23417,#23418,#1556,.T.) ;
#30354=EDGE_CURVE('',#23418,#23416,#19366,.T.) ;
#30355=EDGE_CURVE('',#23417,#23419,#6013,.T.) ;
#30356=EDGE_CURVE('',#23419,#23420,#1557,.T.) ;
#30357=EDGE_CURVE('',#23420,#23418,#6014,.T.) ;
#30358=EDGE_CURVE('',#23421,#23419,#19367,.T.) ;
#30359=EDGE_CURVE('',#23421,#23422,#1558,.T.) ;
#30360=EDGE_CURVE('',#23422,#23420,#19368,.T.) ;
#30361=EDGE_CURVE('',#23421,#23423,#6015,.T.) ;
#30362=EDGE_CURVE('',#23423,#23424,#1559,.T.) ;
#30363=EDGE_CURVE('',#23424,#23422,#6016,.T.) ;
#30364=EDGE_CURVE('',#23423,#23425,#19369,.T.) ;
#30365=EDGE_CURVE('',#23425,#23426,#1560,.T.) ;
#30366=EDGE_CURVE('',#23426,#23424,#19370,.T.) ;
#30367=EDGE_CURVE('',#23425,#23427,#6017,.T.) ;
#30368=EDGE_CURVE('',#23427,#23428,#1561,.T.) ;
#30369=EDGE_CURVE('',#23428,#23426,#6018,.T.) ;
#30370=EDGE_CURVE('',#23429,#23427,#19371,.T.) ;
#30371=EDGE_CURVE('',#23429,#23430,#1562,.T.) ;
#30372=EDGE_CURVE('',#23430,#23428,#19372,.T.) ;
#30373=EDGE_CURVE('',#23429,#23431,#6019,.T.) ;
#30374=EDGE_CURVE('',#23431,#23432,#1563,.T.) ;
#30375=EDGE_CURVE('',#23432,#23430,#6020,.T.) ;
#30376=EDGE_CURVE('',#23431,#23433,#19373,.T.) ;
#30377=EDGE_CURVE('',#23433,#23434,#1564,.T.) ;
#30378=EDGE_CURVE('',#23434,#23432,#19374,.T.) ;
#30379=EDGE_CURVE('',#23433,#23435,#6021,.T.) ;
#30380=EDGE_CURVE('',#23435,#23436,#1565,.T.) ;
#30381=EDGE_CURVE('',#23436,#23434,#6022,.T.) ;
#30382=EDGE_CURVE('',#23437,#23435,#19375,.T.) ;
#30383=EDGE_CURVE('',#23437,#23438,#1566,.T.) ;
#30384=EDGE_CURVE('',#23438,#23436,#19376,.T.) ;
#30385=EDGE_CURVE('',#23437,#23439,#6023,.T.) ;
#30386=EDGE_CURVE('',#23439,#23440,#1567,.T.) ;
#30387=EDGE_CURVE('',#23440,#23438,#6024,.T.) ;
#30388=EDGE_CURVE('',#23439,#23441,#19377,.T.) ;
#30389=EDGE_CURVE('',#23441,#23442,#1568,.T.) ;
#30390=EDGE_CURVE('',#23442,#23440,#19378,.T.) ;
#30391=EDGE_CURVE('',#23441,#23443,#6025,.T.) ;
#30392=EDGE_CURVE('',#23443,#23444,#1569,.T.) ;
#30393=EDGE_CURVE('',#23444,#23442,#6026,.T.) ;
#30394=EDGE_CURVE('',#23445,#23443,#19379,.T.) ;
#30395=EDGE_CURVE('',#23445,#23446,#1570,.T.) ;
#30396=EDGE_CURVE('',#23446,#23444,#19380,.T.) ;
#30397=EDGE_CURVE('',#23445,#23447,#6027,.T.) ;
#30398=EDGE_CURVE('',#23447,#23448,#1571,.T.) ;
#30399=EDGE_CURVE('',#23448,#23446,#6028,.T.) ;
#30400=EDGE_CURVE('',#23447,#23449,#19381,.T.) ;
#30401=EDGE_CURVE('',#23449,#23450,#1572,.T.) ;
#30402=EDGE_CURVE('',#23450,#23448,#19382,.T.) ;
#30403=EDGE_CURVE('',#23449,#23451,#6029,.T.) ;
#30404=EDGE_CURVE('',#23451,#23452,#1573,.T.) ;
#30405=EDGE_CURVE('',#23452,#23450,#6030,.T.) ;
#30406=EDGE_CURVE('',#23453,#23451,#19383,.T.) ;
#30407=EDGE_CURVE('',#23453,#23454,#1574,.T.) ;
#30408=EDGE_CURVE('',#23454,#23452,#19384,.T.) ;
#30409=EDGE_CURVE('',#23453,#23455,#6031,.T.) ;
#30410=EDGE_CURVE('',#23455,#23456,#1575,.T.) ;
#30411=EDGE_CURVE('',#23456,#23454,#6032,.T.) ;
#30412=EDGE_CURVE('',#23455,#23457,#19385,.T.) ;
#30413=EDGE_CURVE('',#23457,#23458,#1576,.T.) ;
#30414=EDGE_CURVE('',#23458,#23456,#19386,.T.) ;
#30415=EDGE_CURVE('',#23457,#23459,#6033,.T.) ;
#30416=EDGE_CURVE('',#23459,#23460,#1577,.T.) ;
#30417=EDGE_CURVE('',#23460,#23458,#6034,.T.) ;
#30418=EDGE_CURVE('',#23461,#23459,#19387,.T.) ;
#30419=EDGE_CURVE('',#23461,#23462,#1578,.T.) ;
#30420=EDGE_CURVE('',#23462,#23460,#19388,.T.) ;
#30421=EDGE_CURVE('',#23463,#23462,#6035,.T.) ;
#30422=EDGE_CURVE('',#23461,#23464,#6036,.T.) ;
#30423=EDGE_CURVE('',#23464,#23463,#1579,.T.) ;
#30424=EDGE_CURVE('',#23465,#23463,#19389,.T.) ;
#30425=EDGE_CURVE('',#23464,#23466,#19390,.T.) ;
#30426=EDGE_CURVE('',#23466,#23465,#1580,.T.) ;
#30427=EDGE_CURVE('',#23467,#23465,#6037,.T.) ;
#30428=EDGE_CURVE('',#23466,#23468,#6038,.T.) ;
#30429=EDGE_CURVE('',#23468,#23467,#1581,.T.) ;
#30430=EDGE_CURVE('',#23469,#23467,#19391,.T.) ;
#30431=EDGE_CURVE('',#23470,#23468,#19392,.T.) ;
#30432=EDGE_CURVE('',#23470,#23469,#1582,.T.) ;
#30433=EDGE_CURVE('',#23471,#23469,#6039,.T.) ;
#30434=EDGE_CURVE('',#23470,#23472,#6040,.T.) ;
#30435=EDGE_CURVE('',#23472,#23471,#1583,.T.) ;
#30436=EDGE_CURVE('',#23473,#23471,#19393,.T.) ;
#30437=EDGE_CURVE('',#23472,#23474,#19394,.T.) ;
#30438=EDGE_CURVE('',#23474,#23473,#1584,.T.) ;
#30439=EDGE_CURVE('',#23475,#23473,#6041,.T.) ;
#30440=EDGE_CURVE('',#23474,#23476,#6042,.T.) ;
#30441=EDGE_CURVE('',#23476,#23475,#1585,.T.) ;
#30442=EDGE_CURVE('',#23477,#23475,#19395,.T.) ;
#30443=EDGE_CURVE('',#23478,#23476,#19396,.T.) ;
#30444=EDGE_CURVE('',#23478,#23477,#1586,.T.) ;
#30445=EDGE_CURVE('',#23479,#23477,#6043,.T.) ;
#30446=EDGE_CURVE('',#23478,#23480,#6044,.T.) ;
#30447=EDGE_CURVE('',#23480,#23479,#1587,.T.) ;
#30448=EDGE_CURVE('',#23481,#23479,#19397,.T.) ;
#30449=EDGE_CURVE('',#23480,#23482,#19398,.T.) ;
#30450=EDGE_CURVE('',#23482,#23481,#1588,.T.) ;
#30451=EDGE_CURVE('',#23483,#23481,#6045,.T.) ;
#30452=EDGE_CURVE('',#23482,#23484,#6046,.T.) ;
#30453=EDGE_CURVE('',#23484,#23483,#1589,.T.) ;
#30454=EDGE_CURVE('',#23485,#23483,#19399,.T.) ;
#30455=EDGE_CURVE('',#23486,#23484,#19400,.T.) ;
#30456=EDGE_CURVE('',#23486,#23485,#1590,.T.) ;
#30457=EDGE_CURVE('',#23487,#23485,#6047,.T.) ;
#30458=EDGE_CURVE('',#23486,#23488,#6048,.T.) ;
#30459=EDGE_CURVE('',#23488,#23487,#1591,.T.) ;
#30460=EDGE_CURVE('',#23489,#23487,#19401,.T.) ;
#30461=EDGE_CURVE('',#23488,#23490,#19402,.T.) ;
#30462=EDGE_CURVE('',#23490,#23489,#1592,.T.) ;
#30463=EDGE_CURVE('',#23491,#23489,#6049,.T.) ;
#30464=EDGE_CURVE('',#23490,#23492,#6050,.T.) ;
#30465=EDGE_CURVE('',#23492,#23491,#1593,.T.) ;
#30466=EDGE_CURVE('',#23493,#23491,#19403,.T.) ;
#30467=EDGE_CURVE('',#23494,#23492,#19404,.T.) ;
#30468=EDGE_CURVE('',#23494,#23493,#1594,.T.) ;
#30469=EDGE_CURVE('',#23495,#23493,#6051,.T.) ;
#30470=EDGE_CURVE('',#23494,#23496,#6052,.T.) ;
#30471=EDGE_CURVE('',#23496,#23495,#1595,.T.) ;
#30472=EDGE_CURVE('',#23497,#23495,#19405,.T.) ;
#30473=EDGE_CURVE('',#23496,#23498,#19406,.T.) ;
#30474=EDGE_CURVE('',#23498,#23497,#1596,.T.) ;
#30475=EDGE_CURVE('',#23499,#23497,#6053,.T.) ;
#30476=EDGE_CURVE('',#23498,#23500,#6054,.T.) ;
#30477=EDGE_CURVE('',#23500,#23499,#1597,.T.) ;
#30478=EDGE_CURVE('',#23501,#23499,#19407,.T.) ;
#30479=EDGE_CURVE('',#23502,#23500,#19408,.T.) ;
#30480=EDGE_CURVE('',#23502,#23501,#1598,.T.) ;
#30481=EDGE_CURVE('',#23503,#23501,#6055,.T.) ;
#30482=EDGE_CURVE('',#23502,#23504,#6056,.T.) ;
#30483=EDGE_CURVE('',#23504,#23503,#1599,.T.) ;
#30484=EDGE_CURVE('',#23505,#23503,#19409,.T.) ;
#30485=EDGE_CURVE('',#23504,#23506,#19410,.T.) ;
#30486=EDGE_CURVE('',#23506,#23505,#1600,.T.) ;
#30487=EDGE_CURVE('',#23507,#23505,#6057,.T.) ;
#30488=EDGE_CURVE('',#23506,#23508,#6058,.T.) ;
#30489=EDGE_CURVE('',#23508,#23507,#1601,.T.) ;
#30490=EDGE_CURVE('',#23509,#23507,#19411,.T.) ;
#30491=EDGE_CURVE('',#23510,#23508,#19412,.T.) ;
#30492=EDGE_CURVE('',#23510,#23509,#1602,.T.) ;
#30493=EDGE_CURVE('',#23511,#23509,#6059,.T.) ;
#30494=EDGE_CURVE('',#23510,#23512,#6060,.T.) ;
#30495=EDGE_CURVE('',#23512,#23511,#1603,.T.) ;
#30496=EDGE_CURVE('',#23513,#23511,#19413,.T.) ;
#30497=EDGE_CURVE('',#23512,#23514,#19414,.T.) ;
#30498=EDGE_CURVE('',#23514,#23513,#1604,.T.) ;
#30499=EDGE_CURVE('',#23515,#23513,#6061,.T.) ;
#30500=EDGE_CURVE('',#23514,#23516,#6062,.T.) ;
#30501=EDGE_CURVE('',#23516,#23515,#1605,.T.) ;
#30502=EDGE_CURVE('',#23517,#23515,#19415,.T.) ;
#30503=EDGE_CURVE('',#23518,#23516,#19416,.T.) ;
#30504=EDGE_CURVE('',#23518,#23517,#1606,.T.) ;
#30505=EDGE_CURVE('',#23519,#23517,#6063,.T.) ;
#30506=EDGE_CURVE('',#23518,#23520,#6064,.T.) ;
#30507=EDGE_CURVE('',#23520,#23519,#1607,.T.) ;
#30508=EDGE_CURVE('',#23521,#23519,#19417,.T.) ;
#30509=EDGE_CURVE('',#23520,#23522,#19418,.T.) ;
#30510=EDGE_CURVE('',#23522,#23521,#1608,.T.) ;
#30511=EDGE_CURVE('',#23523,#23521,#6065,.T.) ;
#30512=EDGE_CURVE('',#23522,#23524,#6066,.T.) ;
#30513=EDGE_CURVE('',#23524,#23523,#1609,.T.) ;
#30514=EDGE_CURVE('',#23525,#23523,#19419,.T.) ;
#30515=EDGE_CURVE('',#23526,#23524,#19420,.T.) ;
#30516=EDGE_CURVE('',#23526,#23525,#1610,.T.) ;
#30517=EDGE_CURVE('',#23527,#23525,#6067,.T.) ;
#30518=EDGE_CURVE('',#23526,#23528,#6068,.T.) ;
#30519=EDGE_CURVE('',#23528,#23527,#1611,.T.) ;
#30520=EDGE_CURVE('',#23529,#23527,#19421,.T.) ;
#30521=EDGE_CURVE('',#23528,#23530,#19422,.T.) ;
#30522=EDGE_CURVE('',#23530,#23529,#1612,.T.) ;
#30523=EDGE_CURVE('',#23531,#23529,#6069,.T.) ;
#30524=EDGE_CURVE('',#23530,#23532,#6070,.T.) ;
#30525=EDGE_CURVE('',#23532,#23531,#1613,.T.) ;
#30526=EDGE_CURVE('',#23533,#23531,#19423,.T.) ;
#30527=EDGE_CURVE('',#23534,#23532,#19424,.T.) ;
#30528=EDGE_CURVE('',#23534,#23533,#1614,.T.) ;
#30529=EDGE_CURVE('',#23535,#23533,#6071,.T.) ;
#30530=EDGE_CURVE('',#23534,#23536,#6072,.T.) ;
#30531=EDGE_CURVE('',#23536,#23535,#1615,.T.) ;
#30532=EDGE_CURVE('',#23537,#23535,#19425,.T.) ;
#30533=EDGE_CURVE('',#23536,#23538,#19426,.T.) ;
#30534=EDGE_CURVE('',#23538,#23537,#1616,.T.) ;
#30535=EDGE_CURVE('',#23382,#23537,#6073,.T.) ;
#30536=EDGE_CURVE('',#23538,#23380,#6074,.T.) ;
#30537=EDGE_CURVE('',#23539,#23463,#6075,.T.) ;
#30538=EDGE_CURVE('',#23540,#23539,#6076,.T.) ;
#30539=EDGE_CURVE('',#23462,#23540,#6077,.T.) ;
#30540=EDGE_CURVE('',#23541,#23465,#6078,.T.) ;
#30541=EDGE_CURVE('',#23539,#23541,#19427,.T.) ;
#30542=EDGE_CURVE('',#23542,#23467,#6079,.T.) ;
#30543=EDGE_CURVE('',#23541,#23542,#6080,.T.) ;
#30544=EDGE_CURVE('',#23469,#23543,#6081,.T.) ;
#30545=EDGE_CURVE('',#23542,#23543,#19428,.T.) ;
#30546=EDGE_CURVE('',#23544,#23471,#6082,.T.) ;
#30547=EDGE_CURVE('',#23543,#23544,#6083,.T.) ;
#30548=EDGE_CURVE('',#23545,#23473,#6084,.T.) ;
#30549=EDGE_CURVE('',#23544,#23545,#19429,.T.) ;
#30550=EDGE_CURVE('',#23546,#23475,#6085,.T.) ;
#30551=EDGE_CURVE('',#23545,#23546,#6086,.T.) ;
#30552=EDGE_CURVE('',#23477,#23547,#6087,.T.) ;
#30553=EDGE_CURVE('',#23546,#23547,#19430,.T.) ;
#30554=EDGE_CURVE('',#23548,#23479,#6088,.T.) ;
#30555=EDGE_CURVE('',#23547,#23548,#6089,.T.) ;
#30556=EDGE_CURVE('',#23549,#23481,#6090,.T.) ;
#30557=EDGE_CURVE('',#23548,#23549,#19431,.T.) ;
#30558=EDGE_CURVE('',#23550,#23483,#6091,.T.) ;
#30559=EDGE_CURVE('',#23549,#23550,#6092,.T.) ;
#30560=EDGE_CURVE('',#23485,#23551,#6093,.T.) ;
#30561=EDGE_CURVE('',#23550,#23551,#19432,.T.) ;
#30562=EDGE_CURVE('',#23552,#23487,#6094,.T.) ;
#30563=EDGE_CURVE('',#23551,#23552,#6095,.T.) ;
#30564=EDGE_CURVE('',#23553,#23489,#6096,.T.) ;
#30565=EDGE_CURVE('',#23552,#23553,#19433,.T.) ;
#30566=EDGE_CURVE('',#23554,#23491,#6097,.T.) ;
#30567=EDGE_CURVE('',#23553,#23554,#6098,.T.) ;
#30568=EDGE_CURVE('',#23493,#23555,#6099,.T.) ;
#30569=EDGE_CURVE('',#23554,#23555,#19434,.T.) ;
#30570=EDGE_CURVE('',#23556,#23495,#6100,.T.) ;
#30571=EDGE_CURVE('',#23555,#23556,#6101,.T.) ;
#30572=EDGE_CURVE('',#23557,#23497,#6102,.T.) ;
#30573=EDGE_CURVE('',#23556,#23557,#19435,.T.) ;
#30574=EDGE_CURVE('',#23558,#23499,#6103,.T.) ;
#30575=EDGE_CURVE('',#23557,#23558,#6104,.T.) ;
#30576=EDGE_CURVE('',#23501,#23559,#6105,.T.) ;
#30577=EDGE_CURVE('',#23558,#23559,#19436,.T.) ;
#30578=EDGE_CURVE('',#23560,#23503,#6106,.T.) ;
#30579=EDGE_CURVE('',#23559,#23560,#6107,.T.) ;
#30580=EDGE_CURVE('',#23561,#23505,#6108,.T.) ;
#30581=EDGE_CURVE('',#23560,#23561,#19437,.T.) ;
#30582=EDGE_CURVE('',#23562,#23507,#6109,.T.) ;
#30583=EDGE_CURVE('',#23561,#23562,#6110,.T.) ;
#30584=EDGE_CURVE('',#23509,#23563,#6111,.T.) ;
#30585=EDGE_CURVE('',#23562,#23563,#19438,.T.) ;
#30586=EDGE_CURVE('',#23564,#23511,#6112,.T.) ;
#30587=EDGE_CURVE('',#23563,#23564,#6113,.T.) ;
#30588=EDGE_CURVE('',#23565,#23513,#6114,.T.) ;
#30589=EDGE_CURVE('',#23564,#23565,#19439,.T.) ;
#30590=EDGE_CURVE('',#23566,#23515,#6115,.T.) ;
#30591=EDGE_CURVE('',#23565,#23566,#6116,.T.) ;
#30592=EDGE_CURVE('',#23517,#23567,#6117,.T.) ;
#30593=EDGE_CURVE('',#23566,#23567,#19440,.T.) ;
#30594=EDGE_CURVE('',#23568,#23519,#6118,.T.) ;
#30595=EDGE_CURVE('',#23567,#23568,#6119,.T.) ;
#30596=EDGE_CURVE('',#23569,#23521,#6120,.T.) ;
#30597=EDGE_CURVE('',#23568,#23569,#19441,.T.) ;
#30598=EDGE_CURVE('',#23570,#23523,#6121,.T.) ;
#30599=EDGE_CURVE('',#23569,#23570,#6122,.T.) ;
#30600=EDGE_CURVE('',#23525,#23571,#6123,.T.) ;
#30601=EDGE_CURVE('',#23570,#23571,#19442,.T.) ;
#30602=EDGE_CURVE('',#23572,#23527,#6124,.T.) ;
#30603=EDGE_CURVE('',#23571,#23572,#6125,.T.) ;
#30604=EDGE_CURVE('',#23573,#23529,#6126,.T.) ;
#30605=EDGE_CURVE('',#23572,#23573,#19443,.T.) ;
#30606=EDGE_CURVE('',#23574,#23531,#6127,.T.) ;
#30607=EDGE_CURVE('',#23573,#23574,#6128,.T.) ;
#30608=EDGE_CURVE('',#23533,#23575,#6129,.T.) ;
#30609=EDGE_CURVE('',#23574,#23575,#19444,.T.) ;
#30610=EDGE_CURVE('',#23576,#23535,#6130,.T.) ;
#30611=EDGE_CURVE('',#23575,#23576,#6131,.T.) ;
#30612=EDGE_CURVE('',#23577,#23537,#6132,.T.) ;
#30613=EDGE_CURVE('',#23576,#23577,#19445,.T.) ;
#30614=EDGE_CURVE('',#23578,#23382,#6133,.T.) ;
#30615=EDGE_CURVE('',#23577,#23578,#6134,.T.) ;
#30616=EDGE_CURVE('',#23381,#23579,#6135,.T.) ;
#30617=EDGE_CURVE('',#23578,#23579,#19446,.T.) ;
#30618=EDGE_CURVE('',#23468,#23461,#19447,.T.) ;
#30619=EDGE_CURVE('',#23476,#23470,#19448,.T.) ;
#30620=EDGE_CURVE('',#23459,#23453,#19449,.T.) ;
#30621=EDGE_CURVE('',#23484,#23478,#19450,.T.) ;
#30622=EDGE_CURVE('',#23451,#23445,#19451,.T.) ;
#30623=EDGE_CURVE('',#23492,#23486,#19452,.T.) ;
#30624=EDGE_CURVE('',#23443,#23437,#19453,.T.) ;
#30625=EDGE_CURVE('',#23500,#23494,#19454,.T.) ;
#30626=EDGE_CURVE('',#23435,#23429,#19455,.T.) ;
#30627=EDGE_CURVE('',#23508,#23502,#19456,.T.) ;
#30628=EDGE_CURVE('',#23427,#23421,#19457,.T.) ;
#30629=EDGE_CURVE('',#23516,#23510,#19458,.T.) ;
#30630=EDGE_CURVE('',#23419,#23413,#19459,.T.) ;
#30631=EDGE_CURVE('',#23524,#23518,#19460,.T.) ;
#30632=EDGE_CURVE('',#23411,#23405,#19461,.T.) ;
#30633=EDGE_CURVE('',#23532,#23526,#19462,.T.) ;
#30634=EDGE_CURVE('',#23403,#23397,#19463,.T.) ;
#30635=EDGE_CURVE('',#23380,#23534,#19464,.T.) ;
#30636=EDGE_CURVE('',#23580,#23389,#19465,.T.) ;
#30637=EDGE_CURVE('',#23395,#23580,#19466,.T.) ;
#30638=EDGE_CURVE('',#23376,#23580,#19467,.T.) ;
#30639=EDGE_CURVE('',#23387,#23379,#19468,.T.) ;
#30640=EDGE_CURVE('',#23378,#23581,#19469,.T.) ;
#30641=EDGE_CURVE('',#23581,#23582,#19470,.T.) ;
#30642=EDGE_CURVE('',#23583,#23582,#19471,.T.) ;
#30643=EDGE_CURVE('',#23583,#23584,#19472,.T.) ;
#30644=EDGE_CURVE('',#23585,#23584,#19473,.T.) ;
#30645=EDGE_CURVE('',#23585,#23586,#19474,.T.) ;
#30646=EDGE_CURVE('',#23587,#23586,#19475,.T.) ;
#30647=EDGE_CURVE('',#23587,#23588,#19476,.T.) ;
#30648=EDGE_CURVE('',#23589,#23588,#19477,.T.) ;
#30649=EDGE_CURVE('',#23589,#23590,#19478,.T.) ;
#30650=EDGE_CURVE('',#23591,#23590,#19479,.T.) ;
#30651=EDGE_CURVE('',#23591,#23592,#19480,.T.) ;
#30652=EDGE_CURVE('',#23593,#23592,#19481,.T.) ;
#30653=EDGE_CURVE('',#23593,#23594,#19482,.T.) ;
#30654=EDGE_CURVE('',#23595,#23594,#19483,.T.) ;
#30655=EDGE_CURVE('',#23595,#23596,#19484,.T.) ;
#30656=EDGE_CURVE('',#23597,#23596,#19485,.T.) ;
#30657=EDGE_CURVE('',#23597,#23598,#19486,.T.) ;
#30658=EDGE_CURVE('',#23599,#23598,#19487,.T.) ;
#30659=EDGE_CURVE('',#23599,#23600,#19488,.T.) ;
#30660=EDGE_CURVE('',#23601,#23600,#19489,.T.) ;
#30661=EDGE_CURVE('',#23601,#23602,#19490,.T.) ;
#30662=EDGE_CURVE('',#23603,#23602,#19491,.T.) ;
#30663=EDGE_CURVE('',#23603,#23604,#19492,.T.) ;
#30664=EDGE_CURVE('',#23605,#23604,#19493,.T.) ;
#30665=EDGE_CURVE('',#23605,#23606,#19494,.T.) ;
#30666=EDGE_CURVE('',#23607,#23606,#19495,.T.) ;
#30667=EDGE_CURVE('',#23607,#23608,#19496,.T.) ;
#30668=EDGE_CURVE('',#23609,#23608,#19497,.T.) ;
#30669=EDGE_CURVE('',#23609,#23610,#19498,.T.) ;
#30670=EDGE_CURVE('',#23611,#23610,#19499,.T.) ;
#30671=EDGE_CURVE('',#23611,#23612,#19500,.T.) ;
#30672=EDGE_CURVE('',#23613,#23612,#19501,.T.) ;
#30673=EDGE_CURVE('',#23613,#23614,#19502,.T.) ;
#30674=EDGE_CURVE('',#23615,#23614,#19503,.T.) ;
#30675=EDGE_CURVE('',#23615,#23616,#19504,.T.) ;
#30676=EDGE_CURVE('',#23617,#23616,#19505,.T.) ;
#30677=EDGE_CURVE('',#23617,#23618,#19506,.T.) ;
#30678=EDGE_CURVE('',#23619,#23618,#19507,.T.) ;
#30679=EDGE_CURVE('',#23619,#23620,#19508,.T.) ;
#30680=EDGE_CURVE('',#23621,#23620,#19509,.T.) ;
#30681=EDGE_CURVE('',#23621,#23581,#19510,.T.) ;
#30682=EDGE_CURVE('',#23622,#23619,#6136,.T.) ;
#30683=EDGE_CURVE('',#23623,#23622,#19511,.T.) ;
#30684=EDGE_CURVE('',#23620,#23623,#6137,.T.) ;
#30685=EDGE_CURVE('',#23624,#23617,#6138,.T.) ;
#30686=EDGE_CURVE('',#23625,#23624,#19512,.T.) ;
#30687=EDGE_CURVE('',#23618,#23625,#6139,.T.) ;
#30688=EDGE_CURVE('',#23626,#23615,#6140,.T.) ;
#30689=EDGE_CURVE('',#23627,#23626,#19513,.T.) ;
#30690=EDGE_CURVE('',#23616,#23627,#6141,.T.) ;
#30691=EDGE_CURVE('',#23628,#23613,#6142,.T.) ;
#30692=EDGE_CURVE('',#23629,#23628,#19514,.T.) ;
#30693=EDGE_CURVE('',#23614,#23629,#6143,.T.) ;
#30694=EDGE_CURVE('',#23630,#23611,#6144,.T.) ;
#30695=EDGE_CURVE('',#23631,#23630,#19515,.T.) ;
#30696=EDGE_CURVE('',#23612,#23631,#6145,.T.) ;
#30697=EDGE_CURVE('',#23632,#23609,#6146,.T.) ;
#30698=EDGE_CURVE('',#23633,#23632,#19516,.T.) ;
#30699=EDGE_CURVE('',#23610,#23633,#6147,.T.) ;
#30700=EDGE_CURVE('',#23634,#23607,#6148,.T.) ;
#30701=EDGE_CURVE('',#23635,#23634,#19517,.T.) ;
#30702=EDGE_CURVE('',#23608,#23635,#6149,.T.) ;
#30703=EDGE_CURVE('',#23636,#23605,#6150,.T.) ;
#30704=EDGE_CURVE('',#23637,#23636,#19518,.T.) ;
#30705=EDGE_CURVE('',#23606,#23637,#6151,.T.) ;
#30706=EDGE_CURVE('',#23638,#23603,#6152,.T.) ;
#30707=EDGE_CURVE('',#23639,#23638,#19519,.T.) ;
#30708=EDGE_CURVE('',#23604,#23639,#6153,.T.) ;
#30709=EDGE_CURVE('',#23640,#23601,#6154,.T.) ;
#30710=EDGE_CURVE('',#23641,#23640,#19520,.T.) ;
#30711=EDGE_CURVE('',#23602,#23641,#6155,.T.) ;
#30712=EDGE_CURVE('',#23642,#23599,#6156,.T.) ;
#30713=EDGE_CURVE('',#23643,#23642,#19521,.T.) ;
#30714=EDGE_CURVE('',#23600,#23643,#6157,.T.) ;
#30715=EDGE_CURVE('',#23644,#23597,#6158,.T.) ;
#30716=EDGE_CURVE('',#23645,#23644,#19522,.T.) ;
#30717=EDGE_CURVE('',#23598,#23645,#6159,.T.) ;
#30718=EDGE_CURVE('',#23646,#23595,#6160,.T.) ;
#30719=EDGE_CURVE('',#23647,#23646,#19523,.T.) ;
#30720=EDGE_CURVE('',#23596,#23647,#6161,.T.) ;
#30721=EDGE_CURVE('',#23648,#23593,#6162,.T.) ;
#30722=EDGE_CURVE('',#23649,#23648,#19524,.T.) ;
#30723=EDGE_CURVE('',#23594,#23649,#6163,.T.) ;
#30724=EDGE_CURVE('',#23650,#23591,#6164,.T.) ;
#30725=EDGE_CURVE('',#23651,#23650,#19525,.T.) ;
#30726=EDGE_CURVE('',#23592,#23651,#6165,.T.) ;
#30727=EDGE_CURVE('',#23652,#23589,#6166,.T.) ;
#30728=EDGE_CURVE('',#23653,#23652,#19526,.T.) ;
#30729=EDGE_CURVE('',#23590,#23653,#6167,.T.) ;
#30730=EDGE_CURVE('',#23654,#23587,#6168,.T.) ;
#30731=EDGE_CURVE('',#23655,#23654,#19527,.T.) ;
#30732=EDGE_CURVE('',#23588,#23655,#6169,.T.) ;
#30733=EDGE_CURVE('',#23656,#23585,#6170,.T.) ;
#30734=EDGE_CURVE('',#23657,#23656,#19528,.T.) ;
#30735=EDGE_CURVE('',#23586,#23657,#6171,.T.) ;
#30736=EDGE_CURVE('',#23658,#23583,#6172,.T.) ;
#30737=EDGE_CURVE('',#23659,#23658,#19529,.T.) ;
#30738=EDGE_CURVE('',#23584,#23659,#6173,.T.) ;
#30739=EDGE_CURVE('',#23660,#23621,#6174,.T.) ;
#30740=EDGE_CURVE('',#23661,#23660,#19530,.T.) ;
#30741=EDGE_CURVE('',#23582,#23661,#6175,.T.) ;
#30742=EDGE_CURVE('',#23600,#23662,#1617,.T.) ;
#30743=EDGE_CURVE('',#23662,#23663,#19531,.T.) ;
#30744=EDGE_CURVE('',#23601,#23663,#1618,.T.) ;
#30745=EDGE_CURVE('',#23643,#23664,#1619,.T.) ;
#30746=EDGE_CURVE('',#23664,#23662,#6176,.T.) ;
#30747=EDGE_CURVE('',#23663,#23665,#6177,.T.) ;
#30748=EDGE_CURVE('',#23665,#23640,#1620,.T.) ;
#30749=EDGE_CURVE('',#23599,#23579,#1621,.T.) ;
#30750=EDGE_CURVE('',#23579,#23666,#6178,.T.) ;
#30751=EDGE_CURVE('',#23666,#23642,#1622,.T.) ;
#30752=EDGE_CURVE('',#23598,#23578,#1623,.T.) ;
#30753=EDGE_CURVE('',#23645,#23577,#1624,.T.) ;
#30754=EDGE_CURVE('',#23667,#23668,#6179,.T.) ;
#30755=EDGE_CURVE('',#23668,#23638,#1625,.T.) ;
#30756=EDGE_CURVE('',#23603,#23667,#1626,.T.) ;
#30757=EDGE_CURVE('',#23597,#23575,#1627,.T.) ;
#30758=EDGE_CURVE('',#23576,#23644,#1628,.T.) ;
#30759=EDGE_CURVE('',#23596,#23574,#1629,.T.) ;
#30760=EDGE_CURVE('',#23647,#23573,#1630,.T.) ;
#30761=EDGE_CURVE('',#23669,#23670,#6180,.T.) ;
#30762=EDGE_CURVE('',#23670,#23636,#1631,.T.) ;
#30763=EDGE_CURVE('',#23605,#23669,#1632,.T.) ;
#30764=EDGE_CURVE('',#23595,#23571,#1633,.T.) ;
#30765=EDGE_CURVE('',#23572,#23646,#1634,.T.) ;
#30766=EDGE_CURVE('',#23594,#23570,#1635,.T.) ;
#30767=EDGE_CURVE('',#23649,#23569,#1636,.T.) ;
#30768=EDGE_CURVE('',#23671,#23672,#6181,.T.) ;
#30769=EDGE_CURVE('',#23672,#23634,#1637,.T.) ;
#30770=EDGE_CURVE('',#23607,#23671,#1638,.T.) ;
#30771=EDGE_CURVE('',#23593,#23567,#1639,.T.) ;
#30772=EDGE_CURVE('',#23568,#23648,#1640,.T.) ;
#30773=EDGE_CURVE('',#23592,#23566,#1641,.T.) ;
#30774=EDGE_CURVE('',#23651,#23565,#1642,.T.) ;
#30775=EDGE_CURVE('',#23673,#23674,#6182,.T.) ;
#30776=EDGE_CURVE('',#23674,#23632,#1643,.T.) ;
#30777=EDGE_CURVE('',#23609,#23673,#1644,.T.) ;
#30778=EDGE_CURVE('',#23591,#23563,#1645,.T.) ;
#30779=EDGE_CURVE('',#23564,#23650,#1646,.T.) ;
#30780=EDGE_CURVE('',#23590,#23562,#1647,.T.) ;
#30781=EDGE_CURVE('',#23653,#23561,#1648,.T.) ;
#30782=EDGE_CURVE('',#23675,#23676,#6183,.T.) ;
#30783=EDGE_CURVE('',#23676,#23630,#1649,.T.) ;
#30784=EDGE_CURVE('',#23611,#23675,#1650,.T.) ;
#30785=EDGE_CURVE('',#23589,#23559,#1651,.T.) ;
#30786=EDGE_CURVE('',#23560,#23652,#1652,.T.) ;
#30787=EDGE_CURVE('',#23588,#23558,#1653,.T.) ;
#30788=EDGE_CURVE('',#23655,#23557,#1654,.T.) ;
#30789=EDGE_CURVE('',#23677,#23678,#6184,.T.) ;
#30790=EDGE_CURVE('',#23678,#23628,#1655,.T.) ;
#30791=EDGE_CURVE('',#23613,#23677,#1656,.T.) ;
#30792=EDGE_CURVE('',#23587,#23555,#1657,.T.) ;
#30793=EDGE_CURVE('',#23556,#23654,#1658,.T.) ;
#30794=EDGE_CURVE('',#23586,#23554,#1659,.T.) ;
#30795=EDGE_CURVE('',#23657,#23553,#1660,.T.) ;
#30796=EDGE_CURVE('',#23679,#23680,#6185,.T.) ;
#30797=EDGE_CURVE('',#23680,#23626,#1661,.T.) ;
#30798=EDGE_CURVE('',#23615,#23679,#1662,.T.) ;
#30799=EDGE_CURVE('',#23585,#23551,#1663,.T.) ;
#30800=EDGE_CURVE('',#23552,#23656,#1664,.T.) ;
#30801=EDGE_CURVE('',#23584,#23550,#1665,.T.) ;
#30802=EDGE_CURVE('',#23659,#23549,#1666,.T.) ;
#30803=EDGE_CURVE('',#23681,#23682,#6186,.T.) ;
#30804=EDGE_CURVE('',#23682,#23624,#1667,.T.) ;
#30805=EDGE_CURVE('',#23617,#23681,#1668,.T.) ;
#30806=EDGE_CURVE('',#23583,#23547,#1669,.T.) ;
#30807=EDGE_CURVE('',#23548,#23658,#1670,.T.) ;
#30808=EDGE_CURVE('',#23582,#23546,#1671,.T.) ;
#30809=EDGE_CURVE('',#23661,#23545,#1672,.T.) ;
#30810=EDGE_CURVE('',#23539,#23622,#1673,.T.) ;
#30811=EDGE_CURVE('',#23619,#23540,#1674,.T.) ;
#30812=EDGE_CURVE('',#23621,#23543,#1675,.T.) ;
#30813=EDGE_CURVE('',#23544,#23660,#1676,.T.) ;
#30814=EDGE_CURVE('',#23620,#23542,#1677,.T.) ;
#30815=EDGE_CURVE('',#23623,#23541,#1678,.T.) ;
#30816=EDGE_CURVE('',#23683,#23540,#19532,.T.) ;
#30817=EDGE_CURVE('',#23618,#23683,#1679,.T.) ;
#30818=EDGE_CURVE('',#23684,#23683,#6187,.T.) ;
#30819=EDGE_CURVE('',#23625,#23684,#1680,.T.) ;
#30820=EDGE_CURVE('',#23682,#23684,#19533,.T.) ;
#30821=EDGE_CURVE('',#23685,#23681,#19534,.T.) ;
#30822=EDGE_CURVE('',#23616,#23685,#1681,.T.) ;
#30823=EDGE_CURVE('',#23686,#23685,#6188,.T.) ;
#30824=EDGE_CURVE('',#23627,#23686,#1682,.T.) ;
#30825=EDGE_CURVE('',#23680,#23686,#19535,.T.) ;
#30826=EDGE_CURVE('',#23687,#23679,#19536,.T.) ;
#30827=EDGE_CURVE('',#23614,#23687,#1683,.T.) ;
#30828=EDGE_CURVE('',#23688,#23687,#6189,.T.) ;
#30829=EDGE_CURVE('',#23629,#23688,#1684,.T.) ;
#30830=EDGE_CURVE('',#23678,#23688,#19537,.T.) ;
#30831=EDGE_CURVE('',#23689,#23677,#19538,.T.) ;
#30832=EDGE_CURVE('',#23612,#23689,#1685,.T.) ;
#30833=EDGE_CURVE('',#23690,#23689,#6190,.T.) ;
#30834=EDGE_CURVE('',#23631,#23690,#1686,.T.) ;
#30835=EDGE_CURVE('',#23676,#23690,#19539,.T.) ;
#30836=EDGE_CURVE('',#23691,#23675,#19540,.T.) ;
#30837=EDGE_CURVE('',#23610,#23691,#1687,.T.) ;
#30838=EDGE_CURVE('',#23692,#23691,#6191,.T.) ;
#30839=EDGE_CURVE('',#23633,#23692,#1688,.T.) ;
#30840=EDGE_CURVE('',#23674,#23692,#19541,.T.) ;
#30841=EDGE_CURVE('',#23693,#23673,#19542,.T.) ;
#30842=EDGE_CURVE('',#23608,#23693,#1689,.T.) ;
#30843=EDGE_CURVE('',#23694,#23693,#6192,.T.) ;
#30844=EDGE_CURVE('',#23635,#23694,#1690,.T.) ;
#30845=EDGE_CURVE('',#23672,#23694,#19543,.T.) ;
#30846=EDGE_CURVE('',#23695,#23671,#19544,.T.) ;
#30847=EDGE_CURVE('',#23606,#23695,#1691,.T.) ;
#30848=EDGE_CURVE('',#23696,#23695,#6193,.T.) ;
#30849=EDGE_CURVE('',#23637,#23696,#1692,.T.) ;
#30850=EDGE_CURVE('',#23670,#23696,#19545,.T.) ;
#30851=EDGE_CURVE('',#23697,#23669,#19546,.T.) ;
#30852=EDGE_CURVE('',#23604,#23697,#1693,.T.) ;
#30853=EDGE_CURVE('',#23698,#23697,#6194,.T.) ;
#30854=EDGE_CURVE('',#23639,#23698,#1694,.T.) ;
#30855=EDGE_CURVE('',#23668,#23698,#19547,.T.) ;
#30856=EDGE_CURVE('',#23699,#23667,#19548,.T.) ;
#30857=EDGE_CURVE('',#23602,#23699,#1695,.T.) ;
#30858=EDGE_CURVE('',#23700,#23699,#6195,.T.) ;
#30859=EDGE_CURVE('',#23641,#23700,#1696,.T.) ;
#30860=EDGE_CURVE('',#23665,#23700,#19549,.T.) ;
#30861=EDGE_CURVE('',#23666,#23664,#19550,.T.) ;
#30862=EDGE_CURVE('',#23390,#23663,#6196,.T.) ;
#30863=EDGE_CURVE('',#23662,#23388,#6197,.T.) ;
#30864=EDGE_CURVE('',#23664,#23386,#6198,.T.) ;
#30865=EDGE_CURVE('',#23666,#23384,#6199,.T.) ;
#30866=EDGE_CURVE('',#23683,#23460,#6200,.T.) ;
#30867=EDGE_CURVE('',#23684,#23458,#6201,.T.) ;
#30868=EDGE_CURVE('',#23682,#23456,#6202,.T.) ;
#30869=EDGE_CURVE('',#23454,#23681,#6203,.T.) ;
#30870=EDGE_CURVE('',#23685,#23452,#6204,.T.) ;
#30871=EDGE_CURVE('',#23686,#23450,#6205,.T.) ;
#30872=EDGE_CURVE('',#23680,#23448,#6206,.T.) ;
#30873=EDGE_CURVE('',#23446,#23679,#6207,.T.) ;
#30874=EDGE_CURVE('',#23687,#23444,#6208,.T.) ;
#30875=EDGE_CURVE('',#23688,#23442,#6209,.T.) ;
#30876=EDGE_CURVE('',#23678,#23440,#6210,.T.) ;
#30877=EDGE_CURVE('',#23438,#23677,#6211,.T.) ;
#30878=EDGE_CURVE('',#23689,#23436,#6212,.T.) ;
#30879=EDGE_CURVE('',#23690,#23434,#6213,.T.) ;
#30880=EDGE_CURVE('',#23676,#23432,#6214,.T.) ;
#30881=EDGE_CURVE('',#23430,#23675,#6215,.T.) ;
#30882=EDGE_CURVE('',#23691,#23428,#6216,.T.) ;
#30883=EDGE_CURVE('',#23692,#23426,#6217,.T.) ;
#30884=EDGE_CURVE('',#23674,#23424,#6218,.T.) ;
#30885=EDGE_CURVE('',#23422,#23673,#6219,.T.) ;
#30886=EDGE_CURVE('',#23693,#23420,#6220,.T.) ;
#30887=EDGE_CURVE('',#23694,#23418,#6221,.T.) ;
#30888=EDGE_CURVE('',#23672,#23416,#6222,.T.) ;
#30889=EDGE_CURVE('',#23414,#23671,#6223,.T.) ;
#30890=EDGE_CURVE('',#23695,#23412,#6224,.T.) ;
#30891=EDGE_CURVE('',#23696,#23410,#6225,.T.) ;
#30892=EDGE_CURVE('',#23670,#23408,#6226,.T.) ;
#30893=EDGE_CURVE('',#23406,#23669,#6227,.T.) ;
#30894=EDGE_CURVE('',#23697,#23404,#6228,.T.) ;
#30895=EDGE_CURVE('',#23698,#23402,#6229,.T.) ;
#30896=EDGE_CURVE('',#23668,#23400,#6230,.T.) ;
#30897=EDGE_CURVE('',#23398,#23667,#6231,.T.) ;
#30898=EDGE_CURVE('',#23699,#23396,#6232,.T.) ;
#30899=EDGE_CURVE('',#23700,#23394,#6233,.T.) ;
#30900=EDGE_CURVE('',#23665,#23392,#6234,.T.) ;
#30901=EDGE_CURVE('',#23373,#23374,#6235,.T.) ;
#44006=ORIENTED_EDGE('',*,*,#30281,.F.) ;
#44007=ORIENTED_EDGE('',*,*,#30282,.T.) ;
#44008=ORIENTED_EDGE('',*,*,#30283,.T.) ;
#44009=ORIENTED_EDGE('',*,*,#30282,.F.) ;
#44010=ORIENTED_EDGE('',*,*,#30284,.F.) ;
#44011=ORIENTED_EDGE('',*,*,#30283,.F.) ;
#44012=ORIENTED_EDGE('',*,*,#30285,.T.) ;
#44013=ORIENTED_EDGE('',*,*,#30286,.T.) ;
#44014=ORIENTED_EDGE('',*,*,#30287,.F.) ;
#44015=ORIENTED_EDGE('',*,*,#30286,.F.) ;
#44016=ORIENTED_EDGE('',*,*,#30288,.F.) ;
#44017=ORIENTED_EDGE('',*,*,#30285,.F.) ;
#44018=ORIENTED_EDGE('',*,*,#30287,.T.) ;
#44019=ORIENTED_EDGE('',*,*,#30289,.T.) ;
#44020=ORIENTED_EDGE('',*,*,#30281,.T.) ;
#44021=ORIENTED_EDGE('',*,*,#30290,.T.) ;
#44022=ORIENTED_EDGE('',*,*,#30291,.T.) ;
#44023=ORIENTED_EDGE('',*,*,#30292,.T.) ;
#44024=ORIENTED_EDGE('',*,*,#30293,.T.) ;
#44025=ORIENTED_EDGE('',*,*,#30291,.F.) ;
#44026=ORIENTED_EDGE('',*,*,#30284,.T.) ;
#44027=ORIENTED_EDGE('',*,*,#30294,.T.) ;
#44028=ORIENTED_EDGE('',*,*,#30295,.T.) ;
#44029=ORIENTED_EDGE('',*,*,#30296,.T.) ;
#44030=ORIENTED_EDGE('',*,*,#30294,.F.) ;
#44031=ORIENTED_EDGE('',*,*,#30288,.T.) ;
#44032=ORIENTED_EDGE('',*,*,#30297,.F.) ;
#44033=ORIENTED_EDGE('',*,*,#30298,.T.) ;
#44034=ORIENTED_EDGE('',*,*,#30299,.T.) ;
#44035=ORIENTED_EDGE('',*,*,#30300,.F.) ;
#44036=ORIENTED_EDGE('',*,*,#30301,.T.) ;
#44037=ORIENTED_EDGE('',*,*,#30302,.T.) ;
#44038=ORIENTED_EDGE('',*,*,#30303,.T.) ;
#44039=ORIENTED_EDGE('',*,*,#30298,.F.) ;
#44040=ORIENTED_EDGE('',*,*,#30304,.T.) ;
#44041=ORIENTED_EDGE('',*,*,#30305,.T.) ;
#44042=ORIENTED_EDGE('',*,*,#30306,.T.) ;
#44043=ORIENTED_EDGE('',*,*,#30302,.F.) ;
#44044=ORIENTED_EDGE('',*,*,#30307,.T.) ;
#44045=ORIENTED_EDGE('',*,*,#30308,.T.) ;
#44046=ORIENTED_EDGE('',*,*,#30309,.T.) ;
#44047=ORIENTED_EDGE('',*,*,#30305,.F.) ;
#44048=ORIENTED_EDGE('',*,*,#30310,.F.) ;
#44049=ORIENTED_EDGE('',*,*,#30311,.T.) ;
#44050=ORIENTED_EDGE('',*,*,#30312,.T.) ;
#44051=ORIENTED_EDGE('',*,*,#30308,.F.) ;
#44052=ORIENTED_EDGE('',*,*,#30313,.T.) ;
#44053=ORIENTED_EDGE('',*,*,#30314,.T.) ;
#44054=ORIENTED_EDGE('',*,*,#30315,.T.) ;
#44055=ORIENTED_EDGE('',*,*,#30311,.F.) ;
#44056=ORIENTED_EDGE('',*,*,#30316,.T.) ;
#44057=ORIENTED_EDGE('',*,*,#30317,.T.) ;
#44058=ORIENTED_EDGE('',*,*,#30318,.T.) ;
#44059=ORIENTED_EDGE('',*,*,#30314,.F.) ;
#44060=ORIENTED_EDGE('',*,*,#30319,.T.) ;
#44061=ORIENTED_EDGE('',*,*,#30320,.T.) ;
#44062=ORIENTED_EDGE('',*,*,#30321,.T.) ;
#44063=ORIENTED_EDGE('',*,*,#30317,.F.) ;
#44064=ORIENTED_EDGE('',*,*,#30322,.F.) ;
#44065=ORIENTED_EDGE('',*,*,#30323,.T.) ;
#44066=ORIENTED_EDGE('',*,*,#30324,.T.) ;
#44067=ORIENTED_EDGE('',*,*,#30320,.F.) ;
#44068=ORIENTED_EDGE('',*,*,#30325,.T.) ;
#44069=ORIENTED_EDGE('',*,*,#30326,.T.) ;
#44070=ORIENTED_EDGE('',*,*,#30327,.T.) ;
#44071=ORIENTED_EDGE('',*,*,#30323,.F.) ;
#44072=ORIENTED_EDGE('',*,*,#30328,.T.) ;
#44073=ORIENTED_EDGE('',*,*,#30329,.T.) ;
#44074=ORIENTED_EDGE('',*,*,#30330,.T.) ;
#44075=ORIENTED_EDGE('',*,*,#30326,.F.) ;
#44076=ORIENTED_EDGE('',*,*,#30331,.T.) ;
#44077=ORIENTED_EDGE('',*,*,#30332,.T.) ;
#44078=ORIENTED_EDGE('',*,*,#30333,.T.) ;
#44079=ORIENTED_EDGE('',*,*,#30329,.F.) ;
#44080=ORIENTED_EDGE('',*,*,#30334,.F.) ;
#44081=ORIENTED_EDGE('',*,*,#30335,.T.) ;
#44082=ORIENTED_EDGE('',*,*,#30336,.T.) ;
#44083=ORIENTED_EDGE('',*,*,#30332,.F.) ;
#44084=ORIENTED_EDGE('',*,*,#30337,.T.) ;
#44085=ORIENTED_EDGE('',*,*,#30338,.T.) ;
#44086=ORIENTED_EDGE('',*,*,#30339,.T.) ;
#44087=ORIENTED_EDGE('',*,*,#30335,.F.) ;
#44088=ORIENTED_EDGE('',*,*,#30340,.T.) ;
#44089=ORIENTED_EDGE('',*,*,#30341,.T.) ;
#44090=ORIENTED_EDGE('',*,*,#30342,.T.) ;
#44091=ORIENTED_EDGE('',*,*,#30338,.F.) ;
#44092=ORIENTED_EDGE('',*,*,#30343,.T.) ;
#44093=ORIENTED_EDGE('',*,*,#30344,.T.) ;
#44094=ORIENTED_EDGE('',*,*,#30345,.T.) ;
#44095=ORIENTED_EDGE('',*,*,#30341,.F.) ;
#44096=ORIENTED_EDGE('',*,*,#30346,.F.) ;
#44097=ORIENTED_EDGE('',*,*,#30347,.T.) ;
#44098=ORIENTED_EDGE('',*,*,#30348,.T.) ;
#44099=ORIENTED_EDGE('',*,*,#30344,.F.) ;
#44100=ORIENTED_EDGE('',*,*,#30349,.T.) ;
#44101=ORIENTED_EDGE('',*,*,#30350,.T.) ;
#44102=ORIENTED_EDGE('',*,*,#30351,.T.) ;
#44103=ORIENTED_EDGE('',*,*,#30347,.F.) ;
#44104=ORIENTED_EDGE('',*,*,#30352,.T.) ;
#44105=ORIENTED_EDGE('',*,*,#30353,.T.) ;
#44106=ORIENTED_EDGE('',*,*,#30354,.T.) ;
#44107=ORIENTED_EDGE('',*,*,#30350,.F.) ;
#44108=ORIENTED_EDGE('',*,*,#30355,.T.) ;
#44109=ORIENTED_EDGE('',*,*,#30356,.T.) ;
#44110=ORIENTED_EDGE('',*,*,#30357,.T.) ;
#44111=ORIENTED_EDGE('',*,*,#30353,.F.) ;
#44112=ORIENTED_EDGE('',*,*,#30358,.F.) ;
#44113=ORIENTED_EDGE('',*,*,#30359,.T.) ;
#44114=ORIENTED_EDGE('',*,*,#30360,.T.) ;
#44115=ORIENTED_EDGE('',*,*,#30356,.F.) ;
#44116=ORIENTED_EDGE('',*,*,#30361,.T.) ;
#44117=ORIENTED_EDGE('',*,*,#30362,.T.) ;
#44118=ORIENTED_EDGE('',*,*,#30363,.T.) ;
#44119=ORIENTED_EDGE('',*,*,#30359,.F.) ;
#44120=ORIENTED_EDGE('',*,*,#30364,.T.) ;
#44121=ORIENTED_EDGE('',*,*,#30365,.T.) ;
#44122=ORIENTED_EDGE('',*,*,#30366,.T.) ;
#44123=ORIENTED_EDGE('',*,*,#30362,.F.) ;
#44124=ORIENTED_EDGE('',*,*,#30367,.T.) ;
#44125=ORIENTED_EDGE('',*,*,#30368,.T.) ;
#44126=ORIENTED_EDGE('',*,*,#30369,.T.) ;
#44127=ORIENTED_EDGE('',*,*,#30365,.F.) ;
#44128=ORIENTED_EDGE('',*,*,#30370,.F.) ;
#44129=ORIENTED_EDGE('',*,*,#30371,.T.) ;
#44130=ORIENTED_EDGE('',*,*,#30372,.T.) ;
#44131=ORIENTED_EDGE('',*,*,#30368,.F.) ;
#44132=ORIENTED_EDGE('',*,*,#30373,.T.) ;
#44133=ORIENTED_EDGE('',*,*,#30374,.T.) ;
#44134=ORIENTED_EDGE('',*,*,#30375,.T.) ;
#44135=ORIENTED_EDGE('',*,*,#30371,.F.) ;
#44136=ORIENTED_EDGE('',*,*,#30376,.T.) ;
#44137=ORIENTED_EDGE('',*,*,#30377,.T.) ;
#44138=ORIENTED_EDGE('',*,*,#30378,.T.) ;
#44139=ORIENTED_EDGE('',*,*,#30374,.F.) ;
#44140=ORIENTED_EDGE('',*,*,#30379,.T.) ;
#44141=ORIENTED_EDGE('',*,*,#30380,.T.) ;
#44142=ORIENTED_EDGE('',*,*,#30381,.T.) ;
#44143=ORIENTED_EDGE('',*,*,#30377,.F.) ;
#44144=ORIENTED_EDGE('',*,*,#30382,.F.) ;
#44145=ORIENTED_EDGE('',*,*,#30383,.T.) ;
#44146=ORIENTED_EDGE('',*,*,#30384,.T.) ;
#44147=ORIENTED_EDGE('',*,*,#30380,.F.) ;
#44148=ORIENTED_EDGE('',*,*,#30385,.T.) ;
#44149=ORIENTED_EDGE('',*,*,#30386,.T.) ;
#44150=ORIENTED_EDGE('',*,*,#30387,.T.) ;
#44151=ORIENTED_EDGE('',*,*,#30383,.F.) ;
#44152=ORIENTED_EDGE('',*,*,#30388,.T.) ;
#44153=ORIENTED_EDGE('',*,*,#30389,.T.) ;
#44154=ORIENTED_EDGE('',*,*,#30390,.T.) ;
#44155=ORIENTED_EDGE('',*,*,#30386,.F.) ;
#44156=ORIENTED_EDGE('',*,*,#30391,.T.) ;
#44157=ORIENTED_EDGE('',*,*,#30392,.T.) ;
#44158=ORIENTED_EDGE('',*,*,#30393,.T.) ;
#44159=ORIENTED_EDGE('',*,*,#30389,.F.) ;
#44160=ORIENTED_EDGE('',*,*,#30394,.F.) ;
#44161=ORIENTED_EDGE('',*,*,#30395,.T.) ;
#44162=ORIENTED_EDGE('',*,*,#30396,.T.) ;
#44163=ORIENTED_EDGE('',*,*,#30392,.F.) ;
#44164=ORIENTED_EDGE('',*,*,#30397,.T.) ;
#44165=ORIENTED_EDGE('',*,*,#30398,.T.) ;
#44166=ORIENTED_EDGE('',*,*,#30399,.T.) ;
#44167=ORIENTED_EDGE('',*,*,#30395,.F.) ;
#44168=ORIENTED_EDGE('',*,*,#30400,.T.) ;
#44169=ORIENTED_EDGE('',*,*,#30401,.T.) ;
#44170=ORIENTED_EDGE('',*,*,#30402,.T.) ;
#44171=ORIENTED_EDGE('',*,*,#30398,.F.) ;
#44172=ORIENTED_EDGE('',*,*,#30403,.T.) ;
#44173=ORIENTED_EDGE('',*,*,#30404,.T.) ;
#44174=ORIENTED_EDGE('',*,*,#30405,.T.) ;
#44175=ORIENTED_EDGE('',*,*,#30401,.F.) ;
#44176=ORIENTED_EDGE('',*,*,#30406,.F.) ;
#44177=ORIENTED_EDGE('',*,*,#30407,.T.) ;
#44178=ORIENTED_EDGE('',*,*,#30408,.T.) ;
#44179=ORIENTED_EDGE('',*,*,#30404,.F.) ;
#44180=ORIENTED_EDGE('',*,*,#30409,.T.) ;
#44181=ORIENTED_EDGE('',*,*,#30410,.T.) ;
#44182=ORIENTED_EDGE('',*,*,#30411,.T.) ;
#44183=ORIENTED_EDGE('',*,*,#30407,.F.) ;
#44184=ORIENTED_EDGE('',*,*,#30412,.T.) ;
#44185=ORIENTED_EDGE('',*,*,#30413,.T.) ;
#44186=ORIENTED_EDGE('',*,*,#30414,.T.) ;
#44187=ORIENTED_EDGE('',*,*,#30410,.F.) ;
#44188=ORIENTED_EDGE('',*,*,#30415,.T.) ;
#44189=ORIENTED_EDGE('',*,*,#30416,.T.) ;
#44190=ORIENTED_EDGE('',*,*,#30417,.T.) ;
#44191=ORIENTED_EDGE('',*,*,#30413,.F.) ;
#44192=ORIENTED_EDGE('',*,*,#30418,.F.) ;
#44193=ORIENTED_EDGE('',*,*,#30419,.T.) ;
#44194=ORIENTED_EDGE('',*,*,#30420,.T.) ;
#44195=ORIENTED_EDGE('',*,*,#30416,.F.) ;
#44196=ORIENTED_EDGE('',*,*,#30421,.T.) ;
#44197=ORIENTED_EDGE('',*,*,#30419,.F.) ;
#44198=ORIENTED_EDGE('',*,*,#30422,.T.) ;
#44199=ORIENTED_EDGE('',*,*,#30423,.T.) ;
#44200=ORIENTED_EDGE('',*,*,#30424,.T.) ;
#44201=ORIENTED_EDGE('',*,*,#30423,.F.) ;
#44202=ORIENTED_EDGE('',*,*,#30425,.T.) ;
#44203=ORIENTED_EDGE('',*,*,#30426,.T.) ;
#44204=ORIENTED_EDGE('',*,*,#30427,.T.) ;
#44205=ORIENTED_EDGE('',*,*,#30426,.F.) ;
#44206=ORIENTED_EDGE('',*,*,#30428,.T.) ;
#44207=ORIENTED_EDGE('',*,*,#30429,.T.) ;
#44208=ORIENTED_EDGE('',*,*,#30430,.T.) ;
#44209=ORIENTED_EDGE('',*,*,#30429,.F.) ;
#44210=ORIENTED_EDGE('',*,*,#30431,.F.) ;
#44211=ORIENTED_EDGE('',*,*,#30432,.T.) ;
#44212=ORIENTED_EDGE('',*,*,#30433,.T.) ;
#44213=ORIENTED_EDGE('',*,*,#30432,.F.) ;
#44214=ORIENTED_EDGE('',*,*,#30434,.T.) ;
#44215=ORIENTED_EDGE('',*,*,#30435,.T.) ;
#44216=ORIENTED_EDGE('',*,*,#30436,.T.) ;
#44217=ORIENTED_EDGE('',*,*,#30435,.F.) ;
#44218=ORIENTED_EDGE('',*,*,#30437,.T.) ;
#44219=ORIENTED_EDGE('',*,*,#30438,.T.) ;
#44220=ORIENTED_EDGE('',*,*,#30439,.T.) ;
#44221=ORIENTED_EDGE('',*,*,#30438,.F.) ;
#44222=ORIENTED_EDGE('',*,*,#30440,.T.) ;
#44223=ORIENTED_EDGE('',*,*,#30441,.T.) ;
#44224=ORIENTED_EDGE('',*,*,#30442,.T.) ;
#44225=ORIENTED_EDGE('',*,*,#30441,.F.) ;
#44226=ORIENTED_EDGE('',*,*,#30443,.F.) ;
#44227=ORIENTED_EDGE('',*,*,#30444,.T.) ;
#44228=ORIENTED_EDGE('',*,*,#30445,.T.) ;
#44229=ORIENTED_EDGE('',*,*,#30444,.F.) ;
#44230=ORIENTED_EDGE('',*,*,#30446,.T.) ;
#44231=ORIENTED_EDGE('',*,*,#30447,.T.) ;
#44232=ORIENTED_EDGE('',*,*,#30448,.T.) ;
#44233=ORIENTED_EDGE('',*,*,#30447,.F.) ;
#44234=ORIENTED_EDGE('',*,*,#30449,.T.) ;
#44235=ORIENTED_EDGE('',*,*,#30450,.T.) ;
#44236=ORIENTED_EDGE('',*,*,#30451,.T.) ;
#44237=ORIENTED_EDGE('',*,*,#30450,.F.) ;
#44238=ORIENTED_EDGE('',*,*,#30452,.T.) ;
#44239=ORIENTED_EDGE('',*,*,#30453,.T.) ;
#44240=ORIENTED_EDGE('',*,*,#30454,.T.) ;
#44241=ORIENTED_EDGE('',*,*,#30453,.F.) ;
#44242=ORIENTED_EDGE('',*,*,#30455,.F.) ;
#44243=ORIENTED_EDGE('',*,*,#30456,.T.) ;
#44244=ORIENTED_EDGE('',*,*,#30457,.T.) ;
#44245=ORIENTED_EDGE('',*,*,#30456,.F.) ;
#44246=ORIENTED_EDGE('',*,*,#30458,.T.) ;
#44247=ORIENTED_EDGE('',*,*,#30459,.T.) ;
#44248=ORIENTED_EDGE('',*,*,#30460,.T.) ;
#44249=ORIENTED_EDGE('',*,*,#30459,.F.) ;
#44250=ORIENTED_EDGE('',*,*,#30461,.T.) ;
#44251=ORIENTED_EDGE('',*,*,#30462,.T.) ;
#44252=ORIENTED_EDGE('',*,*,#30463,.T.) ;
#44253=ORIENTED_EDGE('',*,*,#30462,.F.) ;
#44254=ORIENTED_EDGE('',*,*,#30464,.T.) ;
#44255=ORIENTED_EDGE('',*,*,#30465,.T.) ;
#44256=ORIENTED_EDGE('',*,*,#30466,.T.) ;
#44257=ORIENTED_EDGE('',*,*,#30465,.F.) ;
#44258=ORIENTED_EDGE('',*,*,#30467,.F.) ;
#44259=ORIENTED_EDGE('',*,*,#30468,.T.) ;
#44260=ORIENTED_EDGE('',*,*,#30469,.T.) ;
#44261=ORIENTED_EDGE('',*,*,#30468,.F.) ;
#44262=ORIENTED_EDGE('',*,*,#30470,.T.) ;
#44263=ORIENTED_EDGE('',*,*,#30471,.T.) ;
#44264=ORIENTED_EDGE('',*,*,#30472,.T.) ;
#44265=ORIENTED_EDGE('',*,*,#30471,.F.) ;
#44266=ORIENTED_EDGE('',*,*,#30473,.T.) ;
#44267=ORIENTED_EDGE('',*,*,#30474,.T.) ;
#44268=ORIENTED_EDGE('',*,*,#30475,.T.) ;
#44269=ORIENTED_EDGE('',*,*,#30474,.F.) ;
#44270=ORIENTED_EDGE('',*,*,#30476,.T.) ;
#44271=ORIENTED_EDGE('',*,*,#30477,.T.) ;
#44272=ORIENTED_EDGE('',*,*,#30478,.T.) ;
#44273=ORIENTED_EDGE('',*,*,#30477,.F.) ;
#44274=ORIENTED_EDGE('',*,*,#30479,.F.) ;
#44275=ORIENTED_EDGE('',*,*,#30480,.T.) ;
#44276=ORIENTED_EDGE('',*,*,#30481,.T.) ;
#44277=ORIENTED_EDGE('',*,*,#30480,.F.) ;
#44278=ORIENTED_EDGE('',*,*,#30482,.T.) ;
#44279=ORIENTED_EDGE('',*,*,#30483,.T.) ;
#44280=ORIENTED_EDGE('',*,*,#30484,.T.) ;
#44281=ORIENTED_EDGE('',*,*,#30483,.F.) ;
#44282=ORIENTED_EDGE('',*,*,#30485,.T.) ;
#44283=ORIENTED_EDGE('',*,*,#30486,.T.) ;
#44284=ORIENTED_EDGE('',*,*,#30487,.T.) ;
#44285=ORIENTED_EDGE('',*,*,#30486,.F.) ;
#44286=ORIENTED_EDGE('',*,*,#30488,.T.) ;
#44287=ORIENTED_EDGE('',*,*,#30489,.T.) ;
#44288=ORIENTED_EDGE('',*,*,#30490,.T.) ;
#44289=ORIENTED_EDGE('',*,*,#30489,.F.) ;
#44290=ORIENTED_EDGE('',*,*,#30491,.F.) ;
#44291=ORIENTED_EDGE('',*,*,#30492,.T.) ;
#44292=ORIENTED_EDGE('',*,*,#30493,.T.) ;
#44293=ORIENTED_EDGE('',*,*,#30492,.F.) ;
#44294=ORIENTED_EDGE('',*,*,#30494,.T.) ;
#44295=ORIENTED_EDGE('',*,*,#30495,.T.) ;
#44296=ORIENTED_EDGE('',*,*,#30496,.T.) ;
#44297=ORIENTED_EDGE('',*,*,#30495,.F.) ;
#44298=ORIENTED_EDGE('',*,*,#30497,.T.) ;
#44299=ORIENTED_EDGE('',*,*,#30498,.T.) ;
#44300=ORIENTED_EDGE('',*,*,#30499,.T.) ;
#44301=ORIENTED_EDGE('',*,*,#30498,.F.) ;
#44302=ORIENTED_EDGE('',*,*,#30500,.T.) ;
#44303=ORIENTED_EDGE('',*,*,#30501,.T.) ;
#44304=ORIENTED_EDGE('',*,*,#30502,.T.) ;
#44305=ORIENTED_EDGE('',*,*,#30501,.F.) ;
#44306=ORIENTED_EDGE('',*,*,#30503,.F.) ;
#44307=ORIENTED_EDGE('',*,*,#30504,.T.) ;
#44308=ORIENTED_EDGE('',*,*,#30505,.T.) ;
#44309=ORIENTED_EDGE('',*,*,#30504,.F.) ;
#44310=ORIENTED_EDGE('',*,*,#30506,.T.) ;
#44311=ORIENTED_EDGE('',*,*,#30507,.T.) ;
#44312=ORIENTED_EDGE('',*,*,#30508,.T.) ;
#44313=ORIENTED_EDGE('',*,*,#30507,.F.) ;
#44314=ORIENTED_EDGE('',*,*,#30509,.T.) ;
#44315=ORIENTED_EDGE('',*,*,#30510,.T.) ;
#44316=ORIENTED_EDGE('',*,*,#30511,.T.) ;
#44317=ORIENTED_EDGE('',*,*,#30510,.F.) ;
#44318=ORIENTED_EDGE('',*,*,#30512,.T.) ;
#44319=ORIENTED_EDGE('',*,*,#30513,.T.) ;
#44320=ORIENTED_EDGE('',*,*,#30514,.T.) ;
#44321=ORIENTED_EDGE('',*,*,#30513,.F.) ;
#44322=ORIENTED_EDGE('',*,*,#30515,.F.) ;
#44323=ORIENTED_EDGE('',*,*,#30516,.T.) ;
#44324=ORIENTED_EDGE('',*,*,#30517,.T.) ;
#44325=ORIENTED_EDGE('',*,*,#30516,.F.) ;
#44326=ORIENTED_EDGE('',*,*,#30518,.T.) ;
#44327=ORIENTED_EDGE('',*,*,#30519,.T.) ;
#44328=ORIENTED_EDGE('',*,*,#30520,.T.) ;
#44329=ORIENTED_EDGE('',*,*,#30519,.F.) ;
#44330=ORIENTED_EDGE('',*,*,#30521,.T.) ;
#44331=ORIENTED_EDGE('',*,*,#30522,.T.) ;
#44332=ORIENTED_EDGE('',*,*,#30523,.T.) ;
#44333=ORIENTED_EDGE('',*,*,#30522,.F.) ;
#44334=ORIENTED_EDGE('',*,*,#30524,.T.) ;
#44335=ORIENTED_EDGE('',*,*,#30525,.T.) ;
#44336=ORIENTED_EDGE('',*,*,#30526,.T.) ;
#44337=ORIENTED_EDGE('',*,*,#30525,.F.) ;
#44338=ORIENTED_EDGE('',*,*,#30527,.F.) ;
#44339=ORIENTED_EDGE('',*,*,#30528,.T.) ;
#44340=ORIENTED_EDGE('',*,*,#30529,.T.) ;
#44341=ORIENTED_EDGE('',*,*,#30528,.F.) ;
#44342=ORIENTED_EDGE('',*,*,#30530,.T.) ;
#44343=ORIENTED_EDGE('',*,*,#30531,.T.) ;
#44344=ORIENTED_EDGE('',*,*,#30532,.T.) ;
#44345=ORIENTED_EDGE('',*,*,#30531,.F.) ;
#44346=ORIENTED_EDGE('',*,*,#30533,.T.) ;
#44347=ORIENTED_EDGE('',*,*,#30534,.T.) ;
#44348=ORIENTED_EDGE('',*,*,#30535,.T.) ;
#44349=ORIENTED_EDGE('',*,*,#30534,.F.) ;
#44350=ORIENTED_EDGE('',*,*,#30536,.T.) ;
#44351=ORIENTED_EDGE('',*,*,#30300,.T.) ;
#44352=ORIENTED_EDGE('',*,*,#30421,.F.) ;
#44353=ORIENTED_EDGE('',*,*,#30537,.F.) ;
#44354=ORIENTED_EDGE('',*,*,#30538,.F.) ;
#44355=ORIENTED_EDGE('',*,*,#30539,.F.) ;
#44356=ORIENTED_EDGE('',*,*,#30424,.F.) ;
#44357=ORIENTED_EDGE('',*,*,#30540,.F.) ;
#44358=ORIENTED_EDGE('',*,*,#30541,.F.) ;
#44359=ORIENTED_EDGE('',*,*,#30537,.T.) ;
#44360=ORIENTED_EDGE('',*,*,#30427,.F.) ;
#44361=ORIENTED_EDGE('',*,*,#30542,.F.) ;
#44362=ORIENTED_EDGE('',*,*,#30543,.F.) ;
#44363=ORIENTED_EDGE('',*,*,#30540,.T.) ;
#44364=ORIENTED_EDGE('',*,*,#30430,.F.) ;
#44365=ORIENTED_EDGE('',*,*,#30544,.T.) ;
#44366=ORIENTED_EDGE('',*,*,#30545,.F.) ;
#44367=ORIENTED_EDGE('',*,*,#30542,.T.) ;
#44368=ORIENTED_EDGE('',*,*,#30433,.F.) ;
#44369=ORIENTED_EDGE('',*,*,#30546,.F.) ;
#44370=ORIENTED_EDGE('',*,*,#30547,.F.) ;
#44371=ORIENTED_EDGE('',*,*,#30544,.F.) ;
#44372=ORIENTED_EDGE('',*,*,#30436,.F.) ;
#44373=ORIENTED_EDGE('',*,*,#30548,.F.) ;
#44374=ORIENTED_EDGE('',*,*,#30549,.F.) ;
#44375=ORIENTED_EDGE('',*,*,#30546,.T.) ;
#44376=ORIENTED_EDGE('',*,*,#30439,.F.) ;
#44377=ORIENTED_EDGE('',*,*,#30550,.F.) ;
#44378=ORIENTED_EDGE('',*,*,#30551,.F.) ;
#44379=ORIENTED_EDGE('',*,*,#30548,.T.) ;
#44380=ORIENTED_EDGE('',*,*,#30442,.F.) ;
#44381=ORIENTED_EDGE('',*,*,#30552,.T.) ;
#44382=ORIENTED_EDGE('',*,*,#30553,.F.) ;
#44383=ORIENTED_EDGE('',*,*,#30550,.T.) ;
#44384=ORIENTED_EDGE('',*,*,#30445,.F.) ;
#44385=ORIENTED_EDGE('',*,*,#30554,.F.) ;
#44386=ORIENTED_EDGE('',*,*,#30555,.F.) ;
#44387=ORIENTED_EDGE('',*,*,#30552,.F.) ;
#44388=ORIENTED_EDGE('',*,*,#30448,.F.) ;
#44389=ORIENTED_EDGE('',*,*,#30556,.F.) ;
#44390=ORIENTED_EDGE('',*,*,#30557,.F.) ;
#44391=ORIENTED_EDGE('',*,*,#30554,.T.) ;
#44392=ORIENTED_EDGE('',*,*,#30451,.F.) ;
#44393=ORIENTED_EDGE('',*,*,#30558,.F.) ;
#44394=ORIENTED_EDGE('',*,*,#30559,.F.) ;
#44395=ORIENTED_EDGE('',*,*,#30556,.T.) ;
#44396=ORIENTED_EDGE('',*,*,#30454,.F.) ;
#44397=ORIENTED_EDGE('',*,*,#30560,.T.) ;
#44398=ORIENTED_EDGE('',*,*,#30561,.F.) ;
#44399=ORIENTED_EDGE('',*,*,#30558,.T.) ;
#44400=ORIENTED_EDGE('',*,*,#30457,.F.) ;
#44401=ORIENTED_EDGE('',*,*,#30562,.F.) ;
#44402=ORIENTED_EDGE('',*,*,#30563,.F.) ;
#44403=ORIENTED_EDGE('',*,*,#30560,.F.) ;
#44404=ORIENTED_EDGE('',*,*,#30460,.F.) ;
#44405=ORIENTED_EDGE('',*,*,#30564,.F.) ;
#44406=ORIENTED_EDGE('',*,*,#30565,.F.) ;
#44407=ORIENTED_EDGE('',*,*,#30562,.T.) ;
#44408=ORIENTED_EDGE('',*,*,#30463,.F.) ;
#44409=ORIENTED_EDGE('',*,*,#30566,.F.) ;
#44410=ORIENTED_EDGE('',*,*,#30567,.F.) ;
#44411=ORIENTED_EDGE('',*,*,#30564,.T.) ;
#44412=ORIENTED_EDGE('',*,*,#30466,.F.) ;
#44413=ORIENTED_EDGE('',*,*,#30568,.T.) ;
#44414=ORIENTED_EDGE('',*,*,#30569,.F.) ;
#44415=ORIENTED_EDGE('',*,*,#30566,.T.) ;
#44416=ORIENTED_EDGE('',*,*,#30469,.F.) ;
#44417=ORIENTED_EDGE('',*,*,#30570,.F.) ;
#44418=ORIENTED_EDGE('',*,*,#30571,.F.) ;
#44419=ORIENTED_EDGE('',*,*,#30568,.F.) ;
#44420=ORIENTED_EDGE('',*,*,#30472,.F.) ;
#44421=ORIENTED_EDGE('',*,*,#30572,.F.) ;
#44422=ORIENTED_EDGE('',*,*,#30573,.F.) ;
#44423=ORIENTED_EDGE('',*,*,#30570,.T.) ;
#44424=ORIENTED_EDGE('',*,*,#30475,.F.) ;
#44425=ORIENTED_EDGE('',*,*,#30574,.F.) ;
#44426=ORIENTED_EDGE('',*,*,#30575,.F.) ;
#44427=ORIENTED_EDGE('',*,*,#30572,.T.) ;
#44428=ORIENTED_EDGE('',*,*,#30478,.F.) ;
#44429=ORIENTED_EDGE('',*,*,#30576,.T.) ;
#44430=ORIENTED_EDGE('',*,*,#30577,.F.) ;
#44431=ORIENTED_EDGE('',*,*,#30574,.T.) ;
#44432=ORIENTED_EDGE('',*,*,#30481,.F.) ;
#44433=ORIENTED_EDGE('',*,*,#30578,.F.) ;
#44434=ORIENTED_EDGE('',*,*,#30579,.F.) ;
#44435=ORIENTED_EDGE('',*,*,#30576,.F.) ;
#44436=ORIENTED_EDGE('',*,*,#30484,.F.) ;
#44437=ORIENTED_EDGE('',*,*,#30580,.F.) ;
#44438=ORIENTED_EDGE('',*,*,#30581,.F.) ;
#44439=ORIENTED_EDGE('',*,*,#30578,.T.) ;
#44440=ORIENTED_EDGE('',*,*,#30487,.F.) ;
#44441=ORIENTED_EDGE('',*,*,#30582,.F.) ;
#44442=ORIENTED_EDGE('',*,*,#30583,.F.) ;
#44443=ORIENTED_EDGE('',*,*,#30580,.T.) ;
#44444=ORIENTED_EDGE('',*,*,#30490,.F.) ;
#44445=ORIENTED_EDGE('',*,*,#30584,.T.) ;
#44446=ORIENTED_EDGE('',*,*,#30585,.F.) ;
#44447=ORIENTED_EDGE('',*,*,#30582,.T.) ;
#44448=ORIENTED_EDGE('',*,*,#30493,.F.) ;
#44449=ORIENTED_EDGE('',*,*,#30586,.F.) ;
#44450=ORIENTED_EDGE('',*,*,#30587,.F.) ;
#44451=ORIENTED_EDGE('',*,*,#30584,.F.) ;
#44452=ORIENTED_EDGE('',*,*,#30496,.F.) ;
#44453=ORIENTED_EDGE('',*,*,#30588,.F.) ;
#44454=ORIENTED_EDGE('',*,*,#30589,.F.) ;
#44455=ORIENTED_EDGE('',*,*,#30586,.T.) ;
#44456=ORIENTED_EDGE('',*,*,#30499,.F.) ;
#44457=ORIENTED_EDGE('',*,*,#30590,.F.) ;
#44458=ORIENTED_EDGE('',*,*,#30591,.F.) ;
#44459=ORIENTED_EDGE('',*,*,#30588,.T.) ;
#44460=ORIENTED_EDGE('',*,*,#30502,.F.) ;
#44461=ORIENTED_EDGE('',*,*,#30592,.T.) ;
#44462=ORIENTED_EDGE('',*,*,#30593,.F.) ;
#44463=ORIENTED_EDGE('',*,*,#30590,.T.) ;
#44464=ORIENTED_EDGE('',*,*,#30505,.F.) ;
#44465=ORIENTED_EDGE('',*,*,#30594,.F.) ;
#44466=ORIENTED_EDGE('',*,*,#30595,.F.) ;
#44467=ORIENTED_EDGE('',*,*,#30592,.F.) ;
#44468=ORIENTED_EDGE('',*,*,#30508,.F.) ;
#44469=ORIENTED_EDGE('',*,*,#30596,.F.) ;
#44470=ORIENTED_EDGE('',*,*,#30597,.F.) ;
#44471=ORIENTED_EDGE('',*,*,#30594,.T.) ;
#44472=ORIENTED_EDGE('',*,*,#30511,.F.) ;
#44473=ORIENTED_EDGE('',*,*,#30598,.F.) ;
#44474=ORIENTED_EDGE('',*,*,#30599,.F.) ;
#44475=ORIENTED_EDGE('',*,*,#30596,.T.) ;
#44476=ORIENTED_EDGE('',*,*,#30514,.F.) ;
#44477=ORIENTED_EDGE('',*,*,#30600,.T.) ;
#44478=ORIENTED_EDGE('',*,*,#30601,.F.) ;
#44479=ORIENTED_EDGE('',*,*,#30598,.T.) ;
#44480=ORIENTED_EDGE('',*,*,#30517,.F.) ;
#44481=ORIENTED_EDGE('',*,*,#30602,.F.) ;
#44482=ORIENTED_EDGE('',*,*,#30603,.F.) ;
#44483=ORIENTED_EDGE('',*,*,#30600,.F.) ;
#44484=ORIENTED_EDGE('',*,*,#30520,.F.) ;
#44485=ORIENTED_EDGE('',*,*,#30604,.F.) ;
#44486=ORIENTED_EDGE('',*,*,#30605,.F.) ;
#44487=ORIENTED_EDGE('',*,*,#30602,.T.) ;
#44488=ORIENTED_EDGE('',*,*,#30523,.F.) ;
#44489=ORIENTED_EDGE('',*,*,#30606,.F.) ;
#44490=ORIENTED_EDGE('',*,*,#30607,.F.) ;
#44491=ORIENTED_EDGE('',*,*,#30604,.T.) ;
#44492=ORIENTED_EDGE('',*,*,#30526,.F.) ;
#44493=ORIENTED_EDGE('',*,*,#30608,.T.) ;
#44494=ORIENTED_EDGE('',*,*,#30609,.F.) ;
#44495=ORIENTED_EDGE('',*,*,#30606,.T.) ;
#44496=ORIENTED_EDGE('',*,*,#30529,.F.) ;
#44497=ORIENTED_EDGE('',*,*,#30610,.F.) ;
#44498=ORIENTED_EDGE('',*,*,#30611,.F.) ;
#44499=ORIENTED_EDGE('',*,*,#30608,.F.) ;
#44500=ORIENTED_EDGE('',*,*,#30532,.F.) ;
#44501=ORIENTED_EDGE('',*,*,#30612,.F.) ;
#44502=ORIENTED_EDGE('',*,*,#30613,.F.) ;
#44503=ORIENTED_EDGE('',*,*,#30610,.T.) ;
#44504=ORIENTED_EDGE('',*,*,#30535,.F.) ;
#44505=ORIENTED_EDGE('',*,*,#30614,.F.) ;
#44506=ORIENTED_EDGE('',*,*,#30615,.F.) ;
#44507=ORIENTED_EDGE('',*,*,#30612,.T.) ;
#44508=ORIENTED_EDGE('',*,*,#30299,.F.) ;
#44509=ORIENTED_EDGE('',*,*,#30616,.T.) ;
#44510=ORIENTED_EDGE('',*,*,#30617,.F.) ;
#44511=ORIENTED_EDGE('',*,*,#30614,.T.) ;
#44512=ORIENTED_EDGE('',*,*,#30428,.F.) ;
#44513=ORIENTED_EDGE('',*,*,#30425,.F.) ;
#44514=ORIENTED_EDGE('',*,*,#30422,.F.) ;
#44515=ORIENTED_EDGE('',*,*,#30618,.F.) ;
#44516=ORIENTED_EDGE('',*,*,#30440,.F.) ;
#44517=ORIENTED_EDGE('',*,*,#30437,.F.) ;
#44518=ORIENTED_EDGE('',*,*,#30434,.F.) ;
#44519=ORIENTED_EDGE('',*,*,#30619,.F.) ;
#44520=ORIENTED_EDGE('',*,*,#30409,.F.) ;
#44521=ORIENTED_EDGE('',*,*,#30620,.F.) ;
#44522=ORIENTED_EDGE('',*,*,#30415,.F.) ;
#44523=ORIENTED_EDGE('',*,*,#30412,.F.) ;
#44524=ORIENTED_EDGE('',*,*,#30452,.F.) ;
#44525=ORIENTED_EDGE('',*,*,#30449,.F.) ;
#44526=ORIENTED_EDGE('',*,*,#30446,.F.) ;
#44527=ORIENTED_EDGE('',*,*,#30621,.F.) ;
#44528=ORIENTED_EDGE('',*,*,#30397,.F.) ;
#44529=ORIENTED_EDGE('',*,*,#30622,.F.) ;
#44530=ORIENTED_EDGE('',*,*,#30403,.F.) ;
#44531=ORIENTED_EDGE('',*,*,#30400,.F.) ;
#44532=ORIENTED_EDGE('',*,*,#30464,.F.) ;
#44533=ORIENTED_EDGE('',*,*,#30461,.F.) ;
#44534=ORIENTED_EDGE('',*,*,#30458,.F.) ;
#44535=ORIENTED_EDGE('',*,*,#30623,.F.) ;
#44536=ORIENTED_EDGE('',*,*,#30385,.F.) ;
#44537=ORIENTED_EDGE('',*,*,#30624,.F.) ;
#44538=ORIENTED_EDGE('',*,*,#30391,.F.) ;
#44539=ORIENTED_EDGE('',*,*,#30388,.F.) ;
#44540=ORIENTED_EDGE('',*,*,#30476,.F.) ;
#44541=ORIENTED_EDGE('',*,*,#30473,.F.) ;
#44542=ORIENTED_EDGE('',*,*,#30470,.F.) ;
#44543=ORIENTED_EDGE('',*,*,#30625,.F.) ;
#44544=ORIENTED_EDGE('',*,*,#30373,.F.) ;
#44545=ORIENTED_EDGE('',*,*,#30626,.F.) ;
#44546=ORIENTED_EDGE('',*,*,#30379,.F.) ;
#44547=ORIENTED_EDGE('',*,*,#30376,.F.) ;
#44548=ORIENTED_EDGE('',*,*,#30488,.F.) ;
#44549=ORIENTED_EDGE('',*,*,#30485,.F.) ;
#44550=ORIENTED_EDGE('',*,*,#30482,.F.) ;
#44551=ORIENTED_EDGE('',*,*,#30627,.F.) ;
#44552=ORIENTED_EDGE('',*,*,#30361,.F.) ;
#44553=ORIENTED_EDGE('',*,*,#30628,.F.) ;
#44554=ORIENTED_EDGE('',*,*,#30367,.F.) ;
#44555=ORIENTED_EDGE('',*,*,#30364,.F.) ;
#44556=ORIENTED_EDGE('',*,*,#30500,.F.) ;
#44557=ORIENTED_EDGE('',*,*,#30497,.F.) ;
#44558=ORIENTED_EDGE('',*,*,#30494,.F.) ;
#44559=ORIENTED_EDGE('',*,*,#30629,.F.) ;
#44560=ORIENTED_EDGE('',*,*,#30349,.F.) ;
#44561=ORIENTED_EDGE('',*,*,#30630,.F.) ;
#44562=ORIENTED_EDGE('',*,*,#30355,.F.) ;
#44563=ORIENTED_EDGE('',*,*,#30352,.F.) ;
#44564=ORIENTED_EDGE('',*,*,#30512,.F.) ;
#44565=ORIENTED_EDGE('',*,*,#30509,.F.) ;
#44566=ORIENTED_EDGE('',*,*,#30506,.F.) ;
#44567=ORIENTED_EDGE('',*,*,#30631,.F.) ;
#44568=ORIENTED_EDGE('',*,*,#30337,.F.) ;
#44569=ORIENTED_EDGE('',*,*,#30632,.F.) ;
#44570=ORIENTED_EDGE('',*,*,#30343,.F.) ;
#44571=ORIENTED_EDGE('',*,*,#30340,.F.) ;
#44572=ORIENTED_EDGE('',*,*,#30524,.F.) ;
#44573=ORIENTED_EDGE('',*,*,#30521,.F.) ;
#44574=ORIENTED_EDGE('',*,*,#30518,.F.) ;
#44575=ORIENTED_EDGE('',*,*,#30633,.F.) ;
#44576=ORIENTED_EDGE('',*,*,#30325,.F.) ;
#44577=ORIENTED_EDGE('',*,*,#30634,.F.) ;
#44578=ORIENTED_EDGE('',*,*,#30331,.F.) ;
#44579=ORIENTED_EDGE('',*,*,#30328,.F.) ;
#44580=ORIENTED_EDGE('',*,*,#30536,.F.) ;
#44581=ORIENTED_EDGE('',*,*,#30533,.F.) ;
#44582=ORIENTED_EDGE('',*,*,#30530,.F.) ;
#44583=ORIENTED_EDGE('',*,*,#30635,.F.) ;
#44584=ORIENTED_EDGE('',*,*,#30313,.F.) ;
#44585=ORIENTED_EDGE('',*,*,#30636,.F.) ;
#44586=ORIENTED_EDGE('',*,*,#30637,.F.) ;
#44587=ORIENTED_EDGE('',*,*,#30319,.F.) ;
#44588=ORIENTED_EDGE('',*,*,#30316,.F.) ;
#44589=ORIENTED_EDGE('',*,*,#30292,.F.) ;
#44590=ORIENTED_EDGE('',*,*,#30293,.F.) ;
#44591=ORIENTED_EDGE('',*,*,#30638,.T.) ;
#44592=ORIENTED_EDGE('',*,*,#30636,.T.) ;
#44593=ORIENTED_EDGE('',*,*,#30310,.T.) ;
#44594=ORIENTED_EDGE('',*,*,#30639,.T.) ;
#44595=ORIENTED_EDGE('',*,*,#30297,.T.) ;
#44596=ORIENTED_EDGE('',*,*,#30635,.T.) ;
#44597=ORIENTED_EDGE('',*,*,#30527,.T.) ;
#44598=ORIENTED_EDGE('',*,*,#30633,.T.) ;
#44599=ORIENTED_EDGE('',*,*,#30515,.T.) ;
#44600=ORIENTED_EDGE('',*,*,#30631,.T.) ;
#44601=ORIENTED_EDGE('',*,*,#30503,.T.) ;
#44602=ORIENTED_EDGE('',*,*,#30629,.T.) ;
#44603=ORIENTED_EDGE('',*,*,#30491,.T.) ;
#44604=ORIENTED_EDGE('',*,*,#30627,.T.) ;
#44605=ORIENTED_EDGE('',*,*,#30479,.T.) ;
#44606=ORIENTED_EDGE('',*,*,#30625,.T.) ;
#44607=ORIENTED_EDGE('',*,*,#30467,.T.) ;
#44608=ORIENTED_EDGE('',*,*,#30623,.T.) ;
#44609=ORIENTED_EDGE('',*,*,#30455,.T.) ;
#44610=ORIENTED_EDGE('',*,*,#30621,.T.) ;
#44611=ORIENTED_EDGE('',*,*,#30443,.T.) ;
#44612=ORIENTED_EDGE('',*,*,#30619,.T.) ;
#44613=ORIENTED_EDGE('',*,*,#30431,.T.) ;
#44614=ORIENTED_EDGE('',*,*,#30618,.T.) ;
#44615=ORIENTED_EDGE('',*,*,#30418,.T.) ;
#44616=ORIENTED_EDGE('',*,*,#30620,.T.) ;
#44617=ORIENTED_EDGE('',*,*,#30406,.T.) ;
#44618=ORIENTED_EDGE('',*,*,#30622,.T.) ;
#44619=ORIENTED_EDGE('',*,*,#30394,.T.) ;
#44620=ORIENTED_EDGE('',*,*,#30624,.T.) ;
#44621=ORIENTED_EDGE('',*,*,#30382,.T.) ;
#44622=ORIENTED_EDGE('',*,*,#30626,.T.) ;
#44623=ORIENTED_EDGE('',*,*,#30370,.T.) ;
#44624=ORIENTED_EDGE('',*,*,#30628,.T.) ;
#44625=ORIENTED_EDGE('',*,*,#30358,.T.) ;
#44626=ORIENTED_EDGE('',*,*,#30630,.T.) ;
#44627=ORIENTED_EDGE('',*,*,#30346,.T.) ;
#44628=ORIENTED_EDGE('',*,*,#30632,.T.) ;
#44629=ORIENTED_EDGE('',*,*,#30334,.T.) ;
#44630=ORIENTED_EDGE('',*,*,#30634,.T.) ;
#44631=ORIENTED_EDGE('',*,*,#30322,.T.) ;
#44632=ORIENTED_EDGE('',*,*,#30637,.T.) ;
#44633=ORIENTED_EDGE('',*,*,#30638,.F.) ;
#44634=ORIENTED_EDGE('',*,*,#30301,.F.) ;
#44635=ORIENTED_EDGE('',*,*,#30639,.F.) ;
#44636=ORIENTED_EDGE('',*,*,#30307,.F.) ;
#44637=ORIENTED_EDGE('',*,*,#30304,.F.) ;
#44638=ORIENTED_EDGE('',*,*,#30295,.F.) ;
#44639=ORIENTED_EDGE('',*,*,#30296,.F.) ;
#44640=ORIENTED_EDGE('',*,*,#30640,.T.) ;
#44641=ORIENTED_EDGE('',*,*,#30641,.T.) ;
#44642=ORIENTED_EDGE('',*,*,#30642,.F.) ;
#44643=ORIENTED_EDGE('',*,*,#30643,.T.) ;
#44644=ORIENTED_EDGE('',*,*,#30644,.F.) ;
#44645=ORIENTED_EDGE('',*,*,#30645,.T.) ;
#44646=ORIENTED_EDGE('',*,*,#30646,.F.) ;
#44647=ORIENTED_EDGE('',*,*,#30647,.T.) ;
#44648=ORIENTED_EDGE('',*,*,#30648,.F.) ;
#44649=ORIENTED_EDGE('',*,*,#30649,.T.) ;
#44650=ORIENTED_EDGE('',*,*,#30650,.F.) ;
#44651=ORIENTED_EDGE('',*,*,#30651,.T.) ;
#44652=ORIENTED_EDGE('',*,*,#30652,.F.) ;
#44653=ORIENTED_EDGE('',*,*,#30653,.T.) ;
#44654=ORIENTED_EDGE('',*,*,#30654,.F.) ;
#44655=ORIENTED_EDGE('',*,*,#30655,.T.) ;
#44656=ORIENTED_EDGE('',*,*,#30656,.F.) ;
#44657=ORIENTED_EDGE('',*,*,#30657,.T.) ;
#44658=ORIENTED_EDGE('',*,*,#30658,.F.) ;
#44659=ORIENTED_EDGE('',*,*,#30659,.T.) ;
#44660=ORIENTED_EDGE('',*,*,#30660,.F.) ;
#44661=ORIENTED_EDGE('',*,*,#30661,.T.) ;
#44662=ORIENTED_EDGE('',*,*,#30662,.F.) ;
#44663=ORIENTED_EDGE('',*,*,#30663,.T.) ;
#44664=ORIENTED_EDGE('',*,*,#30664,.F.) ;
#44665=ORIENTED_EDGE('',*,*,#30665,.T.) ;
#44666=ORIENTED_EDGE('',*,*,#30666,.F.) ;
#44667=ORIENTED_EDGE('',*,*,#30667,.T.) ;
#44668=ORIENTED_EDGE('',*,*,#30668,.F.) ;
#44669=ORIENTED_EDGE('',*,*,#30669,.T.) ;
#44670=ORIENTED_EDGE('',*,*,#30670,.F.) ;
#44671=ORIENTED_EDGE('',*,*,#30671,.T.) ;
#44672=ORIENTED_EDGE('',*,*,#30672,.F.) ;
#44673=ORIENTED_EDGE('',*,*,#30673,.T.) ;
#44674=ORIENTED_EDGE('',*,*,#30674,.F.) ;
#44675=ORIENTED_EDGE('',*,*,#30675,.T.) ;
#44676=ORIENTED_EDGE('',*,*,#30676,.F.) ;
#44677=ORIENTED_EDGE('',*,*,#30677,.T.) ;
#44678=ORIENTED_EDGE('',*,*,#30678,.F.) ;
#44679=ORIENTED_EDGE('',*,*,#30679,.T.) ;
#44680=ORIENTED_EDGE('',*,*,#30680,.F.) ;
#44681=ORIENTED_EDGE('',*,*,#30681,.T.) ;
#44682=ORIENTED_EDGE('',*,*,#30640,.F.) ;
#44683=ORIENTED_EDGE('',*,*,#30679,.F.) ;
#44684=ORIENTED_EDGE('',*,*,#30682,.F.) ;
#44685=ORIENTED_EDGE('',*,*,#30683,.F.) ;
#44686=ORIENTED_EDGE('',*,*,#30684,.F.) ;
#44687=ORIENTED_EDGE('',*,*,#30677,.F.) ;
#44688=ORIENTED_EDGE('',*,*,#30685,.F.) ;
#44689=ORIENTED_EDGE('',*,*,#30686,.F.) ;
#44690=ORIENTED_EDGE('',*,*,#30687,.F.) ;
#44691=ORIENTED_EDGE('',*,*,#30675,.F.) ;
#44692=ORIENTED_EDGE('',*,*,#30688,.F.) ;
#44693=ORIENTED_EDGE('',*,*,#30689,.F.) ;
#44694=ORIENTED_EDGE('',*,*,#30690,.F.) ;
#44695=ORIENTED_EDGE('',*,*,#30673,.F.) ;
#44696=ORIENTED_EDGE('',*,*,#30691,.F.) ;
#44697=ORIENTED_EDGE('',*,*,#30692,.F.) ;
#44698=ORIENTED_EDGE('',*,*,#30693,.F.) ;
#44699=ORIENTED_EDGE('',*,*,#30671,.F.) ;
#44700=ORIENTED_EDGE('',*,*,#30694,.F.) ;
#44701=ORIENTED_EDGE('',*,*,#30695,.F.) ;
#44702=ORIENTED_EDGE('',*,*,#30696,.F.) ;
#44703=ORIENTED_EDGE('',*,*,#30669,.F.) ;
#44704=ORIENTED_EDGE('',*,*,#30697,.F.) ;
#44705=ORIENTED_EDGE('',*,*,#30698,.F.) ;
#44706=ORIENTED_EDGE('',*,*,#30699,.F.) ;
#44707=ORIENTED_EDGE('',*,*,#30667,.F.) ;
#44708=ORIENTED_EDGE('',*,*,#30700,.F.) ;
#44709=ORIENTED_EDGE('',*,*,#30701,.F.) ;
#44710=ORIENTED_EDGE('',*,*,#30702,.F.) ;
#44711=ORIENTED_EDGE('',*,*,#30665,.F.) ;
#44712=ORIENTED_EDGE('',*,*,#30703,.F.) ;
#44713=ORIENTED_EDGE('',*,*,#30704,.F.) ;
#44714=ORIENTED_EDGE('',*,*,#30705,.F.) ;
#44715=ORIENTED_EDGE('',*,*,#30663,.F.) ;
#44716=ORIENTED_EDGE('',*,*,#30706,.F.) ;
#44717=ORIENTED_EDGE('',*,*,#30707,.F.) ;
#44718=ORIENTED_EDGE('',*,*,#30708,.F.) ;
#44719=ORIENTED_EDGE('',*,*,#30661,.F.) ;
#44720=ORIENTED_EDGE('',*,*,#30709,.F.) ;
#44721=ORIENTED_EDGE('',*,*,#30710,.F.) ;
#44722=ORIENTED_EDGE('',*,*,#30711,.F.) ;
#44723=ORIENTED_EDGE('',*,*,#30659,.F.) ;
#44724=ORIENTED_EDGE('',*,*,#30712,.F.) ;
#44725=ORIENTED_EDGE('',*,*,#30713,.F.) ;
#44726=ORIENTED_EDGE('',*,*,#30714,.F.) ;
#44727=ORIENTED_EDGE('',*,*,#30657,.F.) ;
#44728=ORIENTED_EDGE('',*,*,#30715,.F.) ;
#44729=ORIENTED_EDGE('',*,*,#30716,.F.) ;
#44730=ORIENTED_EDGE('',*,*,#30717,.F.) ;
#44731=ORIENTED_EDGE('',*,*,#30655,.F.) ;
#44732=ORIENTED_EDGE('',*,*,#30718,.F.) ;
#44733=ORIENTED_EDGE('',*,*,#30719,.F.) ;
#44734=ORIENTED_EDGE('',*,*,#30720,.F.) ;
#44735=ORIENTED_EDGE('',*,*,#30653,.F.) ;
#44736=ORIENTED_EDGE('',*,*,#30721,.F.) ;
#44737=ORIENTED_EDGE('',*,*,#30722,.F.) ;
#44738=ORIENTED_EDGE('',*,*,#30723,.F.) ;
#44739=ORIENTED_EDGE('',*,*,#30651,.F.) ;
#44740=ORIENTED_EDGE('',*,*,#30724,.F.) ;
#44741=ORIENTED_EDGE('',*,*,#30725,.F.) ;
#44742=ORIENTED_EDGE('',*,*,#30726,.F.) ;
#44743=ORIENTED_EDGE('',*,*,#30649,.F.) ;
#44744=ORIENTED_EDGE('',*,*,#30727,.F.) ;
#44745=ORIENTED_EDGE('',*,*,#30728,.F.) ;
#44746=ORIENTED_EDGE('',*,*,#30729,.F.) ;
#44747=ORIENTED_EDGE('',*,*,#30647,.F.) ;
#44748=ORIENTED_EDGE('',*,*,#30730,.F.) ;
#44749=ORIENTED_EDGE('',*,*,#30731,.F.) ;
#44750=ORIENTED_EDGE('',*,*,#30732,.F.) ;
#44751=ORIENTED_EDGE('',*,*,#30645,.F.) ;
#44752=ORIENTED_EDGE('',*,*,#30733,.F.) ;
#44753=ORIENTED_EDGE('',*,*,#30734,.F.) ;
#44754=ORIENTED_EDGE('',*,*,#30735,.F.) ;
#44755=ORIENTED_EDGE('',*,*,#30643,.F.) ;
#44756=ORIENTED_EDGE('',*,*,#30736,.F.) ;
#44757=ORIENTED_EDGE('',*,*,#30737,.F.) ;
#44758=ORIENTED_EDGE('',*,*,#30738,.F.) ;
#44759=ORIENTED_EDGE('',*,*,#30681,.F.) ;
#44760=ORIENTED_EDGE('',*,*,#30739,.F.) ;
#44761=ORIENTED_EDGE('',*,*,#30740,.F.) ;
#44762=ORIENTED_EDGE('',*,*,#30741,.F.) ;
#44763=ORIENTED_EDGE('',*,*,#30641,.F.) ;
#44764=ORIENTED_EDGE('',*,*,#30660,.T.) ;
#44765=ORIENTED_EDGE('',*,*,#30742,.T.) ;
#44766=ORIENTED_EDGE('',*,*,#30743,.T.) ;
#44767=ORIENTED_EDGE('',*,*,#30744,.F.) ;
#44768=ORIENTED_EDGE('',*,*,#30714,.T.) ;
#44769=ORIENTED_EDGE('',*,*,#30745,.T.) ;
#44770=ORIENTED_EDGE('',*,*,#30746,.T.) ;
#44771=ORIENTED_EDGE('',*,*,#30742,.F.) ;
#44772=ORIENTED_EDGE('',*,*,#30747,.T.) ;
#44773=ORIENTED_EDGE('',*,*,#30748,.T.) ;
#44774=ORIENTED_EDGE('',*,*,#30709,.T.) ;
#44775=ORIENTED_EDGE('',*,*,#30744,.T.) ;
#44776=ORIENTED_EDGE('',*,*,#30712,.T.) ;
#44777=ORIENTED_EDGE('',*,*,#30749,.T.) ;
#44778=ORIENTED_EDGE('',*,*,#30750,.T.) ;
#44779=ORIENTED_EDGE('',*,*,#30751,.T.) ;
#44780=ORIENTED_EDGE('',*,*,#30658,.T.) ;
#44781=ORIENTED_EDGE('',*,*,#30752,.T.) ;
#44782=ORIENTED_EDGE('',*,*,#30617,.T.) ;
#44783=ORIENTED_EDGE('',*,*,#30749,.F.) ;
#44784=ORIENTED_EDGE('',*,*,#30717,.T.) ;
#44785=ORIENTED_EDGE('',*,*,#30753,.T.) ;
#44786=ORIENTED_EDGE('',*,*,#30615,.T.) ;
#44787=ORIENTED_EDGE('',*,*,#30752,.F.) ;
#44788=ORIENTED_EDGE('',*,*,#30754,.T.) ;
#44789=ORIENTED_EDGE('',*,*,#30755,.T.) ;
#44790=ORIENTED_EDGE('',*,*,#30706,.T.) ;
#44791=ORIENTED_EDGE('',*,*,#30756,.T.) ;
#44792=ORIENTED_EDGE('',*,*,#30715,.T.) ;
#44793=ORIENTED_EDGE('',*,*,#30757,.T.) ;
#44794=ORIENTED_EDGE('',*,*,#30611,.T.) ;
#44795=ORIENTED_EDGE('',*,*,#30758,.T.) ;
#44796=ORIENTED_EDGE('',*,*,#30656,.T.) ;
#44797=ORIENTED_EDGE('',*,*,#30759,.T.) ;
#44798=ORIENTED_EDGE('',*,*,#30609,.T.) ;
#44799=ORIENTED_EDGE('',*,*,#30757,.F.) ;
#44800=ORIENTED_EDGE('',*,*,#30720,.T.) ;
#44801=ORIENTED_EDGE('',*,*,#30760,.T.) ;
#44802=ORIENTED_EDGE('',*,*,#30607,.T.) ;
#44803=ORIENTED_EDGE('',*,*,#30759,.F.) ;
#44804=ORIENTED_EDGE('',*,*,#30761,.T.) ;
#44805=ORIENTED_EDGE('',*,*,#30762,.T.) ;
#44806=ORIENTED_EDGE('',*,*,#30703,.T.) ;
#44807=ORIENTED_EDGE('',*,*,#30763,.T.) ;
#44808=ORIENTED_EDGE('',*,*,#30718,.T.) ;
#44809=ORIENTED_EDGE('',*,*,#30764,.T.) ;
#44810=ORIENTED_EDGE('',*,*,#30603,.T.) ;
#44811=ORIENTED_EDGE('',*,*,#30765,.T.) ;
#44812=ORIENTED_EDGE('',*,*,#30654,.T.) ;
#44813=ORIENTED_EDGE('',*,*,#30766,.T.) ;
#44814=ORIENTED_EDGE('',*,*,#30601,.T.) ;
#44815=ORIENTED_EDGE('',*,*,#30764,.F.) ;
#44816=ORIENTED_EDGE('',*,*,#30723,.T.) ;
#44817=ORIENTED_EDGE('',*,*,#30767,.T.) ;
#44818=ORIENTED_EDGE('',*,*,#30599,.T.) ;
#44819=ORIENTED_EDGE('',*,*,#30766,.F.) ;
#44820=ORIENTED_EDGE('',*,*,#30768,.T.) ;
#44821=ORIENTED_EDGE('',*,*,#30769,.T.) ;
#44822=ORIENTED_EDGE('',*,*,#30700,.T.) ;
#44823=ORIENTED_EDGE('',*,*,#30770,.T.) ;
#44824=ORIENTED_EDGE('',*,*,#30721,.T.) ;
#44825=ORIENTED_EDGE('',*,*,#30771,.T.) ;
#44826=ORIENTED_EDGE('',*,*,#30595,.T.) ;
#44827=ORIENTED_EDGE('',*,*,#30772,.T.) ;
#44828=ORIENTED_EDGE('',*,*,#30652,.T.) ;
#44829=ORIENTED_EDGE('',*,*,#30773,.T.) ;
#44830=ORIENTED_EDGE('',*,*,#30593,.T.) ;
#44831=ORIENTED_EDGE('',*,*,#30771,.F.) ;
#44832=ORIENTED_EDGE('',*,*,#30726,.T.) ;
#44833=ORIENTED_EDGE('',*,*,#30774,.T.) ;
#44834=ORIENTED_EDGE('',*,*,#30591,.T.) ;
#44835=ORIENTED_EDGE('',*,*,#30773,.F.) ;
#44836=ORIENTED_EDGE('',*,*,#30775,.T.) ;
#44837=ORIENTED_EDGE('',*,*,#30776,.T.) ;
#44838=ORIENTED_EDGE('',*,*,#30697,.T.) ;
#44839=ORIENTED_EDGE('',*,*,#30777,.T.) ;
#44840=ORIENTED_EDGE('',*,*,#30724,.T.) ;
#44841=ORIENTED_EDGE('',*,*,#30778,.T.) ;
#44842=ORIENTED_EDGE('',*,*,#30587,.T.) ;
#44843=ORIENTED_EDGE('',*,*,#30779,.T.) ;
#44844=ORIENTED_EDGE('',*,*,#30650,.T.) ;
#44845=ORIENTED_EDGE('',*,*,#30780,.T.) ;
#44846=ORIENTED_EDGE('',*,*,#30585,.T.) ;
#44847=ORIENTED_EDGE('',*,*,#30778,.F.) ;
#44848=ORIENTED_EDGE('',*,*,#30729,.T.) ;
#44849=ORIENTED_EDGE('',*,*,#30781,.T.) ;
#44850=ORIENTED_EDGE('',*,*,#30583,.T.) ;
#44851=ORIENTED_EDGE('',*,*,#30780,.F.) ;
#44852=ORIENTED_EDGE('',*,*,#30782,.T.) ;
#44853=ORIENTED_EDGE('',*,*,#30783,.T.) ;
#44854=ORIENTED_EDGE('',*,*,#30694,.T.) ;
#44855=ORIENTED_EDGE('',*,*,#30784,.T.) ;
#44856=ORIENTED_EDGE('',*,*,#30727,.T.) ;
#44857=ORIENTED_EDGE('',*,*,#30785,.T.) ;
#44858=ORIENTED_EDGE('',*,*,#30579,.T.) ;
#44859=ORIENTED_EDGE('',*,*,#30786,.T.) ;
#44860=ORIENTED_EDGE('',*,*,#30648,.T.) ;
#44861=ORIENTED_EDGE('',*,*,#30787,.T.) ;
#44862=ORIENTED_EDGE('',*,*,#30577,.T.) ;
#44863=ORIENTED_EDGE('',*,*,#30785,.F.) ;
#44864=ORIENTED_EDGE('',*,*,#30732,.T.) ;
#44865=ORIENTED_EDGE('',*,*,#30788,.T.) ;
#44866=ORIENTED_EDGE('',*,*,#30575,.T.) ;
#44867=ORIENTED_EDGE('',*,*,#30787,.F.) ;
#44868=ORIENTED_EDGE('',*,*,#30789,.T.) ;
#44869=ORIENTED_EDGE('',*,*,#30790,.T.) ;
#44870=ORIENTED_EDGE('',*,*,#30691,.T.) ;
#44871=ORIENTED_EDGE('',*,*,#30791,.T.) ;
#44872=ORIENTED_EDGE('',*,*,#30730,.T.) ;
#44873=ORIENTED_EDGE('',*,*,#30792,.T.) ;
#44874=ORIENTED_EDGE('',*,*,#30571,.T.) ;
#44875=ORIENTED_EDGE('',*,*,#30793,.T.) ;
#44876=ORIENTED_EDGE('',*,*,#30646,.T.) ;
#44877=ORIENTED_EDGE('',*,*,#30794,.T.) ;
#44878=ORIENTED_EDGE('',*,*,#30569,.T.) ;
#44879=ORIENTED_EDGE('',*,*,#30792,.F.) ;
#44880=ORIENTED_EDGE('',*,*,#30735,.T.) ;
#44881=ORIENTED_EDGE('',*,*,#30795,.T.) ;
#44882=ORIENTED_EDGE('',*,*,#30567,.T.) ;
#44883=ORIENTED_EDGE('',*,*,#30794,.F.) ;
#44884=ORIENTED_EDGE('',*,*,#30796,.T.) ;
#44885=ORIENTED_EDGE('',*,*,#30797,.T.) ;
#44886=ORIENTED_EDGE('',*,*,#30688,.T.) ;
#44887=ORIENTED_EDGE('',*,*,#30798,.T.) ;
#44888=ORIENTED_EDGE('',*,*,#30733,.T.) ;
#44889=ORIENTED_EDGE('',*,*,#30799,.T.) ;
#44890=ORIENTED_EDGE('',*,*,#30563,.T.) ;
#44891=ORIENTED_EDGE('',*,*,#30800,.T.) ;
#44892=ORIENTED_EDGE('',*,*,#30644,.T.) ;
#44893=ORIENTED_EDGE('',*,*,#30801,.T.) ;
#44894=ORIENTED_EDGE('',*,*,#30561,.T.) ;
#44895=ORIENTED_EDGE('',*,*,#30799,.F.) ;
#44896=ORIENTED_EDGE('',*,*,#30738,.T.) ;
#44897=ORIENTED_EDGE('',*,*,#30802,.T.) ;
#44898=ORIENTED_EDGE('',*,*,#30559,.T.) ;
#44899=ORIENTED_EDGE('',*,*,#30801,.F.) ;
#44900=ORIENTED_EDGE('',*,*,#30803,.T.) ;
#44901=ORIENTED_EDGE('',*,*,#30804,.T.) ;
#44902=ORIENTED_EDGE('',*,*,#30685,.T.) ;
#44903=ORIENTED_EDGE('',*,*,#30805,.T.) ;
#44904=ORIENTED_EDGE('',*,*,#30736,.T.) ;
#44905=ORIENTED_EDGE('',*,*,#30806,.T.) ;
#44906=ORIENTED_EDGE('',*,*,#30555,.T.) ;
#44907=ORIENTED_EDGE('',*,*,#30807,.T.) ;
#44908=ORIENTED_EDGE('',*,*,#30642,.T.) ;
#44909=ORIENTED_EDGE('',*,*,#30808,.T.) ;
#44910=ORIENTED_EDGE('',*,*,#30553,.T.) ;
#44911=ORIENTED_EDGE('',*,*,#30806,.F.) ;
#44912=ORIENTED_EDGE('',*,*,#30741,.T.) ;
#44913=ORIENTED_EDGE('',*,*,#30809,.T.) ;
#44914=ORIENTED_EDGE('',*,*,#30551,.T.) ;
#44915=ORIENTED_EDGE('',*,*,#30808,.F.) ;
#44916=ORIENTED_EDGE('',*,*,#30538,.T.) ;
#44917=ORIENTED_EDGE('',*,*,#30810,.T.) ;
#44918=ORIENTED_EDGE('',*,*,#30682,.T.) ;
#44919=ORIENTED_EDGE('',*,*,#30811,.T.) ;
#44920=ORIENTED_EDGE('',*,*,#30739,.T.) ;
#44921=ORIENTED_EDGE('',*,*,#30812,.T.) ;
#44922=ORIENTED_EDGE('',*,*,#30547,.T.) ;
#44923=ORIENTED_EDGE('',*,*,#30813,.T.) ;
#44924=ORIENTED_EDGE('',*,*,#30680,.T.) ;
#44925=ORIENTED_EDGE('',*,*,#30814,.T.) ;
#44926=ORIENTED_EDGE('',*,*,#30545,.T.) ;
#44927=ORIENTED_EDGE('',*,*,#30812,.F.) ;
#44928=ORIENTED_EDGE('',*,*,#30543,.T.) ;
#44929=ORIENTED_EDGE('',*,*,#30814,.F.) ;
#44930=ORIENTED_EDGE('',*,*,#30684,.T.) ;
#44931=ORIENTED_EDGE('',*,*,#30815,.T.) ;
#44932=ORIENTED_EDGE('',*,*,#30541,.T.) ;
#44933=ORIENTED_EDGE('',*,*,#30815,.F.) ;
#44934=ORIENTED_EDGE('',*,*,#30683,.T.) ;
#44935=ORIENTED_EDGE('',*,*,#30810,.F.) ;
#44936=ORIENTED_EDGE('',*,*,#30740,.T.) ;
#44937=ORIENTED_EDGE('',*,*,#30813,.F.) ;
#44938=ORIENTED_EDGE('',*,*,#30549,.T.) ;
#44939=ORIENTED_EDGE('',*,*,#30809,.F.) ;
#44940=ORIENTED_EDGE('',*,*,#30816,.T.) ;
#44941=ORIENTED_EDGE('',*,*,#30811,.F.) ;
#44942=ORIENTED_EDGE('',*,*,#30678,.T.) ;
#44943=ORIENTED_EDGE('',*,*,#30817,.T.) ;
#44944=ORIENTED_EDGE('',*,*,#30818,.T.) ;
#44945=ORIENTED_EDGE('',*,*,#30817,.F.) ;
#44946=ORIENTED_EDGE('',*,*,#30687,.T.) ;
#44947=ORIENTED_EDGE('',*,*,#30819,.T.) ;
#44948=ORIENTED_EDGE('',*,*,#30820,.T.) ;
#44949=ORIENTED_EDGE('',*,*,#30819,.F.) ;
#44950=ORIENTED_EDGE('',*,*,#30686,.T.) ;
#44951=ORIENTED_EDGE('',*,*,#30804,.F.) ;
#44952=ORIENTED_EDGE('',*,*,#30737,.T.) ;
#44953=ORIENTED_EDGE('',*,*,#30807,.F.) ;
#44954=ORIENTED_EDGE('',*,*,#30557,.T.) ;
#44955=ORIENTED_EDGE('',*,*,#30802,.F.) ;
#44956=ORIENTED_EDGE('',*,*,#30821,.T.) ;
#44957=ORIENTED_EDGE('',*,*,#30805,.F.) ;
#44958=ORIENTED_EDGE('',*,*,#30676,.T.) ;
#44959=ORIENTED_EDGE('',*,*,#30822,.T.) ;
#44960=ORIENTED_EDGE('',*,*,#30823,.T.) ;
#44961=ORIENTED_EDGE('',*,*,#30822,.F.) ;
#44962=ORIENTED_EDGE('',*,*,#30690,.T.) ;
#44963=ORIENTED_EDGE('',*,*,#30824,.T.) ;
#44964=ORIENTED_EDGE('',*,*,#30825,.T.) ;
#44965=ORIENTED_EDGE('',*,*,#30824,.F.) ;
#44966=ORIENTED_EDGE('',*,*,#30689,.T.) ;
#44967=ORIENTED_EDGE('',*,*,#30797,.F.) ;
#44968=ORIENTED_EDGE('',*,*,#30734,.T.) ;
#44969=ORIENTED_EDGE('',*,*,#30800,.F.) ;
#44970=ORIENTED_EDGE('',*,*,#30565,.T.) ;
#44971=ORIENTED_EDGE('',*,*,#30795,.F.) ;
#44972=ORIENTED_EDGE('',*,*,#30826,.T.) ;
#44973=ORIENTED_EDGE('',*,*,#30798,.F.) ;
#44974=ORIENTED_EDGE('',*,*,#30674,.T.) ;
#44975=ORIENTED_EDGE('',*,*,#30827,.T.) ;
#44976=ORIENTED_EDGE('',*,*,#30828,.T.) ;
#44977=ORIENTED_EDGE('',*,*,#30827,.F.) ;
#44978=ORIENTED_EDGE('',*,*,#30693,.T.) ;
#44979=ORIENTED_EDGE('',*,*,#30829,.T.) ;
#44980=ORIENTED_EDGE('',*,*,#30830,.T.) ;
#44981=ORIENTED_EDGE('',*,*,#30829,.F.) ;
#44982=ORIENTED_EDGE('',*,*,#30692,.T.) ;
#44983=ORIENTED_EDGE('',*,*,#30790,.F.) ;
#44984=ORIENTED_EDGE('',*,*,#30731,.T.) ;
#44985=ORIENTED_EDGE('',*,*,#30793,.F.) ;
#44986=ORIENTED_EDGE('',*,*,#30573,.T.) ;
#44987=ORIENTED_EDGE('',*,*,#30788,.F.) ;
#44988=ORIENTED_EDGE('',*,*,#30831,.T.) ;
#44989=ORIENTED_EDGE('',*,*,#30791,.F.) ;
#44990=ORIENTED_EDGE('',*,*,#30672,.T.) ;
#44991=ORIENTED_EDGE('',*,*,#30832,.T.) ;
#44992=ORIENTED_EDGE('',*,*,#30833,.T.) ;
#44993=ORIENTED_EDGE('',*,*,#30832,.F.) ;
#44994=ORIENTED_EDGE('',*,*,#30696,.T.) ;
#44995=ORIENTED_EDGE('',*,*,#30834,.T.) ;
#44996=ORIENTED_EDGE('',*,*,#30835,.T.) ;
#44997=ORIENTED_EDGE('',*,*,#30834,.F.) ;
#44998=ORIENTED_EDGE('',*,*,#30695,.T.) ;
#44999=ORIENTED_EDGE('',*,*,#30783,.F.) ;
#45000=ORIENTED_EDGE('',*,*,#30728,.T.) ;
#45001=ORIENTED_EDGE('',*,*,#30786,.F.) ;
#45002=ORIENTED_EDGE('',*,*,#30581,.T.) ;
#45003=ORIENTED_EDGE('',*,*,#30781,.F.) ;
#45004=ORIENTED_EDGE('',*,*,#30836,.T.) ;
#45005=ORIENTED_EDGE('',*,*,#30784,.F.) ;
#45006=ORIENTED_EDGE('',*,*,#30670,.T.) ;
#45007=ORIENTED_EDGE('',*,*,#30837,.T.) ;
#45008=ORIENTED_EDGE('',*,*,#30838,.T.) ;
#45009=ORIENTED_EDGE('',*,*,#30837,.F.) ;
#45010=ORIENTED_EDGE('',*,*,#30699,.T.) ;
#45011=ORIENTED_EDGE('',*,*,#30839,.T.) ;
#45012=ORIENTED_EDGE('',*,*,#30840,.T.) ;
#45013=ORIENTED_EDGE('',*,*,#30839,.F.) ;
#45014=ORIENTED_EDGE('',*,*,#30698,.T.) ;
#45015=ORIENTED_EDGE('',*,*,#30776,.F.) ;
#45016=ORIENTED_EDGE('',*,*,#30725,.T.) ;
#45017=ORIENTED_EDGE('',*,*,#30779,.F.) ;
#45018=ORIENTED_EDGE('',*,*,#30589,.T.) ;
#45019=ORIENTED_EDGE('',*,*,#30774,.F.) ;
#45020=ORIENTED_EDGE('',*,*,#30841,.T.) ;
#45021=ORIENTED_EDGE('',*,*,#30777,.F.) ;
#45022=ORIENTED_EDGE('',*,*,#30668,.T.) ;
#45023=ORIENTED_EDGE('',*,*,#30842,.T.) ;
#45024=ORIENTED_EDGE('',*,*,#30843,.T.) ;
#45025=ORIENTED_EDGE('',*,*,#30842,.F.) ;
#45026=ORIENTED_EDGE('',*,*,#30702,.T.) ;
#45027=ORIENTED_EDGE('',*,*,#30844,.T.) ;
#45028=ORIENTED_EDGE('',*,*,#30845,.T.) ;
#45029=ORIENTED_EDGE('',*,*,#30844,.F.) ;
#45030=ORIENTED_EDGE('',*,*,#30701,.T.) ;
#45031=ORIENTED_EDGE('',*,*,#30769,.F.) ;
#45032=ORIENTED_EDGE('',*,*,#30722,.T.) ;
#45033=ORIENTED_EDGE('',*,*,#30772,.F.) ;
#45034=ORIENTED_EDGE('',*,*,#30597,.T.) ;
#45035=ORIENTED_EDGE('',*,*,#30767,.F.) ;
#45036=ORIENTED_EDGE('',*,*,#30846,.T.) ;
#45037=ORIENTED_EDGE('',*,*,#30770,.F.) ;
#45038=ORIENTED_EDGE('',*,*,#30666,.T.) ;
#45039=ORIENTED_EDGE('',*,*,#30847,.T.) ;
#45040=ORIENTED_EDGE('',*,*,#30848,.T.) ;
#45041=ORIENTED_EDGE('',*,*,#30847,.F.) ;
#45042=ORIENTED_EDGE('',*,*,#30705,.T.) ;
#45043=ORIENTED_EDGE('',*,*,#30849,.T.) ;
#45044=ORIENTED_EDGE('',*,*,#30850,.T.) ;
#45045=ORIENTED_EDGE('',*,*,#30849,.F.) ;
#45046=ORIENTED_EDGE('',*,*,#30704,.T.) ;
#45047=ORIENTED_EDGE('',*,*,#30762,.F.) ;
#45048=ORIENTED_EDGE('',*,*,#30719,.T.) ;
#45049=ORIENTED_EDGE('',*,*,#30765,.F.) ;
#45050=ORIENTED_EDGE('',*,*,#30605,.T.) ;
#45051=ORIENTED_EDGE('',*,*,#30760,.F.) ;
#45052=ORIENTED_EDGE('',*,*,#30851,.T.) ;
#45053=ORIENTED_EDGE('',*,*,#30763,.F.) ;
#45054=ORIENTED_EDGE('',*,*,#30664,.T.) ;
#45055=ORIENTED_EDGE('',*,*,#30852,.T.) ;
#45056=ORIENTED_EDGE('',*,*,#30853,.T.) ;
#45057=ORIENTED_EDGE('',*,*,#30852,.F.) ;
#45058=ORIENTED_EDGE('',*,*,#30708,.T.) ;
#45059=ORIENTED_EDGE('',*,*,#30854,.T.) ;
#45060=ORIENTED_EDGE('',*,*,#30855,.T.) ;
#45061=ORIENTED_EDGE('',*,*,#30854,.F.) ;
#45062=ORIENTED_EDGE('',*,*,#30707,.T.) ;
#45063=ORIENTED_EDGE('',*,*,#30755,.F.) ;
#45064=ORIENTED_EDGE('',*,*,#30716,.T.) ;
#45065=ORIENTED_EDGE('',*,*,#30758,.F.) ;
#45066=ORIENTED_EDGE('',*,*,#30613,.T.) ;
#45067=ORIENTED_EDGE('',*,*,#30753,.F.) ;
#45068=ORIENTED_EDGE('',*,*,#30856,.T.) ;
#45069=ORIENTED_EDGE('',*,*,#30756,.F.) ;
#45070=ORIENTED_EDGE('',*,*,#30662,.T.) ;
#45071=ORIENTED_EDGE('',*,*,#30857,.T.) ;
#45072=ORIENTED_EDGE('',*,*,#30858,.T.) ;
#45073=ORIENTED_EDGE('',*,*,#30857,.F.) ;
#45074=ORIENTED_EDGE('',*,*,#30711,.T.) ;
#45075=ORIENTED_EDGE('',*,*,#30859,.T.) ;
#45076=ORIENTED_EDGE('',*,*,#30860,.T.) ;
#45077=ORIENTED_EDGE('',*,*,#30859,.F.) ;
#45078=ORIENTED_EDGE('',*,*,#30710,.T.) ;
#45079=ORIENTED_EDGE('',*,*,#30748,.F.) ;
#45080=ORIENTED_EDGE('',*,*,#30713,.T.) ;
#45081=ORIENTED_EDGE('',*,*,#30751,.F.) ;
#45082=ORIENTED_EDGE('',*,*,#30861,.T.) ;
#45083=ORIENTED_EDGE('',*,*,#30745,.F.) ;
#45084=ORIENTED_EDGE('',*,*,#30312,.F.) ;
#45085=ORIENTED_EDGE('',*,*,#30862,.T.) ;
#45086=ORIENTED_EDGE('',*,*,#30743,.F.) ;
#45087=ORIENTED_EDGE('',*,*,#30863,.T.) ;
#45088=ORIENTED_EDGE('',*,*,#30309,.F.) ;
#45089=ORIENTED_EDGE('',*,*,#30863,.F.) ;
#45090=ORIENTED_EDGE('',*,*,#30746,.F.) ;
#45091=ORIENTED_EDGE('',*,*,#30864,.T.) ;
#45092=ORIENTED_EDGE('',*,*,#30306,.F.) ;
#45093=ORIENTED_EDGE('',*,*,#30864,.F.) ;
#45094=ORIENTED_EDGE('',*,*,#30861,.F.) ;
#45095=ORIENTED_EDGE('',*,*,#30865,.T.) ;
#45096=ORIENTED_EDGE('',*,*,#30303,.F.) ;
#45097=ORIENTED_EDGE('',*,*,#30865,.F.) ;
#45098=ORIENTED_EDGE('',*,*,#30750,.F.) ;
#45099=ORIENTED_EDGE('',*,*,#30616,.F.) ;
#45100=ORIENTED_EDGE('',*,*,#30417,.F.) ;
#45101=ORIENTED_EDGE('',*,*,#30866,.F.) ;
#45102=ORIENTED_EDGE('',*,*,#30818,.F.) ;
#45103=ORIENTED_EDGE('',*,*,#30867,.T.) ;
#45104=ORIENTED_EDGE('',*,*,#30411,.F.) ;
#45105=ORIENTED_EDGE('',*,*,#30868,.F.) ;
#45106=ORIENTED_EDGE('',*,*,#30803,.F.) ;
#45107=ORIENTED_EDGE('',*,*,#30869,.F.) ;
#45108=ORIENTED_EDGE('',*,*,#30414,.F.) ;
#45109=ORIENTED_EDGE('',*,*,#30867,.F.) ;
#45110=ORIENTED_EDGE('',*,*,#30820,.F.) ;
#45111=ORIENTED_EDGE('',*,*,#30868,.T.) ;
#45112=ORIENTED_EDGE('',*,*,#30405,.F.) ;
#45113=ORIENTED_EDGE('',*,*,#30870,.F.) ;
#45114=ORIENTED_EDGE('',*,*,#30823,.F.) ;
#45115=ORIENTED_EDGE('',*,*,#30871,.T.) ;
#45116=ORIENTED_EDGE('',*,*,#30399,.F.) ;
#45117=ORIENTED_EDGE('',*,*,#30872,.F.) ;
#45118=ORIENTED_EDGE('',*,*,#30796,.F.) ;
#45119=ORIENTED_EDGE('',*,*,#30873,.F.) ;
#45120=ORIENTED_EDGE('',*,*,#30402,.F.) ;
#45121=ORIENTED_EDGE('',*,*,#30871,.F.) ;
#45122=ORIENTED_EDGE('',*,*,#30825,.F.) ;
#45123=ORIENTED_EDGE('',*,*,#30872,.T.) ;
#45124=ORIENTED_EDGE('',*,*,#30393,.F.) ;
#45125=ORIENTED_EDGE('',*,*,#30874,.F.) ;
#45126=ORIENTED_EDGE('',*,*,#30828,.F.) ;
#45127=ORIENTED_EDGE('',*,*,#30875,.T.) ;
#45128=ORIENTED_EDGE('',*,*,#30387,.F.) ;
#45129=ORIENTED_EDGE('',*,*,#30876,.F.) ;
#45130=ORIENTED_EDGE('',*,*,#30789,.F.) ;
#45131=ORIENTED_EDGE('',*,*,#30877,.F.) ;
#45132=ORIENTED_EDGE('',*,*,#30390,.F.) ;
#45133=ORIENTED_EDGE('',*,*,#30875,.F.) ;
#45134=ORIENTED_EDGE('',*,*,#30830,.F.) ;
#45135=ORIENTED_EDGE('',*,*,#30876,.T.) ;
#45136=ORIENTED_EDGE('',*,*,#30381,.F.) ;
#45137=ORIENTED_EDGE('',*,*,#30878,.F.) ;
#45138=ORIENTED_EDGE('',*,*,#30833,.F.) ;
#45139=ORIENTED_EDGE('',*,*,#30879,.T.) ;
#45140=ORIENTED_EDGE('',*,*,#30375,.F.) ;
#45141=ORIENTED_EDGE('',*,*,#30880,.F.) ;
#45142=ORIENTED_EDGE('',*,*,#30782,.F.) ;
#45143=ORIENTED_EDGE('',*,*,#30881,.F.) ;
#45144=ORIENTED_EDGE('',*,*,#30378,.F.) ;
#45145=ORIENTED_EDGE('',*,*,#30879,.F.) ;
#45146=ORIENTED_EDGE('',*,*,#30835,.F.) ;
#45147=ORIENTED_EDGE('',*,*,#30880,.T.) ;
#45148=ORIENTED_EDGE('',*,*,#30369,.F.) ;
#45149=ORIENTED_EDGE('',*,*,#30882,.F.) ;
#45150=ORIENTED_EDGE('',*,*,#30838,.F.) ;
#45151=ORIENTED_EDGE('',*,*,#30883,.T.) ;
#45152=ORIENTED_EDGE('',*,*,#30363,.F.) ;
#45153=ORIENTED_EDGE('',*,*,#30884,.F.) ;
#45154=ORIENTED_EDGE('',*,*,#30775,.F.) ;
#45155=ORIENTED_EDGE('',*,*,#30885,.F.) ;
#45156=ORIENTED_EDGE('',*,*,#30366,.F.) ;
#45157=ORIENTED_EDGE('',*,*,#30883,.F.) ;
#45158=ORIENTED_EDGE('',*,*,#30840,.F.) ;
#45159=ORIENTED_EDGE('',*,*,#30884,.T.) ;
#45160=ORIENTED_EDGE('',*,*,#30357,.F.) ;
#45161=ORIENTED_EDGE('',*,*,#30886,.F.) ;
#45162=ORIENTED_EDGE('',*,*,#30843,.F.) ;
#45163=ORIENTED_EDGE('',*,*,#30887,.T.) ;
#45164=ORIENTED_EDGE('',*,*,#30351,.F.) ;
#45165=ORIENTED_EDGE('',*,*,#30888,.F.) ;
#45166=ORIENTED_EDGE('',*,*,#30768,.F.) ;
#45167=ORIENTED_EDGE('',*,*,#30889,.F.) ;
#45168=ORIENTED_EDGE('',*,*,#30354,.F.) ;
#45169=ORIENTED_EDGE('',*,*,#30887,.F.) ;
#45170=ORIENTED_EDGE('',*,*,#30845,.F.) ;
#45171=ORIENTED_EDGE('',*,*,#30888,.T.) ;
#45172=ORIENTED_EDGE('',*,*,#30345,.F.) ;
#45173=ORIENTED_EDGE('',*,*,#30890,.F.) ;
#45174=ORIENTED_EDGE('',*,*,#30848,.F.) ;
#45175=ORIENTED_EDGE('',*,*,#30891,.T.) ;
#45176=ORIENTED_EDGE('',*,*,#30339,.F.) ;
#45177=ORIENTED_EDGE('',*,*,#30892,.F.) ;
#45178=ORIENTED_EDGE('',*,*,#30761,.F.) ;
#45179=ORIENTED_EDGE('',*,*,#30893,.F.) ;
#45180=ORIENTED_EDGE('',*,*,#30342,.F.) ;
#45181=ORIENTED_EDGE('',*,*,#30891,.F.) ;
#45182=ORIENTED_EDGE('',*,*,#30850,.F.) ;
#45183=ORIENTED_EDGE('',*,*,#30892,.T.) ;
#45184=ORIENTED_EDGE('',*,*,#30333,.F.) ;
#45185=ORIENTED_EDGE('',*,*,#30894,.F.) ;
#45186=ORIENTED_EDGE('',*,*,#30853,.F.) ;
#45187=ORIENTED_EDGE('',*,*,#30895,.T.) ;
#45188=ORIENTED_EDGE('',*,*,#30327,.F.) ;
#45189=ORIENTED_EDGE('',*,*,#30896,.F.) ;
#45190=ORIENTED_EDGE('',*,*,#30754,.F.) ;
#45191=ORIENTED_EDGE('',*,*,#30897,.F.) ;
#45192=ORIENTED_EDGE('',*,*,#30330,.F.) ;
#45193=ORIENTED_EDGE('',*,*,#30895,.F.) ;
#45194=ORIENTED_EDGE('',*,*,#30855,.F.) ;
#45195=ORIENTED_EDGE('',*,*,#30896,.T.) ;
#45196=ORIENTED_EDGE('',*,*,#30321,.F.) ;
#45197=ORIENTED_EDGE('',*,*,#30898,.F.) ;
#45198=ORIENTED_EDGE('',*,*,#30858,.F.) ;
#45199=ORIENTED_EDGE('',*,*,#30899,.T.) ;
#45200=ORIENTED_EDGE('',*,*,#30315,.F.) ;
#45201=ORIENTED_EDGE('',*,*,#30900,.F.) ;
#45202=ORIENTED_EDGE('',*,*,#30747,.F.) ;
#45203=ORIENTED_EDGE('',*,*,#30862,.F.) ;
#45204=ORIENTED_EDGE('',*,*,#30318,.F.) ;
#45205=ORIENTED_EDGE('',*,*,#30899,.F.) ;
#45206=ORIENTED_EDGE('',*,*,#30860,.F.) ;
#45207=ORIENTED_EDGE('',*,*,#30900,.T.) ;
#45208=ORIENTED_EDGE('',*,*,#30324,.F.) ;
#45209=ORIENTED_EDGE('',*,*,#30897,.T.) ;
#45210=ORIENTED_EDGE('',*,*,#30856,.F.) ;
#45211=ORIENTED_EDGE('',*,*,#30898,.T.) ;
#45212=ORIENTED_EDGE('',*,*,#30336,.F.) ;
#45213=ORIENTED_EDGE('',*,*,#30893,.T.) ;
#45214=ORIENTED_EDGE('',*,*,#30851,.F.) ;
#45215=ORIENTED_EDGE('',*,*,#30894,.T.) ;
#45216=ORIENTED_EDGE('',*,*,#30348,.F.) ;
#45217=ORIENTED_EDGE('',*,*,#30889,.T.) ;
#45218=ORIENTED_EDGE('',*,*,#30846,.F.) ;
#45219=ORIENTED_EDGE('',*,*,#30890,.T.) ;
#45220=ORIENTED_EDGE('',*,*,#30360,.F.) ;
#45221=ORIENTED_EDGE('',*,*,#30885,.T.) ;
#45222=ORIENTED_EDGE('',*,*,#30841,.F.) ;
#45223=ORIENTED_EDGE('',*,*,#30886,.T.) ;
#45224=ORIENTED_EDGE('',*,*,#30372,.F.) ;
#45225=ORIENTED_EDGE('',*,*,#30881,.T.) ;
#45226=ORIENTED_EDGE('',*,*,#30836,.F.) ;
#45227=ORIENTED_EDGE('',*,*,#30882,.T.) ;
#45228=ORIENTED_EDGE('',*,*,#30384,.F.) ;
#45229=ORIENTED_EDGE('',*,*,#30877,.T.) ;
#45230=ORIENTED_EDGE('',*,*,#30831,.F.) ;
#45231=ORIENTED_EDGE('',*,*,#30878,.T.) ;
#45232=ORIENTED_EDGE('',*,*,#30396,.F.) ;
#45233=ORIENTED_EDGE('',*,*,#30873,.T.) ;
#45234=ORIENTED_EDGE('',*,*,#30826,.F.) ;
#45235=ORIENTED_EDGE('',*,*,#30874,.T.) ;
#45236=ORIENTED_EDGE('',*,*,#30408,.F.) ;
#45237=ORIENTED_EDGE('',*,*,#30869,.T.) ;
#45238=ORIENTED_EDGE('',*,*,#30821,.F.) ;
#45239=ORIENTED_EDGE('',*,*,#30870,.T.) ;
#45240=ORIENTED_EDGE('',*,*,#30420,.F.) ;
#45241=ORIENTED_EDGE('',*,*,#30539,.T.) ;
#45242=ORIENTED_EDGE('',*,*,#30816,.F.) ;
#45243=ORIENTED_EDGE('',*,*,#30866,.T.) ;
#45244=ORIENTED_EDGE('',*,*,#30289,.F.) ;
#45245=ORIENTED_EDGE('',*,*,#30901,.T.) ;
#45246=ORIENTED_EDGE('',*,*,#30290,.F.) ;
#45247=ORIENTED_EDGE('',*,*,#30901,.F.) ;
#45881=TOROIDAL_SURFACE('',#54545,3.96824583655185,1.) ;
#45882=TOROIDAL_SURFACE('',#54550,4.,1.) ;
#45883=TOROIDAL_SURFACE('',#54559,4.95,0.15) ;
#45884=TOROIDAL_SURFACE('',#54563,0.350000000000003,0.15) ;
#45885=TOROIDAL_SURFACE('',#54567,4.95,0.15) ;
#45886=TOROIDAL_SURFACE('',#54571,0.350000000000003,0.15) ;
#45887=TOROIDAL_SURFACE('',#54575,4.95,0.15) ;
#45888=TOROIDAL_SURFACE('',#54579,0.350000000000003,0.15) ;
#45889=TOROIDAL_SURFACE('',#54583,4.95,0.15) ;
#45890=TOROIDAL_SURFACE('',#54587,0.350000000000003,0.15) ;
#45891=TOROIDAL_SURFACE('',#54591,4.95,0.15) ;
#45892=TOROIDAL_SURFACE('',#54595,0.350000000000003,0.15) ;
#45893=TOROIDAL_SURFACE('',#54599,4.95,0.15) ;
#45894=TOROIDAL_SURFACE('',#54603,0.350000000000003,0.15) ;
#45895=TOROIDAL_SURFACE('',#54607,4.95,0.15) ;
#45896=TOROIDAL_SURFACE('',#54611,0.350000000000003,0.15) ;
#45897=TOROIDAL_SURFACE('',#54615,4.95,0.15) ;
#45898=TOROIDAL_SURFACE('',#54619,0.350000000000003,0.15) ;
#45899=TOROIDAL_SURFACE('',#54623,4.95,0.15) ;
#45900=TOROIDAL_SURFACE('',#54627,0.350000000000003,0.15) ;
#45901=TOROIDAL_SURFACE('',#54631,4.95,0.15) ;
#45902=TOROIDAL_SURFACE('',#54635,0.350000000000003,0.15) ;
#45903=TOROIDAL_SURFACE('',#54639,4.95,0.15) ;
#45904=TOROIDAL_SURFACE('',#54643,0.350000000000003,0.15) ;
#45905=TOROIDAL_SURFACE('',#54647,4.95,0.15) ;
#45906=TOROIDAL_SURFACE('',#54651,0.350000000000003,0.15) ;
#45907=TOROIDAL_SURFACE('',#54655,4.95,0.15) ;
#45908=TOROIDAL_SURFACE('',#54659,0.350000000000003,0.15) ;
#45909=TOROIDAL_SURFACE('',#54663,4.95,0.15) ;
#45910=TOROIDAL_SURFACE('',#54667,0.350000000000003,0.15) ;
#45911=TOROIDAL_SURFACE('',#54671,4.95,0.15) ;
#45912=TOROIDAL_SURFACE('',#54675,0.350000000000003,0.15) ;
#45913=TOROIDAL_SURFACE('',#54679,4.95,0.15) ;
#45914=TOROIDAL_SURFACE('',#54683,0.350000000000003,0.15) ;
#45915=TOROIDAL_SURFACE('',#54687,4.95,0.15) ;
#45916=TOROIDAL_SURFACE('',#54691,0.350000000000003,0.15) ;
#45917=TOROIDAL_SURFACE('',#54695,4.95,0.15) ;
#45918=TOROIDAL_SURFACE('',#54699,0.350000000000003,0.15) ;
#45919=TOROIDAL_SURFACE('',#54703,4.95,0.15) ;
#45920=TOROIDAL_SURFACE('',#54707,0.350000000000003,0.15) ;
#45921=TOROIDAL_SURFACE('',#54711,4.95,0.15) ;
#45922=TOROIDAL_SURFACE('',#54715,0.350000000000003,0.15) ;
#45923=TOROIDAL_SURFACE('',#54818,4.95,0.15) ;
#45924=TOROIDAL_SURFACE('',#54822,4.95,0.15) ;
#45925=TOROIDAL_SURFACE('',#54905,4.95,0.15) ;
#45926=TOROIDAL_SURFACE('',#54910,4.95,0.15) ;
#45927=TOROIDAL_SURFACE('',#54914,4.95,0.15) ;
#45928=TOROIDAL_SURFACE('',#54918,4.95,0.15) ;
#45929=TOROIDAL_SURFACE('',#54922,4.95,0.15) ;
#45930=TOROIDAL_SURFACE('',#54926,4.95,0.15) ;
#45931=TOROIDAL_SURFACE('',#54930,4.95,0.15) ;
#45932=TOROIDAL_SURFACE('',#54934,4.95,0.15) ;
#45933=TOROIDAL_SURFACE('',#54938,4.95,0.15) ;
#45934=TOROIDAL_SURFACE('',#54942,4.95,0.15) ;
#45935=TOROIDAL_SURFACE('',#54946,4.95,0.15) ;
#45936=TOROIDAL_SURFACE('',#54948,0.350000000000003,0.15) ;
#45937=TOROIDAL_SURFACE('',#54949,0.350000000000003,0.15) ;
#45938=TOROIDAL_SURFACE('',#54950,4.95,0.15) ;
#45939=TOROIDAL_SURFACE('',#54953,0.350000000000003,0.15) ;
#45940=TOROIDAL_SURFACE('',#54955,0.350000000000003,0.15) ;
#45941=TOROIDAL_SURFACE('',#54956,4.95,0.15) ;
#45942=TOROIDAL_SURFACE('',#54959,0.350000000000003,0.15) ;
#45943=TOROIDAL_SURFACE('',#54961,0.350000000000003,0.15) ;
#45944=TOROIDAL_SURFACE('',#54962,4.95,0.15) ;
#45945=TOROIDAL_SURFACE('',#54965,0.350000000000003,0.15) ;
#45946=TOROIDAL_SURFACE('',#54967,0.350000000000003,0.15) ;
#45947=TOROIDAL_SURFACE('',#54968,4.95,0.15) ;
#45948=TOROIDAL_SURFACE('',#54971,0.350000000000003,0.15) ;
#45949=TOROIDAL_SURFACE('',#54973,0.350000000000003,0.15) ;
#45950=TOROIDAL_SURFACE('',#54974,4.95,0.15) ;
#45951=TOROIDAL_SURFACE('',#54977,0.350000000000003,0.15) ;
#45952=TOROIDAL_SURFACE('',#54979,0.350000000000003,0.15) ;
#45953=TOROIDAL_SURFACE('',#54980,4.95,0.15) ;
#45954=TOROIDAL_SURFACE('',#54983,0.350000000000003,0.15) ;
#45955=TOROIDAL_SURFACE('',#54985,0.350000000000003,0.15) ;
#45956=TOROIDAL_SURFACE('',#54986,4.95,0.15) ;
#45957=TOROIDAL_SURFACE('',#54989,0.350000000000003,0.15) ;
#45958=TOROIDAL_SURFACE('',#54991,0.350000000000003,0.15) ;
#45959=TOROIDAL_SURFACE('',#54992,4.95,0.15) ;
#45960=TOROIDAL_SURFACE('',#54995,0.350000000000003,0.15) ;
#45961=TOROIDAL_SURFACE('',#54997,0.350000000000003,0.15) ;
#45962=TOROIDAL_SURFACE('',#54998,4.95,0.15) ;
#45963=TOROIDAL_SURFACE('',#55001,0.350000000000003,0.15) ;
#45964=TOROIDAL_SURFACE('',#55003,0.350000000000003,0.15) ;
#48743=ADVANCED_FACE('',(#13525),#45881,.F.) ;
#48744=ADVANCED_FACE('',(#13526,#766),#2942,.F.) ;
#48745=ADVANCED_FACE('',(#13527),#45882,.F.) ;
#48746=ADVANCED_FACE('',(#13528,#767),#2943,.T.) ;
#48747=ADVANCED_FACE('',(#13529,#768),#2944,.T.) ;
#48748=ADVANCED_FACE('',(#13530,#769),#2945,.F.) ;
#48749=ADVANCED_FACE('',(#13531),#2113,.F.) ;
#48750=ADVANCED_FACE('',(#13532),#2114,.F.) ;
#48751=ADVANCED_FACE('',(#13533),#45883,.T.) ;
#48752=ADVANCED_FACE('',(#13534),#10613,.T.) ;
#48753=ADVANCED_FACE('',(#13535),#45884,.T.) ;
#48754=ADVANCED_FACE('',(#13536),#10614,.T.) ;
#48755=ADVANCED_FACE('',(#13537),#45885,.T.) ;
#48756=ADVANCED_FACE('',(#13538),#10615,.T.) ;
#48757=ADVANCED_FACE('',(#13539),#45886,.T.) ;
#48758=ADVANCED_FACE('',(#13540),#10616,.T.) ;
#48759=ADVANCED_FACE('',(#13541),#45887,.T.) ;
#48760=ADVANCED_FACE('',(#13542),#10617,.T.) ;
#48761=ADVANCED_FACE('',(#13543),#45888,.T.) ;
#48762=ADVANCED_FACE('',(#13544),#10618,.T.) ;
#48763=ADVANCED_FACE('',(#13545),#45889,.T.) ;
#48764=ADVANCED_FACE('',(#13546),#10619,.T.) ;
#48765=ADVANCED_FACE('',(#13547),#45890,.T.) ;
#48766=ADVANCED_FACE('',(#13548),#10620,.T.) ;
#48767=ADVANCED_FACE('',(#13549),#45891,.T.) ;
#48768=ADVANCED_FACE('',(#13550),#10621,.T.) ;
#48769=ADVANCED_FACE('',(#13551),#45892,.T.) ;
#48770=ADVANCED_FACE('',(#13552),#10622,.T.) ;
#48771=ADVANCED_FACE('',(#13553),#45893,.T.) ;
#48772=ADVANCED_FACE('',(#13554),#10623,.T.) ;
#48773=ADVANCED_FACE('',(#13555),#45894,.T.) ;
#48774=ADVANCED_FACE('',(#13556),#10624,.T.) ;
#48775=ADVANCED_FACE('',(#13557),#45895,.T.) ;
#48776=ADVANCED_FACE('',(#13558),#10625,.T.) ;
#48777=ADVANCED_FACE('',(#13559),#45896,.T.) ;
#48778=ADVANCED_FACE('',(#13560),#10626,.T.) ;
#48779=ADVANCED_FACE('',(#13561),#45897,.T.) ;
#48780=ADVANCED_FACE('',(#13562),#10627,.T.) ;
#48781=ADVANCED_FACE('',(#13563),#45898,.T.) ;
#48782=ADVANCED_FACE('',(#13564),#10628,.T.) ;
#48783=ADVANCED_FACE('',(#13565),#45899,.T.) ;
#48784=ADVANCED_FACE('',(#13566),#10629,.T.) ;
#48785=ADVANCED_FACE('',(#13567),#45900,.T.) ;
#48786=ADVANCED_FACE('',(#13568),#10630,.T.) ;
#48787=ADVANCED_FACE('',(#13569),#45901,.T.) ;
#48788=ADVANCED_FACE('',(#13570),#10631,.T.) ;
#48789=ADVANCED_FACE('',(#13571),#45902,.T.) ;
#48790=ADVANCED_FACE('',(#13572),#10632,.T.) ;
#48791=ADVANCED_FACE('',(#13573),#45903,.T.) ;
#48792=ADVANCED_FACE('',(#13574),#10633,.T.) ;
#48793=ADVANCED_FACE('',(#13575),#45904,.T.) ;
#48794=ADVANCED_FACE('',(#13576),#10634,.T.) ;
#48795=ADVANCED_FACE('',(#13577),#45905,.T.) ;
#48796=ADVANCED_FACE('',(#13578),#10635,.T.) ;
#48797=ADVANCED_FACE('',(#13579),#45906,.T.) ;
#48798=ADVANCED_FACE('',(#13580),#10636,.T.) ;
#48799=ADVANCED_FACE('',(#13581),#45907,.T.) ;
#48800=ADVANCED_FACE('',(#13582),#10637,.T.) ;
#48801=ADVANCED_FACE('',(#13583),#45908,.T.) ;
#48802=ADVANCED_FACE('',(#13584),#10638,.T.) ;
#48803=ADVANCED_FACE('',(#13585),#45909,.T.) ;
#48804=ADVANCED_FACE('',(#13586),#10639,.T.) ;
#48805=ADVANCED_FACE('',(#13587),#45910,.T.) ;
#48806=ADVANCED_FACE('',(#13588),#10640,.T.) ;
#48807=ADVANCED_FACE('',(#13589),#45911,.T.) ;
#48808=ADVANCED_FACE('',(#13590),#10641,.T.) ;
#48809=ADVANCED_FACE('',(#13591),#45912,.T.) ;
#48810=ADVANCED_FACE('',(#13592),#10642,.T.) ;
#48811=ADVANCED_FACE('',(#13593),#45913,.T.) ;
#48812=ADVANCED_FACE('',(#13594),#10643,.T.) ;
#48813=ADVANCED_FACE('',(#13595),#45914,.T.) ;
#48814=ADVANCED_FACE('',(#13596),#10644,.T.) ;
#48815=ADVANCED_FACE('',(#13597),#45915,.T.) ;
#48816=ADVANCED_FACE('',(#13598),#10645,.T.) ;
#48817=ADVANCED_FACE('',(#13599),#45916,.T.) ;
#48818=ADVANCED_FACE('',(#13600),#10646,.T.) ;
#48819=ADVANCED_FACE('',(#13601),#45917,.T.) ;
#48820=ADVANCED_FACE('',(#13602),#10647,.T.) ;
#48821=ADVANCED_FACE('',(#13603),#45918,.T.) ;
#48822=ADVANCED_FACE('',(#13604),#10648,.T.) ;
#48823=ADVANCED_FACE('',(#13605),#45919,.T.) ;
#48824=ADVANCED_FACE('',(#13606),#10649,.T.) ;
#48825=ADVANCED_FACE('',(#13607),#45920,.T.) ;
#48826=ADVANCED_FACE('',(#13608),#10650,.T.) ;
#48827=ADVANCED_FACE('',(#13609),#45921,.T.) ;
#48828=ADVANCED_FACE('',(#13610),#10651,.T.) ;
#48829=ADVANCED_FACE('',(#13611),#45922,.T.) ;
#48830=ADVANCED_FACE('',(#13612),#10652,.T.) ;
#48831=ADVANCED_FACE('',(#13613),#2946,.T.) ;
#48832=ADVANCED_FACE('',(#13614),#10653,.T.) ;
#48833=ADVANCED_FACE('',(#13615),#2947,.T.) ;
#48834=ADVANCED_FACE('',(#13616),#10654,.T.) ;
#48835=ADVANCED_FACE('',(#13617),#2948,.T.) ;
#48836=ADVANCED_FACE('',(#13618),#10655,.T.) ;
#48837=ADVANCED_FACE('',(#13619),#2949,.T.) ;
#48838=ADVANCED_FACE('',(#13620),#10656,.T.) ;
#48839=ADVANCED_FACE('',(#13621),#2950,.T.) ;
#48840=ADVANCED_FACE('',(#13622),#10657,.T.) ;
#48841=ADVANCED_FACE('',(#13623),#2951,.T.) ;
#48842=ADVANCED_FACE('',(#13624),#10658,.T.) ;
#48843=ADVANCED_FACE('',(#13625),#2952,.T.) ;
#48844=ADVANCED_FACE('',(#13626),#10659,.T.) ;
#48845=ADVANCED_FACE('',(#13627),#2953,.T.) ;
#48846=ADVANCED_FACE('',(#13628),#10660,.T.) ;
#48847=ADVANCED_FACE('',(#13629),#2954,.T.) ;
#48848=ADVANCED_FACE('',(#13630),#10661,.T.) ;
#48849=ADVANCED_FACE('',(#13631),#2955,.T.) ;
#48850=ADVANCED_FACE('',(#13632),#10662,.T.) ;
#48851=ADVANCED_FACE('',(#13633),#2956,.T.) ;
#48852=ADVANCED_FACE('',(#13634),#10663,.T.) ;
#48853=ADVANCED_FACE('',(#13635),#2957,.T.) ;
#48854=ADVANCED_FACE('',(#13636),#10664,.T.) ;
#48855=ADVANCED_FACE('',(#13637),#2958,.T.) ;
#48856=ADVANCED_FACE('',(#13638),#10665,.T.) ;
#48857=ADVANCED_FACE('',(#13639),#2959,.T.) ;
#48858=ADVANCED_FACE('',(#13640),#10666,.T.) ;
#48859=ADVANCED_FACE('',(#13641),#2960,.T.) ;
#48860=ADVANCED_FACE('',(#13642),#10667,.T.) ;
#48861=ADVANCED_FACE('',(#13643),#2961,.T.) ;
#48862=ADVANCED_FACE('',(#13644),#10668,.T.) ;
#48863=ADVANCED_FACE('',(#13645),#2962,.T.) ;
#48864=ADVANCED_FACE('',(#13646),#10669,.T.) ;
#48865=ADVANCED_FACE('',(#13647),#2963,.T.) ;
#48866=ADVANCED_FACE('',(#13648),#10670,.T.) ;
#48867=ADVANCED_FACE('',(#13649),#2964,.T.) ;
#48868=ADVANCED_FACE('',(#13650),#10671,.T.) ;
#48869=ADVANCED_FACE('',(#13651),#2965,.T.) ;
#48870=ADVANCED_FACE('',(#13652),#10672,.T.) ;
#48871=ADVANCED_FACE('',(#13653),#2966,.F.) ;
#48872=ADVANCED_FACE('',(#13654),#2967,.F.) ;
#48873=ADVANCED_FACE('',(#13655),#2968,.F.) ;
#48874=ADVANCED_FACE('',(#13656),#2969,.F.) ;
#48875=ADVANCED_FACE('',(#13657),#2970,.F.) ;
#48876=ADVANCED_FACE('',(#13658),#2971,.F.) ;
#48877=ADVANCED_FACE('',(#13659),#2972,.F.) ;
#48878=ADVANCED_FACE('',(#13660),#2973,.F.) ;
#48879=ADVANCED_FACE('',(#13661),#2974,.F.) ;
#48880=ADVANCED_FACE('',(#13662),#2975,.F.) ;
#48881=ADVANCED_FACE('',(#13663),#2976,.F.) ;
#48882=ADVANCED_FACE('',(#13664),#2977,.F.) ;
#48883=ADVANCED_FACE('',(#13665),#2978,.F.) ;
#48884=ADVANCED_FACE('',(#13666),#2979,.F.) ;
#48885=ADVANCED_FACE('',(#13667),#2980,.F.) ;
#48886=ADVANCED_FACE('',(#13668),#2981,.F.) ;
#48887=ADVANCED_FACE('',(#13669),#2982,.F.) ;
#48888=ADVANCED_FACE('',(#13670),#2983,.F.) ;
#48889=ADVANCED_FACE('',(#13671),#2984,.F.) ;
#48890=ADVANCED_FACE('',(#13672),#45923,.F.) ;
#48891=ADVANCED_FACE('',(#13673),#2985,.F.) ;
#48892=ADVANCED_FACE('',(#13674),#45924,.F.) ;
#48893=ADVANCED_FACE('',(#13675),#2986,.T.) ;
#48894=ADVANCED_FACE('',(#13676),#2987,.T.) ;
#48895=ADVANCED_FACE('',(#13677),#2988,.T.) ;
#48896=ADVANCED_FACE('',(#13678),#2989,.T.) ;
#48897=ADVANCED_FACE('',(#13679),#2990,.T.) ;
#48898=ADVANCED_FACE('',(#13680),#2991,.T.) ;
#48899=ADVANCED_FACE('',(#13681),#2992,.T.) ;
#48900=ADVANCED_FACE('',(#13682),#2993,.T.) ;
#48901=ADVANCED_FACE('',(#13683),#2994,.T.) ;
#48902=ADVANCED_FACE('',(#13684),#2995,.T.) ;
#48903=ADVANCED_FACE('',(#13685),#2996,.T.) ;
#48904=ADVANCED_FACE('',(#13686),#2997,.T.) ;
#48905=ADVANCED_FACE('',(#13687),#2998,.T.) ;
#48906=ADVANCED_FACE('',(#13688),#2999,.T.) ;
#48907=ADVANCED_FACE('',(#13689),#3000,.T.) ;
#48908=ADVANCED_FACE('',(#13690),#3001,.T.) ;
#48909=ADVANCED_FACE('',(#13691),#3002,.T.) ;
#48910=ADVANCED_FACE('',(#13692),#3003,.T.) ;
#48911=ADVANCED_FACE('',(#13693),#3004,.T.) ;
#48912=ADVANCED_FACE('',(#13694),#3005,.T.) ;
#48913=ADVANCED_FACE('',(#13695),#45925,.T.) ;
#48914=ADVANCED_FACE('',(#13696),#10673,.T.) ;
#48915=ADVANCED_FACE('',(#13697),#10674,.T.) ;
#48916=ADVANCED_FACE('',(#13698),#10675,.T.) ;
#48917=ADVANCED_FACE('',(#13699),#45926,.T.) ;
#48918=ADVANCED_FACE('',(#13700),#10676,.T.) ;
#48919=ADVANCED_FACE('',(#13701),#10677,.T.) ;
#48920=ADVANCED_FACE('',(#13702),#10678,.T.) ;
#48921=ADVANCED_FACE('',(#13703),#45927,.T.) ;
#48922=ADVANCED_FACE('',(#13704),#10679,.T.) ;
#48923=ADVANCED_FACE('',(#13705),#10680,.T.) ;
#48924=ADVANCED_FACE('',(#13706),#10681,.T.) ;
#48925=ADVANCED_FACE('',(#13707),#45928,.T.) ;
#48926=ADVANCED_FACE('',(#13708),#10682,.T.) ;
#48927=ADVANCED_FACE('',(#13709),#10683,.T.) ;
#48928=ADVANCED_FACE('',(#13710),#10684,.T.) ;
#48929=ADVANCED_FACE('',(#13711),#45929,.T.) ;
#48930=ADVANCED_FACE('',(#13712),#10685,.T.) ;
#48931=ADVANCED_FACE('',(#13713),#10686,.T.) ;
#48932=ADVANCED_FACE('',(#13714),#10687,.T.) ;
#48933=ADVANCED_FACE('',(#13715),#45930,.T.) ;
#48934=ADVANCED_FACE('',(#13716),#10688,.T.) ;
#48935=ADVANCED_FACE('',(#13717),#10689,.T.) ;
#48936=ADVANCED_FACE('',(#13718),#10690,.T.) ;
#48937=ADVANCED_FACE('',(#13719),#45931,.T.) ;
#48938=ADVANCED_FACE('',(#13720),#10691,.T.) ;
#48939=ADVANCED_FACE('',(#13721),#10692,.T.) ;
#48940=ADVANCED_FACE('',(#13722),#10693,.T.) ;
#48941=ADVANCED_FACE('',(#13723),#45932,.T.) ;
#48942=ADVANCED_FACE('',(#13724),#10694,.T.) ;
#48943=ADVANCED_FACE('',(#13725),#10695,.T.) ;
#48944=ADVANCED_FACE('',(#13726),#10696,.T.) ;
#48945=ADVANCED_FACE('',(#13727),#45933,.T.) ;
#48946=ADVANCED_FACE('',(#13728),#10697,.T.) ;
#48947=ADVANCED_FACE('',(#13729),#10698,.T.) ;
#48948=ADVANCED_FACE('',(#13730),#10699,.T.) ;
#48949=ADVANCED_FACE('',(#13731),#45934,.T.) ;
#48950=ADVANCED_FACE('',(#13732),#10700,.T.) ;
#48951=ADVANCED_FACE('',(#13733),#10701,.T.) ;
#48952=ADVANCED_FACE('',(#13734),#10702,.T.) ;
#48953=ADVANCED_FACE('',(#13735),#45935,.T.) ;
#48954=ADVANCED_FACE('',(#13736),#10703,.T.) ;
#48955=ADVANCED_FACE('',(#13737),#45936,.T.) ;
#48956=ADVANCED_FACE('',(#13738),#45937,.T.) ;
#48957=ADVANCED_FACE('',(#13739),#45938,.T.) ;
#48958=ADVANCED_FACE('',(#13740),#10704,.T.) ;
#48959=ADVANCED_FACE('',(#13741),#45939,.T.) ;
#48960=ADVANCED_FACE('',(#13742),#45940,.T.) ;
#48961=ADVANCED_FACE('',(#13743),#45941,.T.) ;
#48962=ADVANCED_FACE('',(#13744),#10705,.T.) ;
#48963=ADVANCED_FACE('',(#13745),#45942,.T.) ;
#48964=ADVANCED_FACE('',(#13746),#45943,.T.) ;
#48965=ADVANCED_FACE('',(#13747),#45944,.T.) ;
#48966=ADVANCED_FACE('',(#13748),#10706,.T.) ;
#48967=ADVANCED_FACE('',(#13749),#45945,.T.) ;
#48968=ADVANCED_FACE('',(#13750),#45946,.T.) ;
#48969=ADVANCED_FACE('',(#13751),#45947,.T.) ;
#48970=ADVANCED_FACE('',(#13752),#10707,.T.) ;
#48971=ADVANCED_FACE('',(#13753),#45948,.T.) ;
#48972=ADVANCED_FACE('',(#13754),#45949,.T.) ;
#48973=ADVANCED_FACE('',(#13755),#45950,.T.) ;
#48974=ADVANCED_FACE('',(#13756),#10708,.T.) ;
#48975=ADVANCED_FACE('',(#13757),#45951,.T.) ;
#48976=ADVANCED_FACE('',(#13758),#45952,.T.) ;
#48977=ADVANCED_FACE('',(#13759),#45953,.T.) ;
#48978=ADVANCED_FACE('',(#13760),#10709,.T.) ;
#48979=ADVANCED_FACE('',(#13761),#45954,.T.) ;
#48980=ADVANCED_FACE('',(#13762),#45955,.T.) ;
#48981=ADVANCED_FACE('',(#13763),#45956,.T.) ;
#48982=ADVANCED_FACE('',(#13764),#10710,.T.) ;
#48983=ADVANCED_FACE('',(#13765),#45957,.T.) ;
#48984=ADVANCED_FACE('',(#13766),#45958,.T.) ;
#48985=ADVANCED_FACE('',(#13767),#45959,.T.) ;
#48986=ADVANCED_FACE('',(#13768),#10711,.T.) ;
#48987=ADVANCED_FACE('',(#13769),#45960,.T.) ;
#48988=ADVANCED_FACE('',(#13770),#45961,.T.) ;
#48989=ADVANCED_FACE('',(#13771),#45962,.T.) ;
#48990=ADVANCED_FACE('',(#13772),#10712,.T.) ;
#48991=ADVANCED_FACE('',(#13773),#45963,.T.) ;
#48992=ADVANCED_FACE('',(#13774),#45964,.T.) ;
#48993=ADVANCED_FACE('',(#13775),#10713,.T.) ;
#48994=ADVANCED_FACE('',(#13776),#3006,.T.) ;
#48995=ADVANCED_FACE('',(#13777),#10714,.T.) ;
#48996=ADVANCED_FACE('',(#13778),#3007,.T.) ;
#48997=ADVANCED_FACE('',(#13779),#3008,.T.) ;
#48998=ADVANCED_FACE('',(#13780),#3009,.T.) ;
#48999=ADVANCED_FACE('',(#13781),#10715,.T.) ;
#49000=ADVANCED_FACE('',(#13782),#3010,.T.) ;
#49001=ADVANCED_FACE('',(#13783),#3011,.T.) ;
#49002=ADVANCED_FACE('',(#13784),#10716,.T.) ;
#49003=ADVANCED_FACE('',(#13785),#3012,.T.) ;
#49004=ADVANCED_FACE('',(#13786),#3013,.T.) ;
#49005=ADVANCED_FACE('',(#13787),#10717,.T.) ;
#49006=ADVANCED_FACE('',(#13788),#3014,.T.) ;
#49007=ADVANCED_FACE('',(#13789),#3015,.T.) ;
#49008=ADVANCED_FACE('',(#13790),#10718,.T.) ;
#49009=ADVANCED_FACE('',(#13791),#3016,.T.) ;
#49010=ADVANCED_FACE('',(#13792),#3017,.T.) ;
#49011=ADVANCED_FACE('',(#13793),#10719,.T.) ;
#49012=ADVANCED_FACE('',(#13794),#3018,.T.) ;
#49013=ADVANCED_FACE('',(#13795),#3019,.T.) ;
#49014=ADVANCED_FACE('',(#13796),#10720,.T.) ;
#49015=ADVANCED_FACE('',(#13797),#3020,.T.) ;
#49016=ADVANCED_FACE('',(#13798),#3021,.T.) ;
#49017=ADVANCED_FACE('',(#13799),#10721,.T.) ;
#49018=ADVANCED_FACE('',(#13800),#3022,.T.) ;
#49019=ADVANCED_FACE('',(#13801),#3023,.T.) ;
#49020=ADVANCED_FACE('',(#13802),#10722,.T.) ;
#49021=ADVANCED_FACE('',(#13803),#3024,.T.) ;
#49022=ADVANCED_FACE('',(#13804),#3025,.T.) ;
#49023=ADVANCED_FACE('',(#13805),#10723,.T.) ;
#49024=ADVANCED_FACE('',(#13806),#10724,.T.) ;
#49025=ADVANCED_FACE('',(#13807),#10725,.T.) ;
#49026=ADVANCED_FACE('',(#13808),#10726,.T.) ;
#49027=ADVANCED_FACE('',(#13809),#10727,.T.) ;
#49028=ADVANCED_FACE('',(#13810),#10728,.T.) ;
#49029=ADVANCED_FACE('',(#13811),#10729,.T.) ;
#49030=ADVANCED_FACE('',(#13812),#10730,.T.) ;
#49031=ADVANCED_FACE('',(#13813),#10731,.T.) ;
#49032=ADVANCED_FACE('',(#13814),#10732,.T.) ;
#49033=ADVANCED_FACE('',(#13815),#10733,.F.) ;
#49076=CLOSED_SHELL('',(#48743,#48744,#48745,#48746,#48747,#48748,#48749,
#48750,#48751,#48752,#48753,#48754,#48755,#48756,#48757,#48758,#48759,#48760,
#48761,#48762,#48763,#48764,#48765,#48766,#48767,#48768,#48769,#48770,#48771,
#48772,#48773,#48774,#48775,#48776,#48777,#48778,#48779,#48780,#48781,#48782,
#48783,#48784,#48785,#48786,#48787,#48788,#48789,#48790,#48791,#48792,#48793,
#48794,#48795,#48796,#48797,#48798,#48799,#48800,#48801,#48802,#48803,#48804,
#48805,#48806,#48807,#48808,#48809,#48810,#48811,#48812,#48813,#48814,#48815,
#48816,#48817,#48818,#48819,#48820,#48821,#48822,#48823,#48824,#48825,#48826,
#48827,#48828,#48829,#48830,#48831,#48832,#48833,#48834,#48835,#48836,#48837,
#48838,#48839,#48840,#48841,#48842,#48843,#48844,#48845,#48846,#48847,#48848,
#48849,#48850,#48851,#48852,#48853,#48854,#48855,#48856,#48857,#48858,#48859,
#48860,#48861,#48862,#48863,#48864,#48865,#48866,#48867,#48868,#48869,#48870,
#48871,#48872,#48873,#48874,#48875,#48876,#48877,#48878,#48879,#48880,#48881,
#48882,#48883,#48884,#48885,#48886,#48887,#48888,#48889,#48890,#48891,#48892,
#48893,#48894,#48895,#48896,#48897,#48898,#48899,#48900,#48901,#48902,#48903,
#48904,#48905,#48906,#48907,#48908,#48909,#48910,#48911,#48912,#48913,#48914,
#48915,#48916,#48917,#48918,#48919,#48920,#48921,#48922,#48923,#48924,#48925,
#48926,#48927,#48928,#48929,#48930,#48931,#48932,#48933,#48934,#48935,#48936,
#48937,#48938,#48939,#48940,#48941,#48942,#48943,#48944,#48945,#48946,#48947,
#48948,#48949,#48950,#48951,#48952,#48953,#48954,#48955,#48956,#48957,#48958,
#48959,#48960,#48961,#48962,#48963,#48964,#48965,#48966,#48967,#48968,#48969,
#48970,#48971,#48972,#48973,#48974,#48975,#48976,#48977,#48978,#48979,#48980,
#48981,#48982,#48983,#48984,#48985,#48986,#48987,#48988,#48989,#48990,#48991,
#48992,#48993,#48994,#48995,#48996,#48997,#48998,#48999,#49000,#49001,#49002,
#49003,#49004,#49005,#49006,#49007,#49008,#49009,#49010,#49011,#49012,#49013,
#49014,#49015,#49016,#49017,#49018,#49019,#49020,#49021,#49022,#49023,#49024,
#49025,#49026,#49027,#49028,#49029,#49030,#49031,#49032,#49033)) ;
#54544=AXIS2_PLACEMENT_3D('',#105464,#68528,#68529) ;
#54545=AXIS2_PLACEMENT_3D('',#105465,#68530,#68531) ;
#54546=AXIS2_PLACEMENT_3D('',#105467,#68532,#68533) ;
#54547=AXIS2_PLACEMENT_3D('',#105469,#68534,#68535) ;
#54548=AXIS2_PLACEMENT_3D('',#105470,#68536,#68537) ;
#54549=AXIS2_PLACEMENT_3D('',#105471,#68538,#68539) ;
#54550=AXIS2_PLACEMENT_3D('',#105490,#68540,#68541) ;
#54551=AXIS2_PLACEMENT_3D('',#105492,#68542,#68543) ;
#54552=AXIS2_PLACEMENT_3D('',#105494,#68544,#68545) ;
#54553=AXIS2_PLACEMENT_3D('',#105495,#68546,#68547) ;
#54554=AXIS2_PLACEMENT_3D('',#105496,#68548,#68549) ;
#54555=AXIS2_PLACEMENT_3D('',#105515,#68550,#68551) ;
#54556=AXIS2_PLACEMENT_3D('',#105517,#68552,#68553) ;
#54557=AXIS2_PLACEMENT_3D('',#105518,#68554,#68555) ;
#54558=AXIS2_PLACEMENT_3D('',#105520,#68556,#68557) ;
#54559=AXIS2_PLACEMENT_3D('',#105747,#68558,#68559) ;
#54560=AXIS2_PLACEMENT_3D('',#105750,#68560,#68561) ;
#54561=AXIS2_PLACEMENT_3D('',#105767,#68562,#68563) ;
#54562=AXIS2_PLACEMENT_3D('',#105782,#68564,#68565) ;
#54563=AXIS2_PLACEMENT_3D('',#105803,#68568,#68569) ;
#54564=AXIS2_PLACEMENT_3D('',#105805,#68570,#68571) ;
#54565=AXIS2_PLACEMENT_3D('',#105823,#68572,#68573) ;
#54566=AXIS2_PLACEMENT_3D('',#105824,#68574,#68575) ;
#54567=AXIS2_PLACEMENT_3D('',#105843,#68578,#68579) ;
#54568=AXIS2_PLACEMENT_3D('',#105845,#68580,#68581) ;
#54569=AXIS2_PLACEMENT_3D('',#105861,#68582,#68583) ;
#54570=AXIS2_PLACEMENT_3D('',#105862,#68584,#68585) ;
#54571=AXIS2_PLACEMENT_3D('',#105883,#68588,#68589) ;
#54572=AXIS2_PLACEMENT_3D('',#105885,#68590,#68591) ;
#54573=AXIS2_PLACEMENT_3D('',#105903,#68592,#68593) ;
#54574=AXIS2_PLACEMENT_3D('',#105904,#68594,#68595) ;
#54575=AXIS2_PLACEMENT_3D('',#105923,#68598,#68599) ;
#54576=AXIS2_PLACEMENT_3D('',#105925,#68600,#68601) ;
#54577=AXIS2_PLACEMENT_3D('',#105941,#68602,#68603) ;
#54578=AXIS2_PLACEMENT_3D('',#105942,#68604,#68605) ;
#54579=AXIS2_PLACEMENT_3D('',#105963,#68608,#68609) ;
#54580=AXIS2_PLACEMENT_3D('',#105965,#68610,#68611) ;
#54581=AXIS2_PLACEMENT_3D('',#105983,#68612,#68613) ;
#54582=AXIS2_PLACEMENT_3D('',#105984,#68614,#68615) ;
#54583=AXIS2_PLACEMENT_3D('',#106003,#68618,#68619) ;
#54584=AXIS2_PLACEMENT_3D('',#106005,#68620,#68621) ;
#54585=AXIS2_PLACEMENT_3D('',#106021,#68622,#68623) ;
#54586=AXIS2_PLACEMENT_3D('',#106022,#68624,#68625) ;
#54587=AXIS2_PLACEMENT_3D('',#106043,#68628,#68629) ;
#54588=AXIS2_PLACEMENT_3D('',#106045,#68630,#68631) ;
#54589=AXIS2_PLACEMENT_3D('',#106063,#68632,#68633) ;
#54590=AXIS2_PLACEMENT_3D('',#106064,#68634,#68635) ;
#54591=AXIS2_PLACEMENT_3D('',#106083,#68638,#68639) ;
#54592=AXIS2_PLACEMENT_3D('',#106085,#68640,#68641) ;
#54593=AXIS2_PLACEMENT_3D('',#106101,#68642,#68643) ;
#54594=AXIS2_PLACEMENT_3D('',#106102,#68644,#68645) ;
#54595=AXIS2_PLACEMENT_3D('',#106123,#68648,#68649) ;
#54596=AXIS2_PLACEMENT_3D('',#106125,#68650,#68651) ;
#54597=AXIS2_PLACEMENT_3D('',#106143,#68652,#68653) ;
#54598=AXIS2_PLACEMENT_3D('',#106144,#68654,#68655) ;
#54599=AXIS2_PLACEMENT_3D('',#106163,#68658,#68659) ;
#54600=AXIS2_PLACEMENT_3D('',#106165,#68660,#68661) ;
#54601=AXIS2_PLACEMENT_3D('',#106181,#68662,#68663) ;
#54602=AXIS2_PLACEMENT_3D('',#106182,#68664,#68665) ;
#54603=AXIS2_PLACEMENT_3D('',#106203,#68668,#68669) ;
#54604=AXIS2_PLACEMENT_3D('',#106205,#68670,#68671) ;
#54605=AXIS2_PLACEMENT_3D('',#106223,#68672,#68673) ;
#54606=AXIS2_PLACEMENT_3D('',#106224,#68674,#68675) ;
#54607=AXIS2_PLACEMENT_3D('',#106243,#68678,#68679) ;
#54608=AXIS2_PLACEMENT_3D('',#106245,#68680,#68681) ;
#54609=AXIS2_PLACEMENT_3D('',#106261,#68682,#68683) ;
#54610=AXIS2_PLACEMENT_3D('',#106262,#68684,#68685) ;
#54611=AXIS2_PLACEMENT_3D('',#106283,#68688,#68689) ;
#54612=AXIS2_PLACEMENT_3D('',#106285,#68690,#68691) ;
#54613=AXIS2_PLACEMENT_3D('',#106303,#68692,#68693) ;
#54614=AXIS2_PLACEMENT_3D('',#106304,#68694,#68695) ;
#54615=AXIS2_PLACEMENT_3D('',#106323,#68698,#68699) ;
#54616=AXIS2_PLACEMENT_3D('',#106325,#68700,#68701) ;
#54617=AXIS2_PLACEMENT_3D('',#106341,#68702,#68703) ;
#54618=AXIS2_PLACEMENT_3D('',#106342,#68704,#68705) ;
#54619=AXIS2_PLACEMENT_3D('',#106363,#68708,#68709) ;
#54620=AXIS2_PLACEMENT_3D('',#106365,#68710,#68711) ;
#54621=AXIS2_PLACEMENT_3D('',#106383,#68712,#68713) ;
#54622=AXIS2_PLACEMENT_3D('',#106384,#68714,#68715) ;
#54623=AXIS2_PLACEMENT_3D('',#106403,#68718,#68719) ;
#54624=AXIS2_PLACEMENT_3D('',#106405,#68720,#68721) ;
#54625=AXIS2_PLACEMENT_3D('',#106421,#68722,#68723) ;
#54626=AXIS2_PLACEMENT_3D('',#106422,#68724,#68725) ;
#54627=AXIS2_PLACEMENT_3D('',#106443,#68728,#68729) ;
#54628=AXIS2_PLACEMENT_3D('',#106445,#68730,#68731) ;
#54629=AXIS2_PLACEMENT_3D('',#106463,#68732,#68733) ;
#54630=AXIS2_PLACEMENT_3D('',#106464,#68734,#68735) ;
#54631=AXIS2_PLACEMENT_3D('',#106483,#68738,#68739) ;
#54632=AXIS2_PLACEMENT_3D('',#106485,#68740,#68741) ;
#54633=AXIS2_PLACEMENT_3D('',#106501,#68742,#68743) ;
#54634=AXIS2_PLACEMENT_3D('',#106502,#68744,#68745) ;
#54635=AXIS2_PLACEMENT_3D('',#106523,#68748,#68749) ;
#54636=AXIS2_PLACEMENT_3D('',#106525,#68750,#68751) ;
#54637=AXIS2_PLACEMENT_3D('',#106543,#68752,#68753) ;
#54638=AXIS2_PLACEMENT_3D('',#106544,#68754,#68755) ;
#54639=AXIS2_PLACEMENT_3D('',#106563,#68758,#68759) ;
#54640=AXIS2_PLACEMENT_3D('',#106565,#68760,#68761) ;
#54641=AXIS2_PLACEMENT_3D('',#106581,#68762,#68763) ;
#54642=AXIS2_PLACEMENT_3D('',#106582,#68764,#68765) ;
#54643=AXIS2_PLACEMENT_3D('',#106603,#68768,#68769) ;
#54644=AXIS2_PLACEMENT_3D('',#106605,#68770,#68771) ;
#54645=AXIS2_PLACEMENT_3D('',#106607,#68772,#68773) ;
#54646=AXIS2_PLACEMENT_3D('',#106624,#68774,#68775) ;
#54647=AXIS2_PLACEMENT_3D('',#106643,#68778,#68779) ;
#54648=AXIS2_PLACEMENT_3D('',#106645,#68780,#68781) ;
#54649=AXIS2_PLACEMENT_3D('',#106647,#68782,#68783) ;
#54650=AXIS2_PLACEMENT_3D('',#106662,#68784,#68785) ;
#54651=AXIS2_PLACEMENT_3D('',#106683,#68788,#68789) ;
#54652=AXIS2_PLACEMENT_3D('',#106685,#68790,#68791) ;
#54653=AXIS2_PLACEMENT_3D('',#106687,#68792,#68793) ;
#54654=AXIS2_PLACEMENT_3D('',#106704,#68794,#68795) ;
#54655=AXIS2_PLACEMENT_3D('',#106723,#68798,#68799) ;
#54656=AXIS2_PLACEMENT_3D('',#106725,#68800,#68801) ;
#54657=AXIS2_PLACEMENT_3D('',#106727,#68802,#68803) ;
#54658=AXIS2_PLACEMENT_3D('',#106742,#68804,#68805) ;
#54659=AXIS2_PLACEMENT_3D('',#106763,#68808,#68809) ;
#54660=AXIS2_PLACEMENT_3D('',#106765,#68810,#68811) ;
#54661=AXIS2_PLACEMENT_3D('',#106767,#68812,#68813) ;
#54662=AXIS2_PLACEMENT_3D('',#106784,#68814,#68815) ;
#54663=AXIS2_PLACEMENT_3D('',#106803,#68818,#68819) ;
#54664=AXIS2_PLACEMENT_3D('',#106805,#68820,#68821) ;
#54665=AXIS2_PLACEMENT_3D('',#106807,#68822,#68823) ;
#54666=AXIS2_PLACEMENT_3D('',#106822,#68824,#68825) ;
#54667=AXIS2_PLACEMENT_3D('',#106843,#68828,#68829) ;
#54668=AXIS2_PLACEMENT_3D('',#106845,#68830,#68831) ;
#54669=AXIS2_PLACEMENT_3D('',#106847,#68832,#68833) ;
#54670=AXIS2_PLACEMENT_3D('',#106864,#68834,#68835) ;
#54671=AXIS2_PLACEMENT_3D('',#106883,#68838,#68839) ;
#54672=AXIS2_PLACEMENT_3D('',#106885,#68840,#68841) ;
#54673=AXIS2_PLACEMENT_3D('',#106887,#68842,#68843) ;
#54674=AXIS2_PLACEMENT_3D('',#106902,#68844,#68845) ;
#54675=AXIS2_PLACEMENT_3D('',#106923,#68848,#68849) ;
#54676=AXIS2_PLACEMENT_3D('',#106925,#68850,#68851) ;
#54677=AXIS2_PLACEMENT_3D('',#106927,#68852,#68853) ;
#54678=AXIS2_PLACEMENT_3D('',#106944,#68854,#68855) ;
#54679=AXIS2_PLACEMENT_3D('',#106963,#68858,#68859) ;
#54680=AXIS2_PLACEMENT_3D('',#106965,#68860,#68861) ;
#54681=AXIS2_PLACEMENT_3D('',#106967,#68862,#68863) ;
#54682=AXIS2_PLACEMENT_3D('',#106982,#68864,#68865) ;
#54683=AXIS2_PLACEMENT_3D('',#107003,#68868,#68869) ;
#54684=AXIS2_PLACEMENT_3D('',#107005,#68870,#68871) ;
#54685=AXIS2_PLACEMENT_3D('',#107007,#68872,#68873) ;
#54686=AXIS2_PLACEMENT_3D('',#107024,#68874,#68875) ;
#54687=AXIS2_PLACEMENT_3D('',#107043,#68878,#68879) ;
#54688=AXIS2_PLACEMENT_3D('',#107045,#68880,#68881) ;
#54689=AXIS2_PLACEMENT_3D('',#107047,#68882,#68883) ;
#54690=AXIS2_PLACEMENT_3D('',#107062,#68884,#68885) ;
#54691=AXIS2_PLACEMENT_3D('',#107083,#68888,#68889) ;
#54692=AXIS2_PLACEMENT_3D('',#107085,#68890,#68891) ;
#54693=AXIS2_PLACEMENT_3D('',#107087,#68892,#68893) ;
#54694=AXIS2_PLACEMENT_3D('',#107104,#68894,#68895) ;
#54695=AXIS2_PLACEMENT_3D('',#107123,#68898,#68899) ;
#54696=AXIS2_PLACEMENT_3D('',#107125,#68900,#68901) ;
#54697=AXIS2_PLACEMENT_3D('',#107127,#68902,#68903) ;
#54698=AXIS2_PLACEMENT_3D('',#107142,#68904,#68905) ;
#54699=AXIS2_PLACEMENT_3D('',#107163,#68908,#68909) ;
#54700=AXIS2_PLACEMENT_3D('',#107165,#68910,#68911) ;
#54701=AXIS2_PLACEMENT_3D('',#107167,#68912,#68913) ;
#54702=AXIS2_PLACEMENT_3D('',#107184,#68914,#68915) ;
#54703=AXIS2_PLACEMENT_3D('',#107203,#68918,#68919) ;
#54704=AXIS2_PLACEMENT_3D('',#107205,#68920,#68921) ;
#54705=AXIS2_PLACEMENT_3D('',#107207,#68922,#68923) ;
#54706=AXIS2_PLACEMENT_3D('',#107222,#68924,#68925) ;
#54707=AXIS2_PLACEMENT_3D('',#107243,#68928,#68929) ;
#54708=AXIS2_PLACEMENT_3D('',#107245,#68930,#68931) ;
#54709=AXIS2_PLACEMENT_3D('',#107247,#68932,#68933) ;
#54710=AXIS2_PLACEMENT_3D('',#107264,#68934,#68935) ;
#54711=AXIS2_PLACEMENT_3D('',#107283,#68938,#68939) ;
#54712=AXIS2_PLACEMENT_3D('',#107285,#68940,#68941) ;
#54713=AXIS2_PLACEMENT_3D('',#107287,#68942,#68943) ;
#54714=AXIS2_PLACEMENT_3D('',#107302,#68944,#68945) ;
#54715=AXIS2_PLACEMENT_3D('',#107323,#68948,#68949) ;
#54716=AXIS2_PLACEMENT_3D('',#107325,#68950,#68951) ;
#54717=AXIS2_PLACEMENT_3D('',#107327,#68952,#68953) ;
#54718=AXIS2_PLACEMENT_3D('',#107344,#68954,#68955) ;
#54719=AXIS2_PLACEMENT_3D('',#107347,#68958,#68959) ;
#54720=AXIS2_PLACEMENT_3D('',#107353,#68963,#68964) ;
#54721=AXIS2_PLACEMENT_3D('',#107356,#68966,#68967) ;
#54722=AXIS2_PLACEMENT_3D('',#107357,#68968,#68969) ;
#54723=AXIS2_PLACEMENT_3D('',#107361,#68972,#68973) ;
#54724=AXIS2_PLACEMENT_3D('',#107364,#68975,#68976) ;
#54725=AXIS2_PLACEMENT_3D('',#107365,#68977,#68978) ;
#54726=AXIS2_PLACEMENT_3D('',#107369,#68981,#68982) ;
#54727=AXIS2_PLACEMENT_3D('',#107372,#68984,#68985) ;
#54728=AXIS2_PLACEMENT_3D('',#107373,#68986,#68987) ;
#54729=AXIS2_PLACEMENT_3D('',#107377,#68990,#68991) ;
#54730=AXIS2_PLACEMENT_3D('',#107380,#68993,#68994) ;
#54731=AXIS2_PLACEMENT_3D('',#107381,#68995,#68996) ;
#54732=AXIS2_PLACEMENT_3D('',#107385,#68999,#69000) ;
#54733=AXIS2_PLACEMENT_3D('',#107388,#69002,#69003) ;
#54734=AXIS2_PLACEMENT_3D('',#107389,#69004,#69005) ;
#54735=AXIS2_PLACEMENT_3D('',#107393,#69008,#69009) ;
#54736=AXIS2_PLACEMENT_3D('',#107396,#69011,#69012) ;
#54737=AXIS2_PLACEMENT_3D('',#107397,#69013,#69014) ;
#54738=AXIS2_PLACEMENT_3D('',#107401,#69017,#69018) ;
#54739=AXIS2_PLACEMENT_3D('',#107404,#69020,#69021) ;
#54740=AXIS2_PLACEMENT_3D('',#107405,#69022,#69023) ;
#54741=AXIS2_PLACEMENT_3D('',#107409,#69026,#69027) ;
#54742=AXIS2_PLACEMENT_3D('',#107412,#69029,#69030) ;
#54743=AXIS2_PLACEMENT_3D('',#107413,#69031,#69032) ;
#54744=AXIS2_PLACEMENT_3D('',#107417,#69035,#69036) ;
#54745=AXIS2_PLACEMENT_3D('',#107420,#69038,#69039) ;
#54746=AXIS2_PLACEMENT_3D('',#107421,#69040,#69041) ;
#54747=AXIS2_PLACEMENT_3D('',#107425,#69044,#69045) ;
#54748=AXIS2_PLACEMENT_3D('',#107428,#69047,#69048) ;
#54749=AXIS2_PLACEMENT_3D('',#107429,#69049,#69050) ;
#54750=AXIS2_PLACEMENT_3D('',#107433,#69053,#69054) ;
#54751=AXIS2_PLACEMENT_3D('',#107436,#69056,#69057) ;
#54752=AXIS2_PLACEMENT_3D('',#107437,#69058,#69059) ;
#54753=AXIS2_PLACEMENT_3D('',#107441,#69062,#69063) ;
#54754=AXIS2_PLACEMENT_3D('',#107444,#69065,#69066) ;
#54755=AXIS2_PLACEMENT_3D('',#107445,#69067,#69068) ;
#54756=AXIS2_PLACEMENT_3D('',#107449,#69071,#69072) ;
#54757=AXIS2_PLACEMENT_3D('',#107452,#69074,#69075) ;
#54758=AXIS2_PLACEMENT_3D('',#107453,#69076,#69077) ;
#54759=AXIS2_PLACEMENT_3D('',#107457,#69080,#69081) ;
#54760=AXIS2_PLACEMENT_3D('',#107460,#69083,#69084) ;
#54761=AXIS2_PLACEMENT_3D('',#107461,#69085,#69086) ;
#54762=AXIS2_PLACEMENT_3D('',#107465,#69089,#69090) ;
#54763=AXIS2_PLACEMENT_3D('',#107468,#69092,#69093) ;
#54764=AXIS2_PLACEMENT_3D('',#107469,#69094,#69095) ;
#54765=AXIS2_PLACEMENT_3D('',#107473,#69098,#69099) ;
#54766=AXIS2_PLACEMENT_3D('',#107476,#69101,#69102) ;
#54767=AXIS2_PLACEMENT_3D('',#107477,#69103,#69104) ;
#54768=AXIS2_PLACEMENT_3D('',#107481,#69107,#69108) ;
#54769=AXIS2_PLACEMENT_3D('',#107484,#69110,#69111) ;
#54770=AXIS2_PLACEMENT_3D('',#107485,#69112,#69113) ;
#54771=AXIS2_PLACEMENT_3D('',#107489,#69116,#69117) ;
#54772=AXIS2_PLACEMENT_3D('',#107492,#69119,#69120) ;
#54773=AXIS2_PLACEMENT_3D('',#107493,#69121,#69122) ;
#54774=AXIS2_PLACEMENT_3D('',#107497,#69125,#69126) ;
#54775=AXIS2_PLACEMENT_3D('',#107500,#69128,#69129) ;
#54776=AXIS2_PLACEMENT_3D('',#107501,#69130,#69131) ;
#54777=AXIS2_PLACEMENT_3D('',#107505,#69134,#69135) ;
#54778=AXIS2_PLACEMENT_3D('',#107508,#69137,#69138) ;
#54779=AXIS2_PLACEMENT_3D('',#107509,#69139,#69140) ;
#54780=AXIS2_PLACEMENT_3D('',#107510,#69141,#69142) ;
#54781=AXIS2_PLACEMENT_3D('',#107511,#69143,#69144) ;
#54782=AXIS2_PLACEMENT_3D('',#107512,#69145,#69146) ;
#54783=AXIS2_PLACEMENT_3D('',#107513,#69147,#69148) ;
#54784=AXIS2_PLACEMENT_3D('',#107514,#69149,#69150) ;
#54785=AXIS2_PLACEMENT_3D('',#107515,#69151,#69152) ;
#54786=AXIS2_PLACEMENT_3D('',#107516,#69153,#69154) ;
#54787=AXIS2_PLACEMENT_3D('',#107517,#69155,#69156) ;
#54788=AXIS2_PLACEMENT_3D('',#107518,#69157,#69158) ;
#54789=AXIS2_PLACEMENT_3D('',#107519,#69159,#69160) ;
#54790=AXIS2_PLACEMENT_3D('',#107520,#69161,#69162) ;
#54791=AXIS2_PLACEMENT_3D('',#107521,#69163,#69164) ;
#54792=AXIS2_PLACEMENT_3D('',#107522,#69165,#69166) ;
#54793=AXIS2_PLACEMENT_3D('',#107523,#69167,#69168) ;
#54794=AXIS2_PLACEMENT_3D('',#107524,#69169,#69170) ;
#54795=AXIS2_PLACEMENT_3D('',#107525,#69171,#69172) ;
#54796=AXIS2_PLACEMENT_3D('',#107526,#69173,#69174) ;
#54797=AXIS2_PLACEMENT_3D('',#107527,#69175,#69176) ;
#54798=AXIS2_PLACEMENT_3D('',#107528,#69177,#69178) ;
#54799=AXIS2_PLACEMENT_3D('',#107529,#69179,#69180) ;
#54800=AXIS2_PLACEMENT_3D('',#107530,#69181,#69182) ;
#54801=AXIS2_PLACEMENT_3D('',#107531,#69183,#69184) ;
#54802=AXIS2_PLACEMENT_3D('',#107532,#69185,#69186) ;
#54803=AXIS2_PLACEMENT_3D('',#107533,#69187,#69188) ;
#54804=AXIS2_PLACEMENT_3D('',#107534,#69189,#69190) ;
#54805=AXIS2_PLACEMENT_3D('',#107535,#69191,#69192) ;
#54806=AXIS2_PLACEMENT_3D('',#107536,#69193,#69194) ;
#54807=AXIS2_PLACEMENT_3D('',#107537,#69195,#69196) ;
#54808=AXIS2_PLACEMENT_3D('',#107538,#69197,#69198) ;
#54809=AXIS2_PLACEMENT_3D('',#107539,#69199,#69200) ;
#54810=AXIS2_PLACEMENT_3D('',#107540,#69201,#69202) ;
#54811=AXIS2_PLACEMENT_3D('',#107541,#69203,#69204) ;
#54812=AXIS2_PLACEMENT_3D('',#107542,#69205,#69206) ;
#54813=AXIS2_PLACEMENT_3D('',#107543,#69207,#69208) ;
#54814=AXIS2_PLACEMENT_3D('',#107544,#69209,#69210) ;
#54815=AXIS2_PLACEMENT_3D('',#107545,#69211,#69212) ;
#54816=AXIS2_PLACEMENT_3D('',#107547,#69213,#69214) ;
#54817=AXIS2_PLACEMENT_3D('',#107548,#69215,#69216) ;
#54818=AXIS2_PLACEMENT_3D('',#107549,#69217,#69218) ;
#54819=AXIS2_PLACEMENT_3D('',#107550,#69219,#69220) ;
#54820=AXIS2_PLACEMENT_3D('',#107551,#69221,#69222) ;
#54821=AXIS2_PLACEMENT_3D('',#107552,#69223,#69224) ;
#54822=AXIS2_PLACEMENT_3D('',#107553,#69225,#69226) ;
#54823=AXIS2_PLACEMENT_3D('',#107555,#69227,#69228) ;
#54824=AXIS2_PLACEMENT_3D('',#107557,#69229,#69230) ;
#54825=AXIS2_PLACEMENT_3D('',#107559,#69231,#69232) ;
#54826=AXIS2_PLACEMENT_3D('',#107561,#69233,#69234) ;
#54827=AXIS2_PLACEMENT_3D('',#107563,#69235,#69236) ;
#54828=AXIS2_PLACEMENT_3D('',#107565,#69237,#69238) ;
#54829=AXIS2_PLACEMENT_3D('',#107567,#69239,#69240) ;
#54830=AXIS2_PLACEMENT_3D('',#107569,#69241,#69242) ;
#54831=AXIS2_PLACEMENT_3D('',#107571,#69243,#69244) ;
#54832=AXIS2_PLACEMENT_3D('',#107573,#69245,#69246) ;
#54833=AXIS2_PLACEMENT_3D('',#107575,#69247,#69248) ;
#54834=AXIS2_PLACEMENT_3D('',#107577,#69249,#69250) ;
#54835=AXIS2_PLACEMENT_3D('',#107579,#69251,#69252) ;
#54836=AXIS2_PLACEMENT_3D('',#107581,#69253,#69254) ;
#54837=AXIS2_PLACEMENT_3D('',#107583,#69255,#69256) ;
#54838=AXIS2_PLACEMENT_3D('',#107585,#69257,#69258) ;
#54839=AXIS2_PLACEMENT_3D('',#107587,#69259,#69260) ;
#54840=AXIS2_PLACEMENT_3D('',#107589,#69261,#69262) ;
#54841=AXIS2_PLACEMENT_3D('',#107591,#69263,#69264) ;
#54842=AXIS2_PLACEMENT_3D('',#107593,#69265,#69266) ;
#54843=AXIS2_PLACEMENT_3D('',#107595,#69267,#69268) ;
#54844=AXIS2_PLACEMENT_3D('',#107597,#69269,#69270) ;
#54845=AXIS2_PLACEMENT_3D('',#107599,#69271,#69272) ;
#54846=AXIS2_PLACEMENT_3D('',#107601,#69273,#69274) ;
#54847=AXIS2_PLACEMENT_3D('',#107603,#69275,#69276) ;
#54848=AXIS2_PLACEMENT_3D('',#107605,#69277,#69278) ;
#54849=AXIS2_PLACEMENT_3D('',#107607,#69279,#69280) ;
#54850=AXIS2_PLACEMENT_3D('',#107609,#69281,#69282) ;
#54851=AXIS2_PLACEMENT_3D('',#107611,#69283,#69284) ;
#54852=AXIS2_PLACEMENT_3D('',#107613,#69285,#69286) ;
#54853=AXIS2_PLACEMENT_3D('',#107615,#69287,#69288) ;
#54854=AXIS2_PLACEMENT_3D('',#107617,#69289,#69290) ;
#54855=AXIS2_PLACEMENT_3D('',#107619,#69291,#69292) ;
#54856=AXIS2_PLACEMENT_3D('',#107621,#69293,#69294) ;
#54857=AXIS2_PLACEMENT_3D('',#107623,#69295,#69296) ;
#54858=AXIS2_PLACEMENT_3D('',#107625,#69297,#69298) ;
#54859=AXIS2_PLACEMENT_3D('',#107627,#69299,#69300) ;
#54860=AXIS2_PLACEMENT_3D('',#107629,#69301,#69302) ;
#54861=AXIS2_PLACEMENT_3D('',#107631,#69303,#69304) ;
#54862=AXIS2_PLACEMENT_3D('',#107633,#69305,#69306) ;
#54863=AXIS2_PLACEMENT_3D('',#107635,#69307,#69308) ;
#54864=AXIS2_PLACEMENT_3D('',#107636,#69309,#69310) ;
#54865=AXIS2_PLACEMENT_3D('',#107637,#69311,#69312) ;
#54866=AXIS2_PLACEMENT_3D('',#107641,#69314,#69315) ;
#54867=AXIS2_PLACEMENT_3D('',#107643,#69317,#69318) ;
#54868=AXIS2_PLACEMENT_3D('',#107647,#69320,#69321) ;
#54869=AXIS2_PLACEMENT_3D('',#107649,#69323,#69324) ;
#54870=AXIS2_PLACEMENT_3D('',#107653,#69326,#69327) ;
#54871=AXIS2_PLACEMENT_3D('',#107655,#69329,#69330) ;
#54872=AXIS2_PLACEMENT_3D('',#107659,#69332,#69333) ;
#54873=AXIS2_PLACEMENT_3D('',#107661,#69335,#69336) ;
#54874=AXIS2_PLACEMENT_3D('',#107665,#69338,#69339) ;
#54875=AXIS2_PLACEMENT_3D('',#107667,#69341,#69342) ;
#54876=AXIS2_PLACEMENT_3D('',#107671,#69344,#69345) ;
#54877=AXIS2_PLACEMENT_3D('',#107673,#69347,#69348) ;
#54878=AXIS2_PLACEMENT_3D('',#107677,#69350,#69351) ;
#54879=AXIS2_PLACEMENT_3D('',#107679,#69353,#69354) ;
#54880=AXIS2_PLACEMENT_3D('',#107683,#69356,#69357) ;
#54881=AXIS2_PLACEMENT_3D('',#107685,#69359,#69360) ;
#54882=AXIS2_PLACEMENT_3D('',#107689,#69362,#69363) ;
#54883=AXIS2_PLACEMENT_3D('',#107691,#69365,#69366) ;
#54884=AXIS2_PLACEMENT_3D('',#107695,#69368,#69369) ;
#54885=AXIS2_PLACEMENT_3D('',#107697,#69371,#69372) ;
#54886=AXIS2_PLACEMENT_3D('',#107701,#69374,#69375) ;
#54887=AXIS2_PLACEMENT_3D('',#107703,#69377,#69378) ;
#54888=AXIS2_PLACEMENT_3D('',#107707,#69380,#69381) ;
#54889=AXIS2_PLACEMENT_3D('',#107709,#69383,#69384) ;
#54890=AXIS2_PLACEMENT_3D('',#107713,#69386,#69387) ;
#54891=AXIS2_PLACEMENT_3D('',#107715,#69389,#69390) ;
#54892=AXIS2_PLACEMENT_3D('',#107719,#69392,#69393) ;
#54893=AXIS2_PLACEMENT_3D('',#107721,#69395,#69396) ;
#54894=AXIS2_PLACEMENT_3D('',#107725,#69398,#69399) ;
#54895=AXIS2_PLACEMENT_3D('',#107727,#69401,#69402) ;
#54896=AXIS2_PLACEMENT_3D('',#107731,#69404,#69405) ;
#54897=AXIS2_PLACEMENT_3D('',#107733,#69407,#69408) ;
#54898=AXIS2_PLACEMENT_3D('',#107737,#69410,#69411) ;
#54899=AXIS2_PLACEMENT_3D('',#107739,#69413,#69414) ;
#54900=AXIS2_PLACEMENT_3D('',#107743,#69416,#69417) ;
#54901=AXIS2_PLACEMENT_3D('',#107745,#69419,#69420) ;
#54902=AXIS2_PLACEMENT_3D('',#107749,#69422,#69423) ;
#54903=AXIS2_PLACEMENT_3D('',#107751,#69425,#69426) ;
#54904=AXIS2_PLACEMENT_3D('',#107755,#69428,#69429) ;
#54905=AXIS2_PLACEMENT_3D('',#107757,#69431,#69432) ;
#54906=AXIS2_PLACEMENT_3D('',#107774,#69433,#69434) ;
#54907=AXIS2_PLACEMENT_3D('',#107789,#69435,#69436) ;
#54908=AXIS2_PLACEMENT_3D('',#107808,#69438,#69439) ;
#54909=AXIS2_PLACEMENT_3D('',#107827,#69441,#69442) ;
#54910=AXIS2_PLACEMENT_3D('',#107860,#69444,#69445) ;
#54911=AXIS2_PLACEMENT_3D('',#107875,#69446,#69447) ;
#54912=AXIS2_PLACEMENT_3D('',#107892,#69448,#69449) ;
#54913=AXIS2_PLACEMENT_3D('',#107926,#69451,#69452) ;
#54914=AXIS2_PLACEMENT_3D('',#107957,#69453,#69454) ;
#54915=AXIS2_PLACEMENT_3D('',#107972,#69455,#69456) ;
#54916=AXIS2_PLACEMENT_3D('',#107989,#69457,#69458) ;
#54917=AXIS2_PLACEMENT_3D('',#108023,#69460,#69461) ;
#54918=AXIS2_PLACEMENT_3D('',#108054,#69462,#69463) ;
#54919=AXIS2_PLACEMENT_3D('',#108069,#69464,#69465) ;
#54920=AXIS2_PLACEMENT_3D('',#108086,#69466,#69467) ;
#54921=AXIS2_PLACEMENT_3D('',#108120,#69469,#69470) ;
#54922=AXIS2_PLACEMENT_3D('',#108151,#69471,#69472) ;
#54923=AXIS2_PLACEMENT_3D('',#108166,#69473,#69474) ;
#54924=AXIS2_PLACEMENT_3D('',#108183,#69475,#69476) ;
#54925=AXIS2_PLACEMENT_3D('',#108217,#69478,#69479) ;
#54926=AXIS2_PLACEMENT_3D('',#108248,#69480,#69481) ;
#54927=AXIS2_PLACEMENT_3D('',#108263,#69482,#69483) ;
#54928=AXIS2_PLACEMENT_3D('',#108280,#69484,#69485) ;
#54929=AXIS2_PLACEMENT_3D('',#108314,#69487,#69488) ;
#54930=AXIS2_PLACEMENT_3D('',#108345,#69489,#69490) ;
#54931=AXIS2_PLACEMENT_3D('',#108360,#69491,#69492) ;
#54932=AXIS2_PLACEMENT_3D('',#108377,#69493,#69494) ;
#54933=AXIS2_PLACEMENT_3D('',#108411,#69496,#69497) ;
#54934=AXIS2_PLACEMENT_3D('',#108442,#69498,#69499) ;
#54935=AXIS2_PLACEMENT_3D('',#108457,#69500,#69501) ;
#54936=AXIS2_PLACEMENT_3D('',#108474,#69502,#69503) ;
#54937=AXIS2_PLACEMENT_3D('',#108508,#69505,#69506) ;
#54938=AXIS2_PLACEMENT_3D('',#108539,#69507,#69508) ;
#54939=AXIS2_PLACEMENT_3D('',#108554,#69509,#69510) ;
#54940=AXIS2_PLACEMENT_3D('',#108571,#69511,#69512) ;
#54941=AXIS2_PLACEMENT_3D('',#108605,#69514,#69515) ;
#54942=AXIS2_PLACEMENT_3D('',#108636,#69516,#69517) ;
#54943=AXIS2_PLACEMENT_3D('',#108651,#69518,#69519) ;
#54944=AXIS2_PLACEMENT_3D('',#108668,#69520,#69521) ;
#54945=AXIS2_PLACEMENT_3D('',#108699,#69522,#69523) ;
#54946=AXIS2_PLACEMENT_3D('',#108730,#69524,#69525) ;
#54947=AXIS2_PLACEMENT_3D('',#108745,#69526,#69527) ;
#54948=AXIS2_PLACEMENT_3D('',#108762,#69528,#69529) ;
#54949=AXIS2_PLACEMENT_3D('',#108763,#69530,#69531) ;
#54950=AXIS2_PLACEMENT_3D('',#108764,#69532,#69533) ;
#54951=AXIS2_PLACEMENT_3D('',#108766,#69534,#69535) ;
#54952=AXIS2_PLACEMENT_3D('',#108781,#69536,#69537) ;
#54953=AXIS2_PLACEMENT_3D('',#108800,#69539,#69540) ;
#54954=AXIS2_PLACEMENT_3D('',#108801,#69541,#69542) ;
#54955=AXIS2_PLACEMENT_3D('',#108802,#69543,#69544) ;
#54956=AXIS2_PLACEMENT_3D('',#108803,#69545,#69546) ;
#54957=AXIS2_PLACEMENT_3D('',#108805,#69547,#69548) ;
#54958=AXIS2_PLACEMENT_3D('',#108820,#69549,#69550) ;
#54959=AXIS2_PLACEMENT_3D('',#108839,#69552,#69553) ;
#54960=AXIS2_PLACEMENT_3D('',#108840,#69554,#69555) ;
#54961=AXIS2_PLACEMENT_3D('',#108841,#69556,#69557) ;
#54962=AXIS2_PLACEMENT_3D('',#108842,#69558,#69559) ;
#54963=AXIS2_PLACEMENT_3D('',#108844,#69560,#69561) ;
#54964=AXIS2_PLACEMENT_3D('',#108859,#69562,#69563) ;
#54965=AXIS2_PLACEMENT_3D('',#108878,#69565,#69566) ;
#54966=AXIS2_PLACEMENT_3D('',#108879,#69567,#69568) ;
#54967=AXIS2_PLACEMENT_3D('',#108880,#69569,#69570) ;
#54968=AXIS2_PLACEMENT_3D('',#108881,#69571,#69572) ;
#54969=AXIS2_PLACEMENT_3D('',#108883,#69573,#69574) ;
#54970=AXIS2_PLACEMENT_3D('',#108898,#69575,#69576) ;
#54971=AXIS2_PLACEMENT_3D('',#108917,#69578,#69579) ;
#54972=AXIS2_PLACEMENT_3D('',#108918,#69580,#69581) ;
#54973=AXIS2_PLACEMENT_3D('',#108919,#69582,#69583) ;
#54974=AXIS2_PLACEMENT_3D('',#108920,#69584,#69585) ;
#54975=AXIS2_PLACEMENT_3D('',#108922,#69586,#69587) ;
#54976=AXIS2_PLACEMENT_3D('',#108937,#69588,#69589) ;
#54977=AXIS2_PLACEMENT_3D('',#108956,#69591,#69592) ;
#54978=AXIS2_PLACEMENT_3D('',#108957,#69593,#69594) ;
#54979=AXIS2_PLACEMENT_3D('',#108958,#69595,#69596) ;
#54980=AXIS2_PLACEMENT_3D('',#108959,#69597,#69598) ;
#54981=AXIS2_PLACEMENT_3D('',#108961,#69599,#69600) ;
#54982=AXIS2_PLACEMENT_3D('',#108976,#69601,#69602) ;
#54983=AXIS2_PLACEMENT_3D('',#108995,#69604,#69605) ;
#54984=AXIS2_PLACEMENT_3D('',#108996,#69606,#69607) ;
#54985=AXIS2_PLACEMENT_3D('',#108997,#69608,#69609) ;
#54986=AXIS2_PLACEMENT_3D('',#108998,#69610,#69611) ;
#54987=AXIS2_PLACEMENT_3D('',#109000,#69612,#69613) ;
#54988=AXIS2_PLACEMENT_3D('',#109015,#69614,#69615) ;
#54989=AXIS2_PLACEMENT_3D('',#109034,#69617,#69618) ;
#54990=AXIS2_PLACEMENT_3D('',#109035,#69619,#69620) ;
#54991=AXIS2_PLACEMENT_3D('',#109036,#69621,#69622) ;
#54992=AXIS2_PLACEMENT_3D('',#109037,#69623,#69624) ;
#54993=AXIS2_PLACEMENT_3D('',#109039,#69625,#69626) ;
#54994=AXIS2_PLACEMENT_3D('',#109054,#69627,#69628) ;
#54995=AXIS2_PLACEMENT_3D('',#109073,#69630,#69631) ;
#54996=AXIS2_PLACEMENT_3D('',#109074,#69632,#69633) ;
#54997=AXIS2_PLACEMENT_3D('',#109075,#69634,#69635) ;
#54998=AXIS2_PLACEMENT_3D('',#109076,#69636,#69637) ;
#54999=AXIS2_PLACEMENT_3D('',#109078,#69638,#69639) ;
#55000=AXIS2_PLACEMENT_3D('',#109093,#69640,#69641) ;
#55001=AXIS2_PLACEMENT_3D('',#109112,#69643,#69644) ;
#55002=AXIS2_PLACEMENT_3D('',#109113,#69645,#69646) ;
#55003=AXIS2_PLACEMENT_3D('',#109114,#69647,#69648) ;
#55004=AXIS2_PLACEMENT_3D('',#109115,#69649,#69650) ;
#55005=AXIS2_PLACEMENT_3D('',#109116,#69651,#69652) ;
#55006=AXIS2_PLACEMENT_3D('',#109119,#69655,#69656) ;
#55007=AXIS2_PLACEMENT_3D('',#109121,#69658,#69659) ;
#55008=AXIS2_PLACEMENT_3D('',#109123,#69661,#69662) ;
#55009=AXIS2_PLACEMENT_3D('',#109124,#69663,#69664) ;
#55010=AXIS2_PLACEMENT_3D('',#109127,#69667,#69668) ;
#55011=AXIS2_PLACEMENT_3D('',#109130,#69671,#69672) ;
#55012=AXIS2_PLACEMENT_3D('',#109131,#69673,#69674) ;
#55013=AXIS2_PLACEMENT_3D('',#109134,#69677,#69678) ;
#55014=AXIS2_PLACEMENT_3D('',#109137,#69681,#69682) ;
#55015=AXIS2_PLACEMENT_3D('',#109138,#69683,#69684) ;
#55016=AXIS2_PLACEMENT_3D('',#109141,#69687,#69688) ;
#55017=AXIS2_PLACEMENT_3D('',#109144,#69691,#69692) ;
#55018=AXIS2_PLACEMENT_3D('',#109145,#69693,#69694) ;
#55019=AXIS2_PLACEMENT_3D('',#109148,#69697,#69698) ;
#55020=AXIS2_PLACEMENT_3D('',#109151,#69701,#69702) ;
#55021=AXIS2_PLACEMENT_3D('',#109152,#69703,#69704) ;
#55022=AXIS2_PLACEMENT_3D('',#109155,#69707,#69708) ;
#55023=AXIS2_PLACEMENT_3D('',#109158,#69711,#69712) ;
#55024=AXIS2_PLACEMENT_3D('',#109159,#69713,#69714) ;
#55025=AXIS2_PLACEMENT_3D('',#109162,#69717,#69718) ;
#55026=AXIS2_PLACEMENT_3D('',#109165,#69721,#69722) ;
#55027=AXIS2_PLACEMENT_3D('',#109166,#69723,#69724) ;
#55028=AXIS2_PLACEMENT_3D('',#109169,#69727,#69728) ;
#55029=AXIS2_PLACEMENT_3D('',#109172,#69731,#69732) ;
#55030=AXIS2_PLACEMENT_3D('',#109173,#69733,#69734) ;
#55031=AXIS2_PLACEMENT_3D('',#109176,#69737,#69738) ;
#55032=AXIS2_PLACEMENT_3D('',#109179,#69741,#69742) ;
#55033=AXIS2_PLACEMENT_3D('',#109180,#69743,#69744) ;
#55034=AXIS2_PLACEMENT_3D('',#109183,#69747,#69748) ;
#55035=AXIS2_PLACEMENT_3D('',#109185,#69750,#69751) ;
#55036=AXIS2_PLACEMENT_3D('',#109186,#69752,#69753) ;
#55037=AXIS2_PLACEMENT_3D('',#109187,#69754,#69755) ;
#55038=AXIS2_PLACEMENT_3D('',#109188,#69756,#69757) ;
#55039=AXIS2_PLACEMENT_3D('',#109189,#69758,#69759) ;
#55040=AXIS2_PLACEMENT_3D('',#109190,#69760,#69761) ;
#55041=AXIS2_PLACEMENT_3D('',#109191,#69762,#69763) ;
#55042=AXIS2_PLACEMENT_3D('',#109192,#69764,#69765) ;
#55043=AXIS2_PLACEMENT_3D('',#109193,#69766,#69767) ;
#55044=AXIS2_PLACEMENT_3D('',#109194,#69768,#69769) ;
#55045=AXIS2_PLACEMENT_3D('',#109195,#69770,#69771) ;
#68528=DIRECTION('axis',(0.,0.,1.)) ;
#68529=DIRECTION('refdir',(1.,0.,0.)) ;
#68530=DIRECTION('center_axis',(1.,2.22044604925031E-16,0.)) ;
#68531=DIRECTION('ref_axis',(0.,1.,0.)) ;
#68532=DIRECTION('center_axis',(1.,2.22044604925031E-16,0.)) ;
#68533=DIRECTION('ref_axis',(2.22044604925031E-16,-1.,0.)) ;
#68534=DIRECTION('center_axis',(0.,0.,1.)) ;
#68535=DIRECTION('ref_axis',(0.,-1.,0.)) ;
#68536=DIRECTION('center_axis',(1.,2.22044604925031E-16,0.)) ;
#68537=DIRECTION('ref_axis',(-2.22044604925031E-16,1.,0.)) ;
#68538=DIRECTION('center_axis',(-1.,-2.22044604925031E-16,0.)) ;
#68539=DIRECTION('ref_axis',(2.22044604925031E-16,-1.,0.)) ;
#68540=DIRECTION('center_axis',(1.,2.22044604925031E-16,0.)) ;
#68541=DIRECTION('ref_axis',(0.,0.,-1.)) ;
#68542=DIRECTION('center_axis',(-1.,-2.22044604925031E-16,0.)) ;
#68543=DIRECTION('ref_axis',(2.22044604925031E-16,-1.,0.)) ;
#68544=DIRECTION('center_axis',(-2.22044604925031E-16,1.,0.)) ;
#68545=DIRECTION('ref_axis',(0.,0.,1.)) ;
#68546=DIRECTION('center_axis',(-1.,-2.22044604925031E-16,0.)) ;
#68547=DIRECTION('ref_axis',(2.22044604925031E-16,-1.,0.)) ;
#68548=DIRECTION('center_axis',(-1.,-2.22044604925031E-16,0.)) ;
#68549=DIRECTION('ref_axis',(2.22044604925031E-16,-1.,0.)) ;
#68550=DIRECTION('center_axis',(-1.,-2.22044604925031E-16,0.)) ;
#68551=DIRECTION('ref_axis',(2.22044604925031E-16,-1.,0.)) ;
#68552=DIRECTION('center_axis',(1.,2.22044604925031E-16,0.)) ;
#68553=DIRECTION('ref_axis',(2.22044604925031E-16,-1.,0.)) ;
#68554=DIRECTION('center_axis',(-1.,-2.22044604925031E-16,0.)) ;
#68555=DIRECTION('ref_axis',(2.22044604925031E-16,-1.,0.)) ;
#68556=DIRECTION('center_axis',(-1.,-2.22044604925031E-16,0.)) ;
#68557=DIRECTION('ref_axis',(2.22044604925031E-16,-1.,0.)) ;
#68558=DIRECTION('center_axis',(1.,2.22044604925031E-16,0.)) ;
#68559=DIRECTION('ref_axis',(0.,0.,-1.)) ;
#68560=DIRECTION('center_axis',(1.,2.22044604925031E-16,0.)) ;
#68561=DIRECTION('ref_axis',(9.02179155423715E-17,-0.406305370818768,0.913737350469939)) ;
#68562=DIRECTION('center_axis',(1.,2.22044604925031E-16,0.)) ;
#68563=DIRECTION('ref_axis',(1.00806141154385E-16,-0.453990499739547,0.891006524188368)) ;
#68564=DIRECTION('center_axis',(-6.86155564311058E-17,0.309016994374948,
-0.951056516295154)) ;
#68565=DIRECTION('ref_axis',(0.707106781186557,-0.672498511963948,-0.218508012224408)) ;
#68566=DIRECTION('',(6.86155564311058E-17,-0.309016994374947,0.951056516295154)) ;
#68567=DIRECTION('',(-6.86155564311058E-17,0.309016994374948,-0.951056516295154)) ;
#68568=DIRECTION('center_axis',(1.,2.22044604925031E-16,0.)) ;
#68569=DIRECTION('ref_axis',(0.,-0.309016994374926,0.95105651629516)) ;
#68570=DIRECTION('center_axis',(-1.,-2.22044604925031E-16,0.)) ;
#68571=DIRECTION('ref_axis',(6.86155564311052E-17,-0.309016994374945,0.951056516295154)) ;
#68572=DIRECTION('center_axis',(1.,2.22044604925031E-16,0.)) ;
#68573=DIRECTION('ref_axis',(6.86155564311052E-17,-0.309016994374945,0.951056516295154)) ;
#68574=DIRECTION('center_axis',(6.86155564311058E-17,-0.309016994374948,
0.951056516295154)) ;
#68575=DIRECTION('ref_axis',(0.707106781186557,0.672498511963948,0.218508012224408)) ;
#68576=DIRECTION('',(-6.86155564311058E-17,0.309016994374948,-0.951056516295154)) ;
#68577=DIRECTION('',(6.86155564311058E-17,-0.309016994374948,0.951056516295154)) ;
#68578=DIRECTION('center_axis',(1.,2.22044604925031E-16,0.)) ;
#68579=DIRECTION('ref_axis',(0.,0.,-1.)) ;
#68580=DIRECTION('center_axis',(1.,2.22044604925031E-16,0.)) ;
#68581=DIRECTION('ref_axis',(9.02179155423715E-17,-0.406305370818768,0.913737350469939)) ;
#68582=DIRECTION('center_axis',(1.,2.22044604925031E-16,0.)) ;
#68583=DIRECTION('ref_axis',(3.47354289865169E-17,-0.156434465040232,0.987688340595138)) ;
#68584=DIRECTION('center_axis',(-2.46519032881566E-32,1.11022302462516E-16,
-1.)) ;
#68585=DIRECTION('ref_axis',(0.707106781186569,-0.707106781186526,-7.85046229341866E-17)) ;
#68586=DIRECTION('',(2.46519032881566E-32,-1.11022302462516E-16,1.)) ;
#68587=DIRECTION('',(-2.46519032881566E-32,1.11022302462516E-16,-1.)) ;
#68588=DIRECTION('center_axis',(1.,2.22044604925031E-16,0.)) ;
#68589=DIRECTION('ref_axis',(0.,-1.13686837721616E-13,1.)) ;
#68590=DIRECTION('center_axis',(-1.,-2.22044604925031E-16,0.)) ;
#68591=DIRECTION('ref_axis',(0.,0.,1.)) ;
#68592=DIRECTION('center_axis',(1.,2.22044604925031E-16,0.)) ;
#68593=DIRECTION('ref_axis',(0.,0.,1.)) ;
#68594=DIRECTION('center_axis',(2.46519032881566E-32,-1.11022302462516E-16,
1.)) ;
#68595=DIRECTION('ref_axis',(0.707106781186589,0.707106781186506,7.85046229341844E-17)) ;
#68596=DIRECTION('',(-2.46519032881566E-32,1.11022302462516E-16,-1.)) ;
#68597=DIRECTION('',(2.46519032881566E-32,-1.11022302462516E-16,1.)) ;
#68598=DIRECTION('center_axis',(1.,2.22044604925031E-16,0.)) ;
#68599=DIRECTION('ref_axis',(0.,0.,-1.)) ;
#68600=DIRECTION('center_axis',(1.,2.22044604925031E-16,0.)) ;
#68601=DIRECTION('ref_axis',(9.02179155423715E-17,-0.406305370818768,0.913737350469939)) ;
#68602=DIRECTION('center_axis',(1.,2.22044604925031E-16,0.)) ;
#68603=DIRECTION('ref_axis',(-3.47354289865171E-17,0.156434465040233,0.987688340595137)) ;
#68604=DIRECTION('center_axis',(6.86155564311058E-17,-0.309016994374947,
-0.951056516295154)) ;
#68605=DIRECTION('ref_axis',(0.707106781186557,-0.672498511963948,0.218508012224407)) ;
#68606=DIRECTION('',(-6.86155564311058E-17,0.309016994374947,0.951056516295154)) ;
#68607=DIRECTION('',(6.86155564311058E-17,-0.309016994374947,-0.951056516295154)) ;
#68608=DIRECTION('center_axis',(1.,2.22044604925031E-16,0.)) ;
#68609=DIRECTION('ref_axis',(0.,0.309016994374757,0.951056516295215)) ;
#68610=DIRECTION('center_axis',(-1.,-2.22044604925031E-16,0.)) ;
#68611=DIRECTION('ref_axis',(-6.86155564311052E-17,0.309016994374945,0.951056516295154)) ;
#68612=DIRECTION('center_axis',(1.,2.22044604925031E-16,0.)) ;
#68613=DIRECTION('ref_axis',(-6.86155564311052E-17,0.309016994374945,0.951056516295154)) ;
#68614=DIRECTION('center_axis',(-6.86155564311058E-17,0.309016994374947,
0.951056516295154)) ;
#68615=DIRECTION('ref_axis',(0.707106781186557,0.672498511963948,-0.218508012224407)) ;
#68616=DIRECTION('',(6.86155564311058E-17,-0.309016994374947,-0.951056516295154)) ;
#68617=DIRECTION('',(-6.86155564311058E-17,0.309016994374947,0.951056516295154)) ;
#68618=DIRECTION('center_axis',(1.,2.22044604925031E-16,0.)) ;
#68619=DIRECTION('ref_axis',(0.,0.,-1.)) ;
#68620=DIRECTION('center_axis',(1.,2.22044604925031E-16,0.)) ;
#68621=DIRECTION('ref_axis',(9.02179155423715E-17,-0.406305370818768,0.913737350469939)) ;
#68622=DIRECTION('center_axis',(1.,2.22044604925031E-16,0.)) ;
#68623=DIRECTION('ref_axis',(-1.00806141154386E-16,0.453990499739549,0.891006524188367)) ;
#68624=DIRECTION('center_axis',(1.30514544126042E-16,-0.587785252292473,
-0.809016994374948)) ;
#68625=DIRECTION('ref_axis',(0.707106781186534,-0.572061402817695,0.415626937777461)) ;
#68626=DIRECTION('',(-1.30514544126042E-16,0.587785252292473,0.809016994374948)) ;
#68627=DIRECTION('',(1.30514544126042E-16,-0.587785252292473,-0.809016994374947)) ;
#68628=DIRECTION('center_axis',(1.,2.22044604925031E-16,0.)) ;
#68629=DIRECTION('ref_axis',(0.,0.587785252292692,0.809016994374789)) ;
#68630=DIRECTION('center_axis',(-1.,-2.22044604925031E-16,0.)) ;
#68631=DIRECTION('ref_axis',(-1.30514544126041E-16,0.587785252292468,0.809016994374951)) ;
#68632=DIRECTION('center_axis',(1.,2.22044604925031E-16,0.)) ;
#68633=DIRECTION('ref_axis',(-1.30514544126041E-16,0.587785252292468,0.809016994374951)) ;
#68634=DIRECTION('center_axis',(-1.30514544126042E-16,0.587785252292473,
0.809016994374948)) ;
#68635=DIRECTION('ref_axis',(0.707106781186568,0.572061402817668,-0.415626937777441)) ;
#68636=DIRECTION('',(1.30514544126042E-16,-0.587785252292473,-0.809016994374947)) ;
#68637=DIRECTION('',(-1.30514544126042E-16,0.587785252292473,0.809016994374947)) ;
#68638=DIRECTION('center_axis',(1.,2.22044604925031E-16,0.)) ;
#68639=DIRECTION('ref_axis',(0.,0.,-1.)) ;
#68640=DIRECTION('center_axis',(1.,2.22044604925031E-16,0.)) ;
#68641=DIRECTION('ref_axis',(9.02179155423715E-17,-0.406305370818768,0.913737350469939)) ;
#68642=DIRECTION('center_axis',(1.,2.22044604925031E-16,0.)) ;
#68643=DIRECTION('ref_axis',(-1.57009245868378E-16,0.70710678118655,0.707106781186545)) ;
#68644=DIRECTION('center_axis',(1.79637858893621E-16,-0.809016994374947,
-0.587785252292473)) ;
#68645=DIRECTION('ref_axis',(0.707106781186551,-0.415626937777451,0.572061402817682)) ;
#68646=DIRECTION('',(-1.79637858893621E-16,0.809016994374947,0.587785252292473)) ;
#68647=DIRECTION('',(1.79637858893621E-16,-0.809016994374947,-0.587785252292473)) ;
#68648=DIRECTION('center_axis',(1.,2.22044604925031E-16,0.)) ;
#68649=DIRECTION('ref_axis',(0.,0.809016994375189,0.58778525229214)) ;
#68650=DIRECTION('center_axis',(-1.,-2.22044604925031E-16,0.)) ;
#68651=DIRECTION('ref_axis',(-1.79637858893621E-16,0.809016994374947,0.587785252292474)) ;
#68652=DIRECTION('center_axis',(1.,2.22044604925031E-16,0.)) ;
#68653=DIRECTION('ref_axis',(-1.79637858893621E-16,0.809016994374947,0.587785252292474)) ;
#68654=DIRECTION('center_axis',(-1.79637858893621E-16,0.809016994374947,
0.587785252292473)) ;
#68655=DIRECTION('ref_axis',(0.707106781186592,0.415626937777427,-0.572061402817648)) ;
#68656=DIRECTION('',(1.79637858893621E-16,-0.809016994374947,-0.587785252292473)) ;
#68657=DIRECTION('',(-1.79637858893621E-16,0.809016994374947,0.587785252292473)) ;
#68658=DIRECTION('center_axis',(1.,2.22044604925031E-16,0.)) ;
#68659=DIRECTION('ref_axis',(0.,0.,-1.)) ;
#68660=DIRECTION('center_axis',(1.,2.22044604925031E-16,0.)) ;
#68661=DIRECTION('ref_axis',(9.02179155423715E-17,-0.406305370818768,0.913737350469939)) ;
#68662=DIRECTION('center_axis',(1.,2.22044604925031E-16,0.)) ;
#68663=DIRECTION('ref_axis',(-1.97843191649031E-16,0.891006524188368,0.453990499739546)) ;
#68664=DIRECTION('center_axis',(2.11176968422134E-16,-0.951056516295154,
-0.309016994374948)) ;
#68665=DIRECTION('ref_axis',(0.707106781186583,-0.2185080122244,0.672498511963923)) ;
#68666=DIRECTION('',(-2.11176968422134E-16,0.951056516295153,0.309016994374948)) ;
#68667=DIRECTION('',(2.11176968422134E-16,-0.951056516295153,-0.309016994374948)) ;
#68668=DIRECTION('center_axis',(1.,2.22044604925031E-16,0.)) ;
#68669=DIRECTION('ref_axis',(0.,0.951056516295183,0.309016994374858)) ;
#68670=DIRECTION('center_axis',(-1.,-2.22044604925031E-16,0.)) ;
#68671=DIRECTION('ref_axis',(-2.11176968422134E-16,0.951056516295153,0.309016994374948)) ;
#68672=DIRECTION('center_axis',(1.,2.22044604925031E-16,0.)) ;
#68673=DIRECTION('ref_axis',(-2.11176968422134E-16,0.951056516295153,0.309016994374948)) ;
#68674=DIRECTION('center_axis',(-2.11176968422134E-16,0.951056516295154,
0.309016994374948)) ;
#68675=DIRECTION('ref_axis',(0.707106781186563,0.218508012224406,-0.672498511963943)) ;
#68676=DIRECTION('',(2.11176968422134E-16,-0.951056516295153,-0.309016994374948)) ;
#68677=DIRECTION('',(-2.11176968422134E-16,0.951056516295153,0.309016994374948)) ;
#68678=DIRECTION('center_axis',(1.,2.22044604925031E-16,0.)) ;
#68679=DIRECTION('ref_axis',(0.,0.,-1.)) ;
#68680=DIRECTION('center_axis',(1.,2.22044604925031E-16,0.)) ;
#68681=DIRECTION('ref_axis',(9.02179155423715E-17,-0.406305370818768,0.913737350469939)) ;
#68682=DIRECTION('center_axis',(1.,2.22044604925031E-16,0.)) ;
#68683=DIRECTION('ref_axis',(-2.19310867376507E-16,0.987688340595138,0.15643446504023)) ;
#68684=DIRECTION('center_axis',(2.22044604925031E-16,-1.,-2.22044604925031E-16)) ;
#68685=DIRECTION('ref_axis',(0.707106781186568,9.08458920382451E-30,0.707106781186527)) ;
#68686=DIRECTION('',(-2.22044604925031E-16,1.,2.22044604925031E-16)) ;
#68687=DIRECTION('',(2.22044604925031E-16,-1.,-2.22044604925031E-16)) ;
#68688=DIRECTION('center_axis',(1.,2.22044604925031E-16,0.)) ;
#68689=DIRECTION('ref_axis',(0.,1.,-1.49213974509621E-13)) ;
#68690=DIRECTION('center_axis',(-1.,-2.22044604925031E-16,0.)) ;
#68691=DIRECTION('ref_axis',(-2.22044604925031E-16,1.,0.)) ;
#68692=DIRECTION('center_axis',(1.,2.22044604925031E-16,0.)) ;
#68693=DIRECTION('ref_axis',(-2.22044604925031E-16,1.,0.)) ;
#68694=DIRECTION('center_axis',(-2.22044604925031E-16,1.,2.22044604925031E-16)) ;
#68695=DIRECTION('ref_axis',(0.707106781186568,3.14018491736755E-16,-0.707106781186527)) ;
#68696=DIRECTION('',(2.22044604925031E-16,-1.,-2.22044604925031E-16)) ;
#68697=DIRECTION('',(-2.22044604925031E-16,1.,2.22044604925031E-16)) ;
#68698=DIRECTION('center_axis',(1.,2.22044604925031E-16,0.)) ;
#68699=DIRECTION('ref_axis',(0.,0.,-1.)) ;
#68700=DIRECTION('center_axis',(1.,2.22044604925031E-16,0.)) ;
#68701=DIRECTION('ref_axis',(9.02179155423715E-17,-0.406305370818768,0.913737350469939)) ;
#68702=DIRECTION('center_axis',(1.,2.22044604925031E-16,0.)) ;
#68703=DIRECTION('ref_axis',(-2.19310867376507E-16,0.987688340595138,-0.156434465040229)) ;
#68704=DIRECTION('center_axis',(2.11176968422134E-16,-0.951056516295154,
0.309016994374947)) ;
#68705=DIRECTION('ref_axis',(0.707106781186563,0.218508012224406,0.672498511963943)) ;
#68706=DIRECTION('',(-2.11176968422134E-16,0.951056516295154,-0.309016994374947)) ;
#68707=DIRECTION('',(2.11176968422134E-16,-0.951056516295154,0.309016994374947)) ;
#68708=DIRECTION('center_axis',(1.,2.22044604925031E-16,0.)) ;
#68709=DIRECTION('ref_axis',(0.,0.,-1.)) ;
#68710=DIRECTION('center_axis',(-1.,-2.22044604925031E-16,0.)) ;
#68711=DIRECTION('ref_axis',(-2.11176968422134E-16,0.951056516295153,-0.309016994374948)) ;
#68712=DIRECTION('center_axis',(1.,2.22044604925031E-16,0.)) ;
#68713=DIRECTION('ref_axis',(-2.11176968422134E-16,0.951056516295153,-0.309016994374948)) ;
#68714=DIRECTION('center_axis',(-2.11176968422134E-16,0.951056516295154,
-0.309016994374947)) ;
#68715=DIRECTION('ref_axis',(0.707106781186563,-0.218508012224405,-0.672498511963943)) ;
#68716=DIRECTION('',(2.11176968422134E-16,-0.951056516295154,0.309016994374947)) ;
#68717=DIRECTION('',(-2.11176968422134E-16,0.951056516295154,-0.309016994374947)) ;
#68718=DIRECTION('center_axis',(1.,2.22044604925031E-16,0.)) ;
#68719=DIRECTION('ref_axis',(0.,0.,-1.)) ;
#68720=DIRECTION('center_axis',(1.,2.22044604925031E-16,0.)) ;
#68721=DIRECTION('ref_axis',(9.02179155423715E-17,-0.406305370818768,0.913737350469939)) ;
#68722=DIRECTION('center_axis',(1.,2.22044604925031E-16,0.)) ;
#68723=DIRECTION('ref_axis',(-1.97843191649031E-16,0.891006524188368,-0.453990499739547)) ;
#68724=DIRECTION('center_axis',(1.79637858893621E-16,-0.809016994374948,
0.587785252292473)) ;
#68725=DIRECTION('ref_axis',(0.707106781186551,0.415626937777452,0.572061402817682)) ;
#68726=DIRECTION('',(-1.79637858893621E-16,0.809016994374948,-0.587785252292473)) ;
#68727=DIRECTION('',(1.79637858893621E-16,-0.809016994374948,0.587785252292473)) ;
#68728=DIRECTION('center_axis',(1.,2.22044604925031E-16,0.)) ;
#68729=DIRECTION('ref_axis',(0.,0.,-1.)) ;
#68730=DIRECTION('center_axis',(-1.,-2.22044604925031E-16,0.)) ;
#68731=DIRECTION('ref_axis',(-1.79637858893621E-16,0.809016994374947,-0.587785252292474)) ;
#68732=DIRECTION('center_axis',(1.,2.22044604925031E-16,0.)) ;
#68733=DIRECTION('ref_axis',(-1.79637858893621E-16,0.809016994374947,-0.587785252292474)) ;
#68734=DIRECTION('center_axis',(-1.79637858893621E-16,0.809016994374948,
-0.587785252292473)) ;
#68735=DIRECTION('ref_axis',(0.707106781186575,-0.415626937777437,-0.572061402817662)) ;
#68736=DIRECTION('',(1.79637858893621E-16,-0.809016994374948,0.587785252292473)) ;
#68737=DIRECTION('',(-1.79637858893621E-16,0.809016994374948,-0.587785252292473)) ;
#68738=DIRECTION('center_axis',(1.,2.22044604925031E-16,0.)) ;
#68739=DIRECTION('ref_axis',(0.,0.,-1.)) ;
#68740=DIRECTION('center_axis',(1.,2.22044604925031E-16,0.)) ;
#68741=DIRECTION('ref_axis',(9.02179155423715E-17,-0.406305370818768,0.913737350469939)) ;
#68742=DIRECTION('center_axis',(1.,2.22044604925031E-16,0.)) ;
#68743=DIRECTION('ref_axis',(-1.57009245868377E-16,0.707106781186547,-0.707106781186547)) ;
#68744=DIRECTION('center_axis',(1.30514544126042E-16,-0.587785252292473,
0.809016994374947)) ;
#68745=DIRECTION('ref_axis',(0.707106781186546,0.572061402817686,0.415626937777454)) ;
#68746=DIRECTION('',(-1.30514544126042E-16,0.587785252292473,-0.809016994374947)) ;
#68747=DIRECTION('',(1.30514544126042E-16,-0.587785252292473,0.809016994374947)) ;
#68748=DIRECTION('center_axis',(1.,2.22044604925031E-16,0.)) ;
#68749=DIRECTION('ref_axis',(0.,0.,-1.)) ;
#68750=DIRECTION('center_axis',(-1.,-2.22044604925031E-16,0.)) ;
#68751=DIRECTION('ref_axis',(-1.30514544126041E-16,0.587785252292468,-0.809016994374951)) ;
#68752=DIRECTION('center_axis',(1.,2.22044604925031E-16,0.)) ;
#68753=DIRECTION('ref_axis',(-1.30514544126041E-16,0.587785252292468,-0.809016994374951)) ;
#68754=DIRECTION('center_axis',(-1.30514544126042E-16,0.587785252292473,
-0.809016994374947)) ;
#68755=DIRECTION('ref_axis',(0.707106781186534,-0.572061402817695,-0.415626937777462)) ;
#68756=DIRECTION('',(1.30514544126042E-16,-0.587785252292473,0.809016994374947)) ;
#68757=DIRECTION('',(-1.30514544126042E-16,0.587785252292473,-0.809016994374947)) ;
#68758=DIRECTION('center_axis',(1.,2.22044604925031E-16,0.)) ;
#68759=DIRECTION('ref_axis',(0.,0.,-1.)) ;
#68760=DIRECTION('center_axis',(1.,2.22044604925031E-16,0.)) ;
#68761=DIRECTION('ref_axis',(9.02179155423715E-17,-0.406305370818768,0.913737350469939)) ;
#68762=DIRECTION('center_axis',(1.,2.22044604925031E-16,0.)) ;
#68763=DIRECTION('ref_axis',(-1.00806141154385E-16,0.453990499739547,-0.891006524188368)) ;
#68764=DIRECTION('center_axis',(6.86155564311059E-17,-0.309016994374948,
0.951056516295154)) ;
#68765=DIRECTION('ref_axis',(0.707106781186557,0.672498511963948,0.218508012224408)) ;
#68766=DIRECTION('',(6.86155564311059E-17,-0.309016994374948,0.951056516295153)) ;
#68767=DIRECTION('',(-6.86155564311059E-17,0.309016994374948,-0.951056516295153)) ;
#68768=DIRECTION('center_axis',(1.,2.22044604925031E-16,0.)) ;
#68769=DIRECTION('ref_axis',(0.,0.,-1.)) ;
#68770=DIRECTION('center_axis',(1.,2.22044604925031E-16,0.)) ;
#68771=DIRECTION('ref_axis',(-6.86155564311052E-17,0.309016994374945,-0.951056516295154)) ;
#68772=DIRECTION('center_axis',(-1.,-2.22044604925031E-16,0.)) ;
#68773=DIRECTION('ref_axis',(-6.86155564311052E-17,0.309016994374945,-0.951056516295154)) ;
#68774=DIRECTION('center_axis',(-6.86155564311059E-17,0.309016994374948,
-0.951056516295154)) ;
#68775=DIRECTION('ref_axis',(0.707106781186557,-0.672498511963948,-0.218508012224408)) ;
#68776=DIRECTION('',(-6.86155564311059E-17,0.309016994374948,-0.951056516295153)) ;
#68777=DIRECTION('',(6.86155564311059E-17,-0.309016994374948,0.951056516295153)) ;
#68778=DIRECTION('center_axis',(1.,2.22044604925031E-16,0.)) ;
#68779=DIRECTION('ref_axis',(0.,0.,-1.)) ;
#68780=DIRECTION('center_axis',(1.,2.22044604925031E-16,0.)) ;
#68781=DIRECTION('ref_axis',(-3.47354289865169E-17,0.156434465040232,-0.987688340595138)) ;
#68782=DIRECTION('center_axis',(1.,2.22044604925031E-16,0.)) ;
#68783=DIRECTION('ref_axis',(9.02179155423715E-17,-0.406305370818768,0.913737350469939)) ;
#68784=DIRECTION('center_axis',(0.,0.,1.)) ;
#68785=DIRECTION('ref_axis',(0.707106781186589,0.707106781186506,0.)) ;
#68786=DIRECTION('',(0.,0.,1.)) ;
#68787=DIRECTION('',(0.,0.,-1.)) ;
#68788=DIRECTION('center_axis',(1.,2.22044604925031E-16,0.)) ;
#68789=DIRECTION('ref_axis',(0.,0.,-1.)) ;
#68790=DIRECTION('center_axis',(1.,2.22044604925031E-16,0.)) ;
#68791=DIRECTION('ref_axis',(0.,0.,-1.)) ;
#68792=DIRECTION('center_axis',(-1.,-2.22044604925031E-16,0.)) ;
#68793=DIRECTION('ref_axis',(0.,0.,-1.)) ;
#68794=DIRECTION('center_axis',(0.,0.,-1.)) ;
#68795=DIRECTION('ref_axis',(0.707106781186569,-0.707106781186526,0.)) ;
#68796=DIRECTION('',(0.,0.,-1.)) ;
#68797=DIRECTION('',(0.,0.,1.)) ;
#68798=DIRECTION('center_axis',(1.,2.22044604925031E-16,0.)) ;
#68799=DIRECTION('ref_axis',(0.,0.,-1.)) ;
#68800=DIRECTION('center_axis',(1.,2.22044604925031E-16,0.)) ;
#68801=DIRECTION('ref_axis',(3.47354289865167E-17,-0.156434465040231,-0.987688340595138)) ;
#68802=DIRECTION('center_axis',(1.,2.22044604925031E-16,0.)) ;
#68803=DIRECTION('ref_axis',(9.02179155423715E-17,-0.406305370818768,0.913737350469939)) ;
#68804=DIRECTION('center_axis',(-6.86155564311058E-17,0.309016994374947,
0.951056516295154)) ;
#68805=DIRECTION('ref_axis',(0.707106781186557,0.672498511963948,-0.218508012224407)) ;
#68806=DIRECTION('',(-6.86155564311058E-17,0.309016994374947,0.951056516295154)) ;
#68807=DIRECTION('',(6.86155564311058E-17,-0.309016994374947,-0.951056516295154)) ;
#68808=DIRECTION('center_axis',(1.,2.22044604925031E-16,0.)) ;
#68809=DIRECTION('ref_axis',(0.,0.,-1.)) ;
#68810=DIRECTION('center_axis',(1.,2.22044604925031E-16,0.)) ;
#68811=DIRECTION('ref_axis',(6.86155564311052E-17,-0.309016994374945,-0.951056516295154)) ;
#68812=DIRECTION('center_axis',(-1.,-2.22044604925031E-16,0.)) ;
#68813=DIRECTION('ref_axis',(6.86155564311052E-17,-0.309016994374945,-0.951056516295154)) ;
#68814=DIRECTION('center_axis',(6.86155564311058E-17,-0.309016994374947,
-0.951056516295154)) ;
#68815=DIRECTION('ref_axis',(0.707106781186557,-0.672498511963948,0.218508012224407)) ;
#68816=DIRECTION('',(6.86155564311058E-17,-0.309016994374947,-0.951056516295154)) ;
#68817=DIRECTION('',(-6.86155564311058E-17,0.309016994374947,0.951056516295154)) ;
#68818=DIRECTION('center_axis',(1.,2.22044604925031E-16,0.)) ;
#68819=DIRECTION('ref_axis',(0.,0.,-1.)) ;
#68820=DIRECTION('center_axis',(1.,2.22044604925031E-16,0.)) ;
#68821=DIRECTION('ref_axis',(1.00806141154385E-16,-0.453990499739546,-0.891006524188368)) ;
#68822=DIRECTION('center_axis',(1.,2.22044604925031E-16,0.)) ;
#68823=DIRECTION('ref_axis',(9.02179155423715E-17,-0.406305370818768,0.913737350469939)) ;
#68824=DIRECTION('center_axis',(-1.30514544126042E-16,0.587785252292473,
0.809016994374948)) ;
#68825=DIRECTION('ref_axis',(0.707106781186551,0.572061402817682,-0.415626937777451)) ;
#68826=DIRECTION('',(-1.30514544126042E-16,0.587785252292473,0.809016994374947)) ;
#68827=DIRECTION('',(1.30514544126042E-16,-0.587785252292473,-0.809016994374947)) ;
#68828=DIRECTION('center_axis',(1.,2.22044604925031E-16,0.)) ;
#68829=DIRECTION('ref_axis',(0.,0.,-1.)) ;
#68830=DIRECTION('center_axis',(1.,2.22044604925031E-16,0.)) ;
#68831=DIRECTION('ref_axis',(1.30514544126042E-16,-0.587785252292474,-0.809016994374947)) ;
#68832=DIRECTION('center_axis',(-1.,-2.22044604925031E-16,0.)) ;
#68833=DIRECTION('ref_axis',(1.30514544126042E-16,-0.587785252292474,-0.809016994374947)) ;
#68834=DIRECTION('center_axis',(1.30514544126042E-16,-0.587785252292473,
-0.809016994374948)) ;
#68835=DIRECTION('ref_axis',(0.707106781186563,-0.572061402817672,0.415626937777444)) ;
#68836=DIRECTION('',(1.30514544126042E-16,-0.587785252292473,-0.809016994374947)) ;
#68837=DIRECTION('',(-1.30514544126042E-16,0.587785252292473,0.809016994374947)) ;
#68838=DIRECTION('center_axis',(1.,2.22044604925031E-16,0.)) ;
#68839=DIRECTION('ref_axis',(0.,0.,-1.)) ;
#68840=DIRECTION('center_axis',(1.,2.22044604925031E-16,0.)) ;
#68841=DIRECTION('ref_axis',(1.57009245868377E-16,-0.707106781186547,-0.707106781186548)) ;
#68842=DIRECTION('center_axis',(1.,2.22044604925031E-16,0.)) ;
#68843=DIRECTION('ref_axis',(9.02179155423715E-17,-0.406305370818768,0.913737350469939)) ;
#68844=DIRECTION('center_axis',(-1.79637858893621E-16,0.809016994374947,
0.587785252292473)) ;
#68845=DIRECTION('ref_axis',(0.707106781186568,0.415626937777442,-0.572061402817668)) ;
#68846=DIRECTION('',(-1.79637858893621E-16,0.809016994374947,0.587785252292473)) ;
#68847=DIRECTION('',(1.79637858893621E-16,-0.809016994374947,-0.587785252292473)) ;
#68848=DIRECTION('center_axis',(1.,2.22044604925031E-16,0.)) ;
#68849=DIRECTION('ref_axis',(0.,0.,-1.)) ;
#68850=DIRECTION('center_axis',(1.,2.22044604925031E-16,0.)) ;
#68851=DIRECTION('ref_axis',(1.79637858893621E-16,-0.809016994374947,-0.587785252292474)) ;
#68852=DIRECTION('center_axis',(-1.,-2.22044604925031E-16,0.)) ;
#68853=DIRECTION('ref_axis',(1.79637858893621E-16,-0.809016994374947,-0.587785252292474)) ;
#68854=DIRECTION('center_axis',(1.79637858893621E-16,-0.809016994374947,
-0.587785252292473)) ;
#68855=DIRECTION('ref_axis',(0.707106781186563,-0.415626937777444,0.572061402817672)) ;
#68856=DIRECTION('',(1.79637858893621E-16,-0.809016994374947,-0.587785252292473)) ;
#68857=DIRECTION('',(-1.79637858893621E-16,0.809016994374947,0.587785252292473)) ;
#68858=DIRECTION('center_axis',(1.,2.22044604925031E-16,0.)) ;
#68859=DIRECTION('ref_axis',(0.,0.,-1.)) ;
#68860=DIRECTION('center_axis',(1.,2.22044604925031E-16,0.)) ;
#68861=DIRECTION('ref_axis',(1.97843191649031E-16,-0.891006524188368,-0.453990499739547)) ;
#68862=DIRECTION('center_axis',(1.,2.22044604925031E-16,0.)) ;
#68863=DIRECTION('ref_axis',(9.02179155423715E-17,-0.406305370818768,0.913737350469939)) ;
#68864=DIRECTION('center_axis',(-2.11176968422134E-16,0.951056516295154,
0.309016994374948)) ;
#68865=DIRECTION('ref_axis',(0.707106781186557,0.218508012224408,-0.672498511963948)) ;
#68866=DIRECTION('',(-2.11176968422134E-16,0.951056516295154,0.309016994374948)) ;
#68867=DIRECTION('',(2.11176968422134E-16,-0.951056516295154,-0.309016994374948)) ;
#68868=DIRECTION('center_axis',(1.,2.22044604925031E-16,0.)) ;
#68869=DIRECTION('ref_axis',(0.,0.,-1.)) ;
#68870=DIRECTION('center_axis',(1.,2.22044604925031E-16,0.)) ;
#68871=DIRECTION('ref_axis',(2.11176968422134E-16,-0.951056516295154,-0.309016994374945)) ;
#68872=DIRECTION('center_axis',(-1.,-2.22044604925031E-16,0.)) ;
#68873=DIRECTION('ref_axis',(2.11176968422134E-16,-0.951056516295154,-0.309016994374945)) ;
#68874=DIRECTION('center_axis',(2.11176968422134E-16,-0.951056516295154,
-0.309016994374948)) ;
#68875=DIRECTION('ref_axis',(0.707106781186557,-0.218508012224408,0.672498511963948)) ;
#68876=DIRECTION('',(2.11176968422134E-16,-0.951056516295154,-0.309016994374948)) ;
#68877=DIRECTION('',(-2.11176968422134E-16,0.951056516295154,0.309016994374948)) ;
#68878=DIRECTION('center_axis',(1.,2.22044604925031E-16,0.)) ;
#68879=DIRECTION('ref_axis',(0.,0.,-1.)) ;
#68880=DIRECTION('center_axis',(1.,2.22044604925031E-16,0.)) ;
#68881=DIRECTION('ref_axis',(2.19310867376507E-16,-0.987688340595138,-0.156434465040231)) ;
#68882=DIRECTION('center_axis',(1.,2.22044604925031E-16,0.)) ;
#68883=DIRECTION('ref_axis',(9.02179155423715E-17,-0.406305370818768,0.913737350469939)) ;
#68884=DIRECTION('center_axis',(-2.22044604925031E-16,1.,5.55111512312578E-17)) ;
#68885=DIRECTION('ref_axis',(0.707106781186568,1.96261557335475E-16,-0.707106781186527)) ;
#68886=DIRECTION('',(-2.22044604925031E-16,1.,5.55111512312578E-17)) ;
#68887=DIRECTION('',(2.22044604925031E-16,-1.,-5.55111512312578E-17)) ;
#68888=DIRECTION('center_axis',(1.,2.22044604925031E-16,0.)) ;
#68889=DIRECTION('ref_axis',(0.,-1.,4.68958205601666E-13)) ;
#68890=DIRECTION('center_axis',(1.,2.22044604925031E-16,0.)) ;
#68891=DIRECTION('ref_axis',(2.22044604925031E-16,-1.,0.)) ;
#68892=DIRECTION('center_axis',(-1.,-2.22044604925031E-16,0.)) ;
#68893=DIRECTION('ref_axis',(2.22044604925031E-16,-1.,0.)) ;
#68894=DIRECTION('center_axis',(2.22044604925031E-16,-1.,-5.55111512312578E-17)) ;
#68895=DIRECTION('ref_axis',(0.707106781186568,1.17756934401289E-16,0.707106781186527)) ;
#68896=DIRECTION('',(2.22044604925031E-16,-1.,-5.55111512312578E-17)) ;
#68897=DIRECTION('',(-2.22044604925031E-16,1.,5.55111512312578E-17)) ;
#68898=DIRECTION('center_axis',(1.,2.22044604925031E-16,0.)) ;
#68899=DIRECTION('ref_axis',(0.,0.,-1.)) ;
#68900=DIRECTION('center_axis',(1.,2.22044604925031E-16,0.)) ;
#68901=DIRECTION('ref_axis',(2.19310867376507E-16,-0.987688340595138,0.156434465040229)) ;
#68902=DIRECTION('center_axis',(1.,2.22044604925031E-16,0.)) ;
#68903=DIRECTION('ref_axis',(9.02179155423715E-17,-0.406305370818768,0.913737350469939)) ;
#68904=DIRECTION('center_axis',(-2.11176968422134E-16,0.951056516295154,
-0.309016994374947)) ;
#68905=DIRECTION('ref_axis',(0.707106781186557,-0.218508012224407,-0.672498511963949)) ;
#68906=DIRECTION('',(-2.11176968422134E-16,0.951056516295154,-0.309016994374947)) ;
#68907=DIRECTION('',(2.11176968422134E-16,-0.951056516295154,0.309016994374947)) ;
#68908=DIRECTION('center_axis',(1.,2.22044604925031E-16,0.)) ;
#68909=DIRECTION('ref_axis',(0.,-0.95105651629504,0.309016994375296)) ;
#68910=DIRECTION('center_axis',(1.,2.22044604925031E-16,0.)) ;
#68911=DIRECTION('ref_axis',(2.11176968422134E-16,-0.951056516295154,0.309016994374945)) ;
#68912=DIRECTION('center_axis',(-1.,-2.22044604925031E-16,0.)) ;
#68913=DIRECTION('ref_axis',(2.11176968422134E-16,-0.951056516295154,0.309016994374945)) ;
#68914=DIRECTION('center_axis',(2.11176968422134E-16,-0.951056516295154,
0.309016994374947)) ;
#68915=DIRECTION('ref_axis',(0.707106781186557,0.218508012224407,0.672498511963948)) ;
#68916=DIRECTION('',(2.11176968422134E-16,-0.951056516295154,0.309016994374947)) ;
#68917=DIRECTION('',(-2.11176968422134E-16,0.951056516295154,-0.309016994374947)) ;
#68918=DIRECTION('center_axis',(1.,2.22044604925031E-16,0.)) ;
#68919=DIRECTION('ref_axis',(0.,0.,-1.)) ;
#68920=DIRECTION('center_axis',(1.,2.22044604925031E-16,0.)) ;
#68921=DIRECTION('ref_axis',(1.97843191649031E-16,-0.891006524188369,0.453990499739545)) ;
#68922=DIRECTION('center_axis',(1.,2.22044604925031E-16,0.)) ;
#68923=DIRECTION('ref_axis',(9.02179155423715E-17,-0.406305370818768,0.913737350469939)) ;
#68924=DIRECTION('center_axis',(-1.79637858893621E-16,0.809016994374948,
-0.587785252292473)) ;
#68925=DIRECTION('ref_axis',(0.707106781186563,-0.415626937777444,-0.572061402817672)) ;
#68926=DIRECTION('',(-1.79637858893621E-16,0.809016994374947,-0.587785252292473)) ;
#68927=DIRECTION('',(1.79637858893621E-16,-0.809016994374947,0.587785252292473)) ;
#68928=DIRECTION('center_axis',(1.,2.22044604925031E-16,0.)) ;
#68929=DIRECTION('ref_axis',(0.,-0.809016994374969,0.587785252292443)) ;
#68930=DIRECTION('center_axis',(1.,2.22044604925031E-16,0.)) ;
#68931=DIRECTION('ref_axis',(1.79637858893621E-16,-0.809016994374947,0.587785252292474)) ;
#68932=DIRECTION('center_axis',(-1.,-2.22044604925031E-16,0.)) ;
#68933=DIRECTION('ref_axis',(1.79637858893621E-16,-0.809016994374947,0.587785252292474)) ;
#68934=DIRECTION('center_axis',(1.79637858893621E-16,-0.809016994374948,
0.587785252292473)) ;
#68935=DIRECTION('ref_axis',(0.707106781186563,0.415626937777444,0.572061402817672)) ;
#68936=DIRECTION('',(1.79637858893621E-16,-0.809016994374947,0.587785252292473)) ;
#68937=DIRECTION('',(-1.79637858893621E-16,0.809016994374947,-0.587785252292473)) ;
#68938=DIRECTION('center_axis',(1.,2.22044604925031E-16,0.)) ;
#68939=DIRECTION('ref_axis',(0.,0.,-1.)) ;
#68940=DIRECTION('center_axis',(1.,2.22044604925031E-16,0.)) ;
#68941=DIRECTION('ref_axis',(1.57009245868377E-16,-0.707106781186548,0.707106781186547)) ;
#68942=DIRECTION('center_axis',(1.,2.22044604925031E-16,0.)) ;
#68943=DIRECTION('ref_axis',(9.02179155423715E-17,-0.406305370818768,0.913737350469939)) ;
#68944=DIRECTION('center_axis',(-1.30514544126042E-16,0.587785252292473,
-0.809016994374947)) ;
#68945=DIRECTION('ref_axis',(0.707106781186551,-0.572061402817681,-0.415626937777452)) ;
#68946=DIRECTION('',(-1.30514544126042E-16,0.587785252292473,-0.809016994374947)) ;
#68947=DIRECTION('',(1.30514544126042E-16,-0.587785252292473,0.809016994374947)) ;
#68948=DIRECTION('center_axis',(1.,2.22044604925031E-16,0.)) ;
#68949=DIRECTION('ref_axis',(0.,-0.587785252292056,0.809016994375251)) ;
#68950=DIRECTION('center_axis',(1.,2.22044604925031E-16,0.)) ;
#68951=DIRECTION('ref_axis',(1.30514544126042E-16,-0.587785252292474,0.809016994374947)) ;
#68952=DIRECTION('center_axis',(-1.,-2.22044604925031E-16,0.)) ;
#68953=DIRECTION('ref_axis',(1.30514544126042E-16,-0.587785252292474,0.809016994374947)) ;
#68954=DIRECTION('center_axis',(1.30514544126042E-16,-0.587785252292473,
0.809016994374947)) ;
#68955=DIRECTION('ref_axis',(0.707106781186563,0.572061402817672,0.415626937777444)) ;
#68956=DIRECTION('',(1.30514544126042E-16,-0.587785252292473,0.809016994374947)) ;
#68957=DIRECTION('',(-1.30514544126042E-16,0.587785252292473,-0.809016994374947)) ;
#68958=DIRECTION('center_axis',(-2.11176968422134E-16,0.951056516295154,
0.309016994374948)) ;
#68959=DIRECTION('ref_axis',(6.86155564311059E-17,-0.309016994374948,0.951056516295153)) ;
#68960=DIRECTION('',(1.,2.22044604925031E-16,0.)) ;
#68961=DIRECTION('',(-6.86155564311059E-17,0.309016994374948,-0.951056516295153)) ;
#68962=DIRECTION('',(-1.,-2.22044604925031E-16,0.)) ;
#68963=DIRECTION('center_axis',(1.,2.22044604925031E-16,0.)) ;
#68964=DIRECTION('ref_axis',(-6.8615556431103E-17,0.309016994374935,-0.951056516295158)) ;
#68965=DIRECTION('',(1.,2.22044604925031E-16,0.)) ;
#68966=DIRECTION('center_axis',(-1.,-2.22044604925031E-16,0.)) ;
#68967=DIRECTION('ref_axis',(-6.86155564311052E-17,0.309016994374945,-0.951056516295154)) ;
#68968=DIRECTION('center_axis',(2.11176968422134E-16,-0.951056516295154,
-0.309016994374948)) ;
#68969=DIRECTION('ref_axis',(-6.86155564311059E-17,0.309016994374948,-0.951056516295153)) ;
#68970=DIRECTION('',(1.,2.22044604925031E-16,0.)) ;
#68971=DIRECTION('',(6.86155564311059E-17,-0.309016994374948,0.951056516295153)) ;
#68972=DIRECTION('center_axis',(1.,2.22044604925031E-16,0.)) ;
#68973=DIRECTION('ref_axis',(2.22044604925031E-16,-1.,0.)) ;
#68974=DIRECTION('',(-1.,-2.22044604925031E-16,0.)) ;
#68975=DIRECTION('center_axis',(-1.,-2.22044604925031E-16,0.)) ;
#68976=DIRECTION('ref_axis',(-3.47354289865169E-17,0.156434465040232,-0.987688340595138)) ;
#68977=DIRECTION('center_axis',(-2.22044604925031E-16,1.,0.)) ;
#68978=DIRECTION('ref_axis',(0.,0.,1.)) ;
#68979=DIRECTION('',(1.,2.22044604925031E-16,0.)) ;
#68980=DIRECTION('',(0.,0.,-1.)) ;
#68981=DIRECTION('center_axis',(1.,2.22044604925031E-16,0.)) ;
#68982=DIRECTION('ref_axis',(9.99672442260732E-31,-4.50212443845799E-15,
-1.)) ;
#68983=DIRECTION('',(1.,2.22044604925031E-16,0.)) ;
#68984=DIRECTION('center_axis',(-1.,-2.22044604925031E-16,0.)) ;
#68985=DIRECTION('ref_axis',(0.,0.,-1.)) ;
#68986=DIRECTION('center_axis',(2.22044604925031E-16,-1.,0.)) ;
#68987=DIRECTION('ref_axis',(0.,0.,-1.)) ;
#68988=DIRECTION('',(1.,2.22044604925031E-16,0.)) ;
#68989=DIRECTION('',(0.,0.,1.)) ;
#68990=DIRECTION('center_axis',(1.,2.22044604925031E-16,0.)) ;
#68991=DIRECTION('ref_axis',(2.22044604925031E-16,-1.,0.)) ;
#68992=DIRECTION('',(-1.,-2.22044604925031E-16,0.)) ;
#68993=DIRECTION('center_axis',(-1.,-2.22044604925031E-16,0.)) ;
#68994=DIRECTION('ref_axis',(3.47354289865164E-17,-0.15643446504023,-0.987688340595138)) ;
#68995=DIRECTION('center_axis',(-2.11176968422134E-16,0.951056516295154,
-0.309016994374947)) ;
#68996=DIRECTION('ref_axis',(-6.86155564311058E-17,0.309016994374947,0.951056516295154)) ;
#68997=DIRECTION('',(1.,2.22044604925031E-16,0.)) ;
#68998=DIRECTION('',(6.86155564311058E-17,-0.309016994374947,-0.951056516295154)) ;
#68999=DIRECTION('center_axis',(1.,2.22044604925031E-16,0.)) ;
#69000=DIRECTION('ref_axis',(6.86155564311052E-17,-0.309016994374945,-0.951056516295154)) ;
#69001=DIRECTION('',(1.,2.22044604925031E-16,0.)) ;
#69002=DIRECTION('center_axis',(-1.,-2.22044604925031E-16,0.)) ;
#69003=DIRECTION('ref_axis',(6.86155564311052E-17,-0.309016994374945,-0.951056516295154)) ;
#69004=DIRECTION('center_axis',(2.11176968422134E-16,-0.951056516295154,
0.309016994374947)) ;
#69005=DIRECTION('ref_axis',(6.86155564311058E-17,-0.309016994374947,-0.951056516295154)) ;
#69006=DIRECTION('',(1.,2.22044604925031E-16,0.)) ;
#69007=DIRECTION('',(-6.86155564311058E-17,0.309016994374947,0.951056516295154)) ;
#69008=DIRECTION('center_axis',(1.,2.22044604925031E-16,0.)) ;
#69009=DIRECTION('ref_axis',(2.22044604925031E-16,-1.,0.)) ;
#69010=DIRECTION('',(-1.,-2.22044604925031E-16,0.)) ;
#69011=DIRECTION('center_axis',(-1.,-2.22044604925031E-16,0.)) ;
#69012=DIRECTION('ref_axis',(1.00806141154385E-16,-0.453990499739546,-0.891006524188368)) ;
#69013=DIRECTION('center_axis',(-1.79637858893621E-16,0.809016994374948,
-0.587785252292473)) ;
#69014=DIRECTION('ref_axis',(-1.30514544126042E-16,0.587785252292473,0.809016994374948)) ;
#69015=DIRECTION('',(1.,2.22044604925031E-16,0.)) ;
#69016=DIRECTION('',(1.30514544126042E-16,-0.587785252292473,-0.809016994374947)) ;
#69017=DIRECTION('center_axis',(1.,2.22044604925031E-16,0.)) ;
#69018=DIRECTION('ref_axis',(1.30514544126041E-16,-0.587785252292468,-0.809016994374951)) ;
#69019=DIRECTION('',(1.,2.22044604925031E-16,0.)) ;
#69020=DIRECTION('center_axis',(-1.,-2.22044604925031E-16,0.)) ;
#69021=DIRECTION('ref_axis',(1.30514544126042E-16,-0.587785252292474,-0.809016994374947)) ;
#69022=DIRECTION('center_axis',(1.79637858893621E-16,-0.809016994374948,
0.587785252292473)) ;
#69023=DIRECTION('ref_axis',(1.30514544126042E-16,-0.587785252292473,-0.809016994374948)) ;
#69024=DIRECTION('',(1.,2.22044604925031E-16,0.)) ;
#69025=DIRECTION('',(-1.30514544126042E-16,0.587785252292473,0.809016994374947)) ;
#69026=DIRECTION('center_axis',(1.,2.22044604925031E-16,0.)) ;
#69027=DIRECTION('ref_axis',(2.22044604925031E-16,-1.,0.)) ;
#69028=DIRECTION('',(-1.,-2.22044604925031E-16,0.)) ;
#69029=DIRECTION('center_axis',(-1.,-2.22044604925031E-16,0.)) ;
#69030=DIRECTION('ref_axis',(1.57009245868377E-16,-0.707106781186547,-0.707106781186548)) ;
#69031=DIRECTION('center_axis',(-1.30514544126042E-16,0.587785252292473,
-0.809016994374947)) ;
#69032=DIRECTION('ref_axis',(-1.79637858893621E-16,0.809016994374947,0.587785252292473)) ;
#69033=DIRECTION('',(1.,2.22044604925031E-16,0.)) ;
#69034=DIRECTION('',(1.79637858893621E-16,-0.809016994374947,-0.587785252292473)) ;
#69035=DIRECTION('center_axis',(1.,2.22044604925031E-16,0.)) ;
#69036=DIRECTION('ref_axis',(1.79637858893621E-16,-0.809016994374949,-0.587785252292472)) ;
#69037=DIRECTION('',(1.,2.22044604925031E-16,0.)) ;
#69038=DIRECTION('center_axis',(-1.,-2.22044604925031E-16,0.)) ;
#69039=DIRECTION('ref_axis',(1.79637858893621E-16,-0.809016994374947,-0.587785252292474)) ;
#69040=DIRECTION('center_axis',(1.30514544126042E-16,-0.587785252292473,
0.809016994374947)) ;
#69041=DIRECTION('ref_axis',(1.79637858893621E-16,-0.809016994374947,-0.587785252292473)) ;
#69042=DIRECTION('',(1.,2.22044604925031E-16,0.)) ;
#69043=DIRECTION('',(-1.79637858893621E-16,0.809016994374947,0.587785252292473)) ;
#69044=DIRECTION('center_axis',(1.,2.22044604925031E-16,0.)) ;
#69045=DIRECTION('ref_axis',(2.22044604925031E-16,-1.,0.)) ;
#69046=DIRECTION('',(-1.,-2.22044604925031E-16,0.)) ;
#69047=DIRECTION('center_axis',(-1.,-2.22044604925031E-16,0.)) ;
#69048=DIRECTION('ref_axis',(1.97843191649031E-16,-0.891006524188368,-0.453990499739547)) ;
#69049=DIRECTION('center_axis',(-6.86155564311058E-17,0.309016994374948,
-0.951056516295154)) ;
#69050=DIRECTION('ref_axis',(-2.11176968422134E-16,0.951056516295154,0.309016994374948)) ;
#69051=DIRECTION('',(1.,2.22044604925031E-16,0.)) ;
#69052=DIRECTION('',(2.11176968422134E-16,-0.951056516295154,-0.309016994374948)) ;
#69053=DIRECTION('center_axis',(1.,2.22044604925031E-16,0.)) ;
#69054=DIRECTION('ref_axis',(2.11176968422134E-16,-0.951056516295157,-0.309016994374937)) ;
#69055=DIRECTION('',(1.,2.22044604925031E-16,0.)) ;
#69056=DIRECTION('center_axis',(-1.,-2.22044604925031E-16,0.)) ;
#69057=DIRECTION('ref_axis',(2.11176968422134E-16,-0.951056516295154,-0.309016994374945)) ;
#69058=DIRECTION('center_axis',(6.86155564311058E-17,-0.309016994374948,
0.951056516295154)) ;
#69059=DIRECTION('ref_axis',(2.11176968422134E-16,-0.951056516295154,-0.309016994374948)) ;
#69060=DIRECTION('',(1.,2.22044604925031E-16,0.)) ;
#69061=DIRECTION('',(-2.11176968422134E-16,0.951056516295154,0.309016994374948)) ;
#69062=DIRECTION('center_axis',(1.,2.22044604925031E-16,0.)) ;
#69063=DIRECTION('ref_axis',(2.22044604925031E-16,-1.,0.)) ;
#69064=DIRECTION('',(-1.,-2.22044604925031E-16,0.)) ;
#69065=DIRECTION('center_axis',(-1.,-2.22044604925031E-16,0.)) ;
#69066=DIRECTION('ref_axis',(2.19310867376507E-16,-0.987688340595138,-0.156434465040231)) ;
#69067=DIRECTION('center_axis',(-1.23259516440783E-32,5.55111512312578E-17,
-1.)) ;
#69068=DIRECTION('ref_axis',(-2.22044604925031E-16,1.,5.55111512312578E-17)) ;
#69069=DIRECTION('',(1.,2.22044604925031E-16,0.)) ;
#69070=DIRECTION('',(2.22044604925031E-16,-1.,-5.55111512312578E-17)) ;
#69071=DIRECTION('center_axis',(1.,2.22044604925031E-16,0.)) ;
#69072=DIRECTION('ref_axis',(2.22044604925031E-16,-1.,6.5797721569339E-16)) ;
#69073=DIRECTION('',(1.,2.22044604925031E-16,0.)) ;
#69074=DIRECTION('center_axis',(-1.,-2.22044604925031E-16,0.)) ;
#69075=DIRECTION('ref_axis',(2.22044604925031E-16,-1.,0.)) ;
#69076=DIRECTION('center_axis',(1.23259516440783E-32,-5.55111512312578E-17,
1.)) ;
#69077=DIRECTION('ref_axis',(2.22044604925031E-16,-1.,-5.55111512312578E-17)) ;
#69078=DIRECTION('',(1.,2.22044604925031E-16,0.)) ;
#69079=DIRECTION('',(-2.22044604925031E-16,1.,5.55111512312578E-17)) ;
#69080=DIRECTION('center_axis',(1.,2.22044604925031E-16,0.)) ;
#69081=DIRECTION('ref_axis',(2.22044604925031E-16,-1.,0.)) ;
#69082=DIRECTION('',(-1.,-2.22044604925031E-16,0.)) ;
#69083=DIRECTION('center_axis',(-1.,-2.22044604925031E-16,0.)) ;
#69084=DIRECTION('ref_axis',(2.19310867376507E-16,-0.987688340595138,0.156434465040229)) ;
#69085=DIRECTION('center_axis',(6.86155564311058E-17,-0.309016994374947,
-0.951056516295154)) ;
#69086=DIRECTION('ref_axis',(-2.11176968422134E-16,0.951056516295154,-0.309016994374947)) ;
#69087=DIRECTION('',(1.,2.22044604925031E-16,0.)) ;
#69088=DIRECTION('',(2.11176968422134E-16,-0.951056516295154,0.309016994374947)) ;
#69089=DIRECTION('center_axis',(1.,2.22044604925031E-16,0.)) ;
#69090=DIRECTION('ref_axis',(2.11176968422134E-16,-0.951056516295156,0.309016994374939)) ;
#69091=DIRECTION('',(1.,2.22044604925031E-16,0.)) ;
#69092=DIRECTION('center_axis',(-1.,-2.22044604925031E-16,0.)) ;
#69093=DIRECTION('ref_axis',(2.11176968422134E-16,-0.951056516295154,0.309016994374945)) ;
#69094=DIRECTION('center_axis',(-6.86155564311058E-17,0.309016994374947,
0.951056516295154)) ;
#69095=DIRECTION('ref_axis',(2.11176968422134E-16,-0.951056516295154,0.309016994374947)) ;
#69096=DIRECTION('',(1.,2.22044604925031E-16,0.)) ;
#69097=DIRECTION('',(-2.11176968422134E-16,0.951056516295154,-0.309016994374947)) ;
#69098=DIRECTION('center_axis',(1.,2.22044604925031E-16,0.)) ;
#69099=DIRECTION('ref_axis',(2.22044604925031E-16,-1.,0.)) ;
#69100=DIRECTION('',(-1.,-2.22044604925031E-16,0.)) ;
#69101=DIRECTION('center_axis',(-1.,-2.22044604925031E-16,0.)) ;
#69102=DIRECTION('ref_axis',(1.97843191649031E-16,-0.891006524188369,0.453990499739545)) ;
#69103=DIRECTION('center_axis',(1.30514544126042E-16,-0.587785252292473,
-0.809016994374948)) ;
#69104=DIRECTION('ref_axis',(-1.79637858893621E-16,0.809016994374948,-0.587785252292473)) ;
#69105=DIRECTION('',(1.,2.22044604925031E-16,0.)) ;
#69106=DIRECTION('',(1.79637858893621E-16,-0.809016994374947,0.587785252292473)) ;
#69107=DIRECTION('center_axis',(1.,2.22044604925031E-16,0.)) ;
#69108=DIRECTION('ref_axis',(1.79637858893618E-16,-0.809016994374932,0.587785252292495)) ;
#69109=DIRECTION('',(1.,2.22044604925031E-16,0.)) ;
#69110=DIRECTION('center_axis',(-1.,-2.22044604925031E-16,0.)) ;
#69111=DIRECTION('ref_axis',(1.79637858893621E-16,-0.809016994374947,0.587785252292474)) ;
#69112=DIRECTION('center_axis',(-1.30514544126042E-16,0.587785252292473,
0.809016994374948)) ;
#69113=DIRECTION('ref_axis',(1.79637858893621E-16,-0.809016994374948,0.587785252292473)) ;
#69114=DIRECTION('',(1.,2.22044604925031E-16,0.)) ;
#69115=DIRECTION('',(-1.79637858893621E-16,0.809016994374947,-0.587785252292473)) ;
#69116=DIRECTION('center_axis',(1.,2.22044604925031E-16,0.)) ;
#69117=DIRECTION('ref_axis',(2.22044604925031E-16,-1.,0.)) ;
#69118=DIRECTION('',(-1.,-2.22044604925031E-16,0.)) ;
#69119=DIRECTION('center_axis',(-1.,-2.22044604925031E-16,0.)) ;
#69120=DIRECTION('ref_axis',(1.57009245868377E-16,-0.707106781186548,0.707106781186547)) ;
#69121=DIRECTION('center_axis',(1.79637858893621E-16,-0.809016994374947,
-0.587785252292473)) ;
#69122=DIRECTION('ref_axis',(-1.30514544126042E-16,0.587785252292473,-0.809016994374947)) ;
#69123=DIRECTION('',(1.,2.22044604925031E-16,0.)) ;
#69124=DIRECTION('',(1.30514544126042E-16,-0.587785252292473,0.809016994374947)) ;
#69125=DIRECTION('center_axis',(1.,2.22044604925031E-16,0.)) ;
#69126=DIRECTION('ref_axis',(1.30514544126042E-16,-0.587785252292474,0.809016994374947)) ;
#69127=DIRECTION('',(1.,2.22044604925031E-16,0.)) ;
#69128=DIRECTION('center_axis',(-1.,-2.22044604925031E-16,0.)) ;
#69129=DIRECTION('ref_axis',(1.30514544126042E-16,-0.587785252292474,0.809016994374947)) ;
#69130=DIRECTION('center_axis',(-1.79637858893621E-16,0.809016994374947,
0.587785252292473)) ;
#69131=DIRECTION('ref_axis',(1.30514544126042E-16,-0.587785252292473,0.809016994374947)) ;
#69132=DIRECTION('',(1.,2.22044604925031E-16,0.)) ;
#69133=DIRECTION('',(-1.30514544126042E-16,0.587785252292473,-0.809016994374947)) ;
#69134=DIRECTION('center_axis',(1.,2.22044604925031E-16,0.)) ;
#69135=DIRECTION('ref_axis',(2.22044604925031E-16,-1.,0.)) ;
#69136=DIRECTION('',(-1.,-2.22044604925031E-16,0.)) ;
#69137=DIRECTION('center_axis',(-1.,-2.22044604925031E-16,0.)) ;
#69138=DIRECTION('ref_axis',(1.00806141154385E-16,-0.453990499739546,0.891006524188368)) ;
#69139=DIRECTION('center_axis',(-1.,-2.22044604925031E-16,0.)) ;
#69140=DIRECTION('ref_axis',(2.22044604925031E-16,-1.,0.)) ;
#69141=DIRECTION('center_axis',(1.,2.22044604925031E-16,0.)) ;
#69142=DIRECTION('ref_axis',(9.02179155423715E-17,-0.406305370818768,0.913737350469939)) ;
#69143=DIRECTION('center_axis',(-1.,-2.22044604925031E-16,0.)) ;
#69144=DIRECTION('ref_axis',(2.22044604925031E-16,-1.,0.)) ;
#69145=DIRECTION('center_axis',(1.,2.22044604925031E-16,0.)) ;
#69146=DIRECTION('ref_axis',(9.02179155423715E-17,-0.406305370818768,0.913737350469939)) ;
#69147=DIRECTION('center_axis',(-1.,-2.22044604925031E-16,0.)) ;
#69148=DIRECTION('ref_axis',(2.22044604925031E-16,-1.,0.)) ;
#69149=DIRECTION('center_axis',(1.,2.22044604925031E-16,0.)) ;
#69150=DIRECTION('ref_axis',(9.02179155423715E-17,-0.406305370818768,0.913737350469939)) ;
#69151=DIRECTION('center_axis',(-1.,-2.22044604925031E-16,0.)) ;
#69152=DIRECTION('ref_axis',(2.22044604925031E-16,-1.,0.)) ;
#69153=DIRECTION('center_axis',(1.,2.22044604925031E-16,0.)) ;
#69154=DIRECTION('ref_axis',(9.02179155423715E-17,-0.406305370818768,0.913737350469939)) ;
#69155=DIRECTION('center_axis',(-1.,-2.22044604925031E-16,0.)) ;
#69156=DIRECTION('ref_axis',(2.22044604925031E-16,-1.,0.)) ;
#69157=DIRECTION('center_axis',(1.,2.22044604925031E-16,0.)) ;
#69158=DIRECTION('ref_axis',(9.02179155423715E-17,-0.406305370818768,0.913737350469939)) ;
#69159=DIRECTION('center_axis',(-1.,-2.22044604925031E-16,0.)) ;
#69160=DIRECTION('ref_axis',(2.22044604925031E-16,-1.,0.)) ;
#69161=DIRECTION('center_axis',(1.,2.22044604925031E-16,0.)) ;
#69162=DIRECTION('ref_axis',(9.02179155423715E-17,-0.406305370818768,0.913737350469939)) ;
#69163=DIRECTION('center_axis',(-1.,-2.22044604925031E-16,0.)) ;
#69164=DIRECTION('ref_axis',(2.22044604925031E-16,-1.,0.)) ;
#69165=DIRECTION('center_axis',(1.,2.22044604925031E-16,0.)) ;
#69166=DIRECTION('ref_axis',(9.02179155423715E-17,-0.406305370818768,0.913737350469939)) ;
#69167=DIRECTION('center_axis',(-1.,-2.22044604925031E-16,0.)) ;
#69168=DIRECTION('ref_axis',(2.22044604925031E-16,-1.,0.)) ;
#69169=DIRECTION('center_axis',(1.,2.22044604925031E-16,0.)) ;
#69170=DIRECTION('ref_axis',(9.02179155423715E-17,-0.406305370818768,0.913737350469939)) ;
#69171=DIRECTION('center_axis',(-1.,-2.22044604925031E-16,0.)) ;
#69172=DIRECTION('ref_axis',(2.22044604925031E-16,-1.,0.)) ;
#69173=DIRECTION('center_axis',(1.,2.22044604925031E-16,0.)) ;
#69174=DIRECTION('ref_axis',(9.02179155423715E-17,-0.406305370818768,0.913737350469939)) ;
#69175=DIRECTION('center_axis',(-1.,-2.22044604925031E-16,0.)) ;
#69176=DIRECTION('ref_axis',(2.22044604925031E-16,-1.,0.)) ;
#69177=DIRECTION('center_axis',(1.,2.22044604925031E-16,0.)) ;
#69178=DIRECTION('ref_axis',(9.02179155423715E-17,-0.406305370818768,0.913737350469939)) ;
#69179=DIRECTION('center_axis',(-1.,-2.22044604925031E-16,0.)) ;
#69180=DIRECTION('ref_axis',(2.22044604925031E-16,-1.,0.)) ;
#69181=DIRECTION('center_axis',(1.,2.22044604925031E-16,0.)) ;
#69182=DIRECTION('ref_axis',(9.02179155423715E-17,-0.406305370818768,0.913737350469939)) ;
#69183=DIRECTION('center_axis',(-1.,-2.22044604925031E-16,0.)) ;
#69184=DIRECTION('ref_axis',(2.22044604925031E-16,-1.,0.)) ;
#69185=DIRECTION('center_axis',(1.,2.22044604925031E-16,0.)) ;
#69186=DIRECTION('ref_axis',(9.02179155423715E-17,-0.406305370818768,0.913737350469939)) ;
#69187=DIRECTION('center_axis',(-1.,-2.22044604925031E-16,0.)) ;
#69188=DIRECTION('ref_axis',(2.22044604925031E-16,-1.,0.)) ;
#69189=DIRECTION('center_axis',(1.,2.22044604925031E-16,0.)) ;
#69190=DIRECTION('ref_axis',(9.02179155423715E-17,-0.406305370818768,0.913737350469939)) ;
#69191=DIRECTION('center_axis',(-1.,-2.22044604925031E-16,0.)) ;
#69192=DIRECTION('ref_axis',(2.22044604925031E-16,-1.,0.)) ;
#69193=DIRECTION('center_axis',(1.,2.22044604925031E-16,0.)) ;
#69194=DIRECTION('ref_axis',(9.02179155423715E-17,-0.406305370818768,0.913737350469939)) ;
#69195=DIRECTION('center_axis',(-1.,-2.22044604925031E-16,0.)) ;
#69196=DIRECTION('ref_axis',(2.22044604925031E-16,-1.,0.)) ;
#69197=DIRECTION('center_axis',(1.,2.22044604925031E-16,0.)) ;
#69198=DIRECTION('ref_axis',(9.02179155423715E-17,-0.406305370818768,0.913737350469939)) ;
#69199=DIRECTION('center_axis',(-1.,-2.22044604925031E-16,0.)) ;
#69200=DIRECTION('ref_axis',(2.22044604925031E-16,-1.,0.)) ;
#69201=DIRECTION('center_axis',(1.,2.22044604925031E-16,0.)) ;
#69202=DIRECTION('ref_axis',(9.02179155423715E-17,-0.406305370818768,0.913737350469939)) ;
#69203=DIRECTION('center_axis',(-1.,-2.22044604925031E-16,0.)) ;
#69204=DIRECTION('ref_axis',(2.22044604925031E-16,-1.,0.)) ;
#69205=DIRECTION('center_axis',(1.,2.22044604925031E-16,0.)) ;
#69206=DIRECTION('ref_axis',(9.02179155423715E-17,-0.406305370818768,0.913737350469939)) ;
#69207=DIRECTION('center_axis',(-1.,-2.22044604925031E-16,0.)) ;
#69208=DIRECTION('ref_axis',(2.22044604925031E-16,-1.,0.)) ;
#69209=DIRECTION('center_axis',(1.,2.22044604925031E-16,0.)) ;
#69210=DIRECTION('ref_axis',(9.02179155423715E-17,-0.406305370818768,0.913737350469939)) ;
#69211=DIRECTION('center_axis',(-1.,-2.22044604925031E-16,0.)) ;
#69212=DIRECTION('ref_axis',(2.22044604925031E-16,-1.,0.)) ;
#69213=DIRECTION('center_axis',(1.,2.22044604925031E-16,0.)) ;
#69214=DIRECTION('ref_axis',(9.02179155423715E-17,-0.406305370818768,0.913737350469939)) ;
#69215=DIRECTION('center_axis',(1.,2.22044604925031E-16,0.)) ;
#69216=DIRECTION('ref_axis',(9.02179155423715E-17,-0.406305370818768,0.913737350469939)) ;
#69217=DIRECTION('center_axis',(1.,2.22044604925031E-16,0.)) ;
#69218=DIRECTION('ref_axis',(0.,0.,-1.)) ;
#69219=DIRECTION('center_axis',(-2.22044604925031E-16,1.,0.)) ;
#69220=DIRECTION('ref_axis',(0.,0.,1.)) ;
#69221=DIRECTION('center_axis',(1.,2.22044604925031E-16,0.)) ;
#69222=DIRECTION('ref_axis',(9.02179155423715E-17,-0.406305370818768,0.913737350469939)) ;
#69223=DIRECTION('center_axis',(-1.,-2.22044604925031E-16,0.)) ;
#69224=DIRECTION('ref_axis',(2.22044604925031E-16,-1.,0.)) ;
#69225=DIRECTION('center_axis',(-1.,-2.22044604925031E-16,0.)) ;
#69226=DIRECTION('ref_axis',(0.,0.,1.)) ;
#69227=DIRECTION('center_axis',(-2.22044604925031E-16,1.,0.)) ;
#69228=DIRECTION('ref_axis',(0.,0.,-1.)) ;
#69229=DIRECTION('center_axis',(-1.,-2.22044604925031E-16,0.)) ;
#69230=DIRECTION('ref_axis',(4.62681868766601E-17,-0.208373389176835,0.978049349819813)) ;
#69231=DIRECTION('center_axis',(1.,2.22044604925031E-16,0.)) ;
#69232=DIRECTION('ref_axis',(3.47354289865164E-17,-0.15643446504023,-0.987688340595138)) ;
#69233=DIRECTION('center_axis',(-1.,-2.22044604925031E-16,0.)) ;
#69234=DIRECTION('ref_axis',(4.62681868766601E-17,-0.208373389176835,0.978049349819813)) ;
#69235=DIRECTION('center_axis',(1.,2.22044604925031E-16,0.)) ;
#69236=DIRECTION('ref_axis',(1.00806141154385E-16,-0.453990499739546,-0.891006524188368)) ;
#69237=DIRECTION('center_axis',(-1.,-2.22044604925031E-16,0.)) ;
#69238=DIRECTION('ref_axis',(4.62681868766601E-17,-0.208373389176835,0.978049349819813)) ;
#69239=DIRECTION('center_axis',(1.,2.22044604925031E-16,0.)) ;
#69240=DIRECTION('ref_axis',(1.57009245868377E-16,-0.707106781186547,-0.707106781186548)) ;
#69241=DIRECTION('center_axis',(-1.,-2.22044604925031E-16,0.)) ;
#69242=DIRECTION('ref_axis',(4.62681868766601E-17,-0.208373389176835,0.978049349819813)) ;
#69243=DIRECTION('center_axis',(1.,2.22044604925031E-16,0.)) ;
#69244=DIRECTION('ref_axis',(1.97843191649031E-16,-0.891006524188368,-0.453990499739547)) ;
#69245=DIRECTION('center_axis',(-1.,-2.22044604925031E-16,0.)) ;
#69246=DIRECTION('ref_axis',(4.62681868766601E-17,-0.208373389176835,0.978049349819813)) ;
#69247=DIRECTION('center_axis',(1.,2.22044604925031E-16,0.)) ;
#69248=DIRECTION('ref_axis',(2.19310867376507E-16,-0.987688340595138,-0.156434465040231)) ;
#69249=DIRECTION('center_axis',(-1.,-2.22044604925031E-16,0.)) ;
#69250=DIRECTION('ref_axis',(4.62681868766601E-17,-0.208373389176835,0.978049349819813)) ;
#69251=DIRECTION('center_axis',(1.,2.22044604925031E-16,0.)) ;
#69252=DIRECTION('ref_axis',(2.19310867376507E-16,-0.987688340595138,0.156434465040229)) ;
#69253=DIRECTION('center_axis',(-1.,-2.22044604925031E-16,0.)) ;
#69254=DIRECTION('ref_axis',(4.62681868766601E-17,-0.208373389176835,0.978049349819813)) ;
#69255=DIRECTION('center_axis',(1.,2.22044604925031E-16,0.)) ;
#69256=DIRECTION('ref_axis',(1.97843191649031E-16,-0.891006524188369,0.453990499739545)) ;
#69257=DIRECTION('center_axis',(-1.,-2.22044604925031E-16,0.)) ;
#69258=DIRECTION('ref_axis',(4.62681868766601E-17,-0.208373389176835,0.978049349819813)) ;
#69259=DIRECTION('center_axis',(1.,2.22044604925031E-16,0.)) ;
#69260=DIRECTION('ref_axis',(1.57009245868377E-16,-0.707106781186548,0.707106781186547)) ;
#69261=DIRECTION('center_axis',(-1.,-2.22044604925031E-16,0.)) ;
#69262=DIRECTION('ref_axis',(4.62681868766601E-17,-0.208373389176835,0.978049349819813)) ;
#69263=DIRECTION('center_axis',(1.,2.22044604925031E-16,0.)) ;
#69264=DIRECTION('ref_axis',(1.00806141154385E-16,-0.453990499739546,0.891006524188368)) ;
#69265=DIRECTION('center_axis',(-1.,-2.22044604925031E-16,0.)) ;
#69266=DIRECTION('ref_axis',(4.62681868766601E-17,-0.208373389176835,0.978049349819813)) ;
#69267=DIRECTION('center_axis',(1.,2.22044604925031E-16,0.)) ;
#69268=DIRECTION('ref_axis',(3.47354289865169E-17,-0.156434465040232,0.987688340595138)) ;
#69269=DIRECTION('center_axis',(-1.,-2.22044604925031E-16,0.)) ;
#69270=DIRECTION('ref_axis',(4.62681868766601E-17,-0.208373389176835,0.978049349819813)) ;
#69271=DIRECTION('center_axis',(1.,2.22044604925031E-16,0.)) ;
#69272=DIRECTION('ref_axis',(-3.47354289865171E-17,0.156434465040233,0.987688340595137)) ;
#69273=DIRECTION('center_axis',(-1.,-2.22044604925031E-16,0.)) ;
#69274=DIRECTION('ref_axis',(4.62681868766601E-17,-0.208373389176835,0.978049349819813)) ;
#69275=DIRECTION('center_axis',(1.,2.22044604925031E-16,0.)) ;
#69276=DIRECTION('ref_axis',(-1.00806141154386E-16,0.453990499739549,0.891006524188367)) ;
#69277=DIRECTION('center_axis',(-1.,-2.22044604925031E-16,0.)) ;
#69278=DIRECTION('ref_axis',(4.62681868766601E-17,-0.208373389176835,0.978049349819813)) ;
#69279=DIRECTION('center_axis',(1.,2.22044604925031E-16,0.)) ;
#69280=DIRECTION('ref_axis',(-1.57009245868377E-16,0.707106781186548,0.707106781186547)) ;
#69281=DIRECTION('center_axis',(-1.,-2.22044604925031E-16,0.)) ;
#69282=DIRECTION('ref_axis',(4.62681868766601E-17,-0.208373389176835,0.978049349819813)) ;
#69283=DIRECTION('center_axis',(1.,2.22044604925031E-16,0.)) ;
#69284=DIRECTION('ref_axis',(-1.97843191649031E-16,0.891006524188368,0.453990499739546)) ;
#69285=DIRECTION('center_axis',(-1.,-2.22044604925031E-16,0.)) ;
#69286=DIRECTION('ref_axis',(4.62681868766601E-17,-0.208373389176835,0.978049349819813)) ;
#69287=DIRECTION('center_axis',(1.,2.22044604925031E-16,0.)) ;
#69288=DIRECTION('ref_axis',(-2.19310867376507E-16,0.987688340595138,0.156434465040232)) ;
#69289=DIRECTION('center_axis',(-1.,-2.22044604925031E-16,0.)) ;
#69290=DIRECTION('ref_axis',(4.62681868766601E-17,-0.208373389176835,0.978049349819813)) ;
#69291=DIRECTION('center_axis',(1.,2.22044604925031E-16,0.)) ;
#69292=DIRECTION('ref_axis',(-2.19310867376507E-16,0.987688340595138,-0.156434465040228)) ;
#69293=DIRECTION('center_axis',(-1.,-2.22044604925031E-16,0.)) ;
#69294=DIRECTION('ref_axis',(4.62681868766601E-17,-0.208373389176835,0.978049349819813)) ;
#69295=DIRECTION('center_axis',(1.,2.22044604925031E-16,0.)) ;
#69296=DIRECTION('ref_axis',(-1.97843191649031E-16,0.891006524188368,-0.453990499739547)) ;
#69297=DIRECTION('center_axis',(-1.,-2.22044604925031E-16,0.)) ;
#69298=DIRECTION('ref_axis',(4.62681868766601E-17,-0.208373389176835,0.978049349819813)) ;
#69299=DIRECTION('center_axis',(1.,2.22044604925031E-16,0.)) ;
#69300=DIRECTION('ref_axis',(-1.57009245868377E-16,0.707106781186547,-0.707106781186547)) ;
#69301=DIRECTION('center_axis',(-1.,-2.22044604925031E-16,0.)) ;
#69302=DIRECTION('ref_axis',(4.62681868766601E-17,-0.208373389176835,0.978049349819813)) ;
#69303=DIRECTION('center_axis',(1.,2.22044604925031E-16,0.)) ;
#69304=DIRECTION('ref_axis',(-1.00806141154385E-16,0.453990499739547,-0.891006524188368)) ;
#69305=DIRECTION('center_axis',(-1.,-2.22044604925031E-16,0.)) ;
#69306=DIRECTION('ref_axis',(4.62681868766601E-17,-0.208373389176835,0.978049349819813)) ;
#69307=DIRECTION('center_axis',(1.,2.22044604925031E-16,0.)) ;
#69308=DIRECTION('ref_axis',(-3.47354289865169E-17,0.156434465040232,-0.987688340595138)) ;
#69309=DIRECTION('center_axis',(-1.,-2.22044604925031E-16,0.)) ;
#69310=DIRECTION('ref_axis',(4.62681868766601E-17,-0.208373389176835,0.978049349819813)) ;
#69311=DIRECTION('center_axis',(-1.,-2.22044604925031E-16,0.)) ;
#69312=DIRECTION('ref_axis',(2.22044604925031E-16,-1.,0.)) ;
#69313=DIRECTION('',(6.86155564311059E-17,-0.309016994374948,0.951056516295153)) ;
#69314=DIRECTION('center_axis',(1.,2.22044604925031E-16,0.)) ;
#69315=DIRECTION('ref_axis',(-6.86155564311052E-17,0.309016994374945,-0.951056516295154)) ;
#69316=DIRECTION('',(-6.86155564311059E-17,0.309016994374948,-0.951056516295153)) ;
#69317=DIRECTION('center_axis',(-1.,-2.22044604925031E-16,0.)) ;
#69318=DIRECTION('ref_axis',(2.22044604925031E-16,-1.,0.)) ;
#69319=DIRECTION('',(1.30514544126042E-16,-0.587785252292473,0.809016994374947)) ;
#69320=DIRECTION('center_axis',(1.,2.22044604925031E-16,0.)) ;
#69321=DIRECTION('ref_axis',(-1.30514544126041E-16,0.587785252292468,-0.809016994374951)) ;
#69322=DIRECTION('',(-1.30514544126042E-16,0.587785252292473,-0.809016994374947)) ;
#69323=DIRECTION('center_axis',(-1.,-2.22044604925031E-16,0.)) ;
#69324=DIRECTION('ref_axis',(2.22044604925031E-16,-1.,0.)) ;
#69325=DIRECTION('',(1.79637858893621E-16,-0.809016994374948,0.587785252292473)) ;
#69326=DIRECTION('center_axis',(1.,2.22044604925031E-16,0.)) ;
#69327=DIRECTION('ref_axis',(-1.79637858893621E-16,0.809016994374947,-0.587785252292474)) ;
#69328=DIRECTION('',(-1.79637858893621E-16,0.809016994374948,-0.587785252292473)) ;
#69329=DIRECTION('center_axis',(-1.,-2.22044604925031E-16,0.)) ;
#69330=DIRECTION('ref_axis',(2.22044604925031E-16,-1.,0.)) ;
#69331=DIRECTION('',(2.11176968422134E-16,-0.951056516295154,0.309016994374947)) ;
#69332=DIRECTION('center_axis',(1.,2.22044604925031E-16,0.)) ;
#69333=DIRECTION('ref_axis',(-2.11176968422134E-16,0.951056516295153,-0.309016994374948)) ;
#69334=DIRECTION('',(-2.11176968422134E-16,0.951056516295154,-0.309016994374947)) ;
#69335=DIRECTION('center_axis',(-1.,-2.22044604925031E-16,0.)) ;
#69336=DIRECTION('ref_axis',(2.22044604925031E-16,-1.,0.)) ;
#69337=DIRECTION('',(2.22044604925031E-16,-1.,-2.22044604925031E-16)) ;
#69338=DIRECTION('center_axis',(1.,2.22044604925031E-16,0.)) ;
#69339=DIRECTION('ref_axis',(-2.22044604925031E-16,1.,0.)) ;
#69340=DIRECTION('',(-2.22044604925031E-16,1.,2.22044604925031E-16)) ;
#69341=DIRECTION('center_axis',(-1.,-2.22044604925031E-16,0.)) ;
#69342=DIRECTION('ref_axis',(2.22044604925031E-16,-1.,0.)) ;
#69343=DIRECTION('',(2.11176968422134E-16,-0.951056516295153,-0.309016994374948)) ;
#69344=DIRECTION('center_axis',(1.,2.22044604925031E-16,0.)) ;
#69345=DIRECTION('ref_axis',(-2.11176968422134E-16,0.951056516295153,0.309016994374948)) ;
#69346=DIRECTION('',(-2.11176968422134E-16,0.951056516295153,0.309016994374948)) ;
#69347=DIRECTION('center_axis',(-1.,-2.22044604925031E-16,0.)) ;
#69348=DIRECTION('ref_axis',(2.22044604925031E-16,-1.,0.)) ;
#69349=DIRECTION('',(1.79637858893621E-16,-0.809016994374947,-0.587785252292473)) ;
#69350=DIRECTION('center_axis',(1.,2.22044604925031E-16,0.)) ;
#69351=DIRECTION('ref_axis',(-1.79637858893621E-16,0.809016994374947,0.587785252292474)) ;
#69352=DIRECTION('',(-1.79637858893621E-16,0.809016994374947,0.587785252292473)) ;
#69353=DIRECTION('center_axis',(-1.,-2.22044604925031E-16,0.)) ;
#69354=DIRECTION('ref_axis',(2.22044604925031E-16,-1.,0.)) ;
#69355=DIRECTION('',(1.30514544126042E-16,-0.587785252292473,-0.809016994374947)) ;
#69356=DIRECTION('center_axis',(1.,2.22044604925031E-16,0.)) ;
#69357=DIRECTION('ref_axis',(-1.30514544126041E-16,0.587785252292468,0.809016994374951)) ;
#69358=DIRECTION('',(-1.30514544126042E-16,0.587785252292473,0.809016994374947)) ;
#69359=DIRECTION('center_axis',(-1.,-2.22044604925031E-16,0.)) ;
#69360=DIRECTION('ref_axis',(2.22044604925031E-16,-1.,0.)) ;
#69361=DIRECTION('',(6.86155564311058E-17,-0.309016994374947,-0.951056516295154)) ;
#69362=DIRECTION('center_axis',(1.,2.22044604925031E-16,0.)) ;
#69363=DIRECTION('ref_axis',(-6.86155564311052E-17,0.309016994374945,0.951056516295154)) ;
#69364=DIRECTION('',(-6.86155564311058E-17,0.309016994374947,0.951056516295154)) ;
#69365=DIRECTION('center_axis',(-1.,-2.22044604925031E-16,0.)) ;
#69366=DIRECTION('ref_axis',(2.22044604925031E-16,-1.,0.)) ;
#69367=DIRECTION('',(-2.46519032881566E-32,1.11022302462516E-16,-1.)) ;
#69368=DIRECTION('center_axis',(1.,2.22044604925031E-16,0.)) ;
#69369=DIRECTION('ref_axis',(0.,0.,1.)) ;
#69370=DIRECTION('',(2.46519032881566E-32,-1.11022302462516E-16,1.)) ;
#69371=DIRECTION('center_axis',(-1.,-2.22044604925031E-16,0.)) ;
#69372=DIRECTION('ref_axis',(2.22044604925031E-16,-1.,0.)) ;
#69373=DIRECTION('',(-6.86155564311058E-17,0.309016994374948,-0.951056516295154)) ;
#69374=DIRECTION('center_axis',(1.,2.22044604925031E-16,0.)) ;
#69375=DIRECTION('ref_axis',(6.86155564311052E-17,-0.309016994374945,0.951056516295154)) ;
#69376=DIRECTION('',(6.86155564311058E-17,-0.309016994374948,0.951056516295154)) ;
#69377=DIRECTION('center_axis',(-1.,-2.22044604925031E-16,0.)) ;
#69378=DIRECTION('ref_axis',(2.22044604925031E-16,-1.,0.)) ;
#69379=DIRECTION('',(-1.30514544126042E-16,0.587785252292473,-0.809016994374947)) ;
#69380=DIRECTION('center_axis',(1.,2.22044604925031E-16,0.)) ;
#69381=DIRECTION('ref_axis',(1.30514544126042E-16,-0.587785252292474,0.809016994374947)) ;
#69382=DIRECTION('',(1.30514544126042E-16,-0.587785252292473,0.809016994374947)) ;
#69383=DIRECTION('center_axis',(-1.,-2.22044604925031E-16,0.)) ;
#69384=DIRECTION('ref_axis',(2.22044604925031E-16,-1.,0.)) ;
#69385=DIRECTION('',(-1.79637858893621E-16,0.809016994374947,-0.587785252292473)) ;
#69386=DIRECTION('center_axis',(1.,2.22044604925031E-16,0.)) ;
#69387=DIRECTION('ref_axis',(1.79637858893621E-16,-0.809016994374947,0.587785252292474)) ;
#69388=DIRECTION('',(1.79637858893621E-16,-0.809016994374947,0.587785252292473)) ;
#69389=DIRECTION('center_axis',(-1.,-2.22044604925031E-16,0.)) ;
#69390=DIRECTION('ref_axis',(2.22044604925031E-16,-1.,0.)) ;
#69391=DIRECTION('',(-2.11176968422134E-16,0.951056516295154,-0.309016994374947)) ;
#69392=DIRECTION('center_axis',(1.,2.22044604925031E-16,0.)) ;
#69393=DIRECTION('ref_axis',(2.11176968422134E-16,-0.951056516295154,0.309016994374945)) ;
#69394=DIRECTION('',(2.11176968422134E-16,-0.951056516295154,0.309016994374947)) ;
#69395=DIRECTION('center_axis',(-1.,-2.22044604925031E-16,0.)) ;
#69396=DIRECTION('ref_axis',(2.22044604925031E-16,-1.,0.)) ;
#69397=DIRECTION('',(-2.22044604925031E-16,1.,5.55111512312578E-17)) ;
#69398=DIRECTION('center_axis',(1.,2.22044604925031E-16,0.)) ;
#69399=DIRECTION('ref_axis',(2.22044604925031E-16,-1.,0.)) ;
#69400=DIRECTION('',(2.22044604925031E-16,-1.,-5.55111512312578E-17)) ;
#69401=DIRECTION('center_axis',(-1.,-2.22044604925031E-16,0.)) ;
#69402=DIRECTION('ref_axis',(2.22044604925031E-16,-1.,0.)) ;
#69403=DIRECTION('',(-2.11176968422134E-16,0.951056516295154,0.309016994374948)) ;
#69404=DIRECTION('center_axis',(1.,2.22044604925031E-16,0.)) ;
#69405=DIRECTION('ref_axis',(2.11176968422134E-16,-0.951056516295154,-0.309016994374945)) ;
#69406=DIRECTION('',(2.11176968422134E-16,-0.951056516295154,-0.309016994374948)) ;
#69407=DIRECTION('center_axis',(-1.,-2.22044604925031E-16,0.)) ;
#69408=DIRECTION('ref_axis',(2.22044604925031E-16,-1.,0.)) ;
#69409=DIRECTION('',(-1.79637858893621E-16,0.809016994374947,0.587785252292473)) ;
#69410=DIRECTION('center_axis',(1.,2.22044604925031E-16,0.)) ;
#69411=DIRECTION('ref_axis',(1.79637858893621E-16,-0.809016994374947,-0.587785252292474)) ;
#69412=DIRECTION('',(1.79637858893621E-16,-0.809016994374947,-0.587785252292473)) ;
#69413=DIRECTION('center_axis',(-1.,-2.22044604925031E-16,0.)) ;
#69414=DIRECTION('ref_axis',(2.22044604925031E-16,-1.,0.)) ;
#69415=DIRECTION('',(-1.30514544126042E-16,0.587785252292473,0.809016994374947)) ;
#69416=DIRECTION('center_axis',(1.,2.22044604925031E-16,0.)) ;
#69417=DIRECTION('ref_axis',(1.30514544126042E-16,-0.587785252292474,-0.809016994374947)) ;
#69418=DIRECTION('',(1.30514544126042E-16,-0.587785252292473,-0.809016994374947)) ;
#69419=DIRECTION('center_axis',(-1.,-2.22044604925031E-16,0.)) ;
#69420=DIRECTION('ref_axis',(2.22044604925031E-16,-1.,0.)) ;
#69421=DIRECTION('',(-6.86155564311058E-17,0.309016994374947,0.951056516295154)) ;
#69422=DIRECTION('center_axis',(1.,2.22044604925031E-16,0.)) ;
#69423=DIRECTION('ref_axis',(6.86155564311052E-17,-0.309016994374945,-0.951056516295154)) ;
#69424=DIRECTION('',(6.86155564311058E-17,-0.309016994374947,-0.951056516295154)) ;
#69425=DIRECTION('center_axis',(-1.,-2.22044604925031E-16,0.)) ;
#69426=DIRECTION('ref_axis',(2.22044604925031E-16,-1.,0.)) ;
#69427=DIRECTION('',(0.,0.,1.)) ;
#69428=DIRECTION('center_axis',(1.,2.22044604925031E-16,0.)) ;
#69429=DIRECTION('ref_axis',(0.,0.,-1.)) ;
#69430=DIRECTION('',(0.,0.,-1.)) ;
#69431=DIRECTION('center_axis',(-1.,-2.22044604925031E-16,0.)) ;
#69432=DIRECTION('ref_axis',(0.,0.,1.)) ;
#69433=DIRECTION('center_axis',(-1.,-2.22044604925031E-16,0.)) ;
#69434=DIRECTION('ref_axis',(3.47354289865169E-17,-0.156434465040232,0.987688340595138)) ;
#69435=DIRECTION('center_axis',(-6.86155564311058E-17,0.309016994374948,
-0.951056516295154)) ;
#69436=DIRECTION('ref_axis',(-0.707106781186557,0.672498511963948,0.218508012224408)) ;
#69437=DIRECTION('',(-6.86155564311058E-17,0.309016994374948,-0.951056516295154)) ;
#69438=DIRECTION('center_axis',(-2.46519032881566E-32,1.11022302462516E-16,
-1.)) ;
#69439=DIRECTION('ref_axis',(-0.707106781186547,-0.707106781186548,-7.8504622934189E-17)) ;
#69440=DIRECTION('',(2.46519032881566E-32,-1.11022302462516E-16,1.)) ;
#69441=DIRECTION('center_axis',(-6.86155564311058E-17,0.309016994374948,
-0.951056516295154)) ;
#69442=DIRECTION('ref_axis',(-0.707106781186557,-0.672498511963948,-0.218508012224408)) ;
#69443=DIRECTION('',(6.86155564311058E-17,-0.309016994374948,0.951056516295154)) ;
#69444=DIRECTION('center_axis',(-1.,-2.22044604925031E-16,0.)) ;
#69445=DIRECTION('ref_axis',(0.,0.,1.)) ;
#69446=DIRECTION('center_axis',(-1.30514544126042E-16,0.587785252292473,
-0.809016994374947)) ;
#69447=DIRECTION('ref_axis',(-0.707106781186563,0.572061402817672,0.415626937777444)) ;
#69448=DIRECTION('center_axis',(6.86155564311058E-17,-0.309016994374947,
-0.951056516295154)) ;
#69449=DIRECTION('ref_axis',(-0.707106781186557,-0.672498511963948,0.218508012224407)) ;
#69450=DIRECTION('',(-6.86155564311058E-17,0.309016994374947,0.951056516295154)) ;
#69451=DIRECTION('center_axis',(-1.30514544126042E-16,0.587785252292473,
-0.809016994374947)) ;
#69452=DIRECTION('ref_axis',(-0.707106781186551,-0.572061402817681,-0.415626937777451)) ;
#69453=DIRECTION('center_axis',(-1.,-2.22044604925031E-16,0.)) ;
#69454=DIRECTION('ref_axis',(0.,0.,1.)) ;
#69455=DIRECTION('center_axis',(-1.79637858893621E-16,0.809016994374948,
-0.587785252292473)) ;
#69456=DIRECTION('ref_axis',(-0.707106781186563,0.415626937777444,0.572061402817672)) ;
#69457=DIRECTION('center_axis',(1.30514544126042E-16,-0.587785252292473,
-0.809016994374948)) ;
#69458=DIRECTION('ref_axis',(-0.707106781186534,-0.572061402817695,0.415626937777461)) ;
#69459=DIRECTION('',(-1.30514544126042E-16,0.587785252292473,0.809016994374947)) ;
#69460=DIRECTION('center_axis',(-1.79637858893621E-16,0.809016994374948,
-0.587785252292473)) ;
#69461=DIRECTION('ref_axis',(-0.707106781186563,-0.415626937777444,-0.572061402817672)) ;
#69462=DIRECTION('center_axis',(-1.,-2.22044604925031E-16,0.)) ;
#69463=DIRECTION('ref_axis',(0.,0.,1.)) ;
#69464=DIRECTION('center_axis',(-2.11176968422134E-16,0.951056516295154,
-0.309016994374947)) ;
#69465=DIRECTION('ref_axis',(-0.707106781186557,0.218508012224407,0.672498511963949)) ;
#69466=DIRECTION('center_axis',(1.79637858893621E-16,-0.809016994374947,
-0.587785252292473)) ;
#69467=DIRECTION('ref_axis',(-0.707106781186551,-0.415626937777452,0.572061402817682)) ;
#69468=DIRECTION('',(-1.79637858893621E-16,0.809016994374947,0.587785252292473)) ;
#69469=DIRECTION('center_axis',(-2.11176968422134E-16,0.951056516295154,
-0.309016994374947)) ;
#69470=DIRECTION('ref_axis',(-0.707106781186557,-0.218508012224407,-0.672498511963948)) ;
#69471=DIRECTION('center_axis',(-1.,-2.22044604925031E-16,0.)) ;
#69472=DIRECTION('ref_axis',(0.,0.,1.)) ;
#69473=DIRECTION('center_axis',(-2.22044604925031E-16,1.,5.55111512312578E-17)) ;
#69474=DIRECTION('ref_axis',(-0.707106781186568,-1.96261557335475E-16,0.707106781186527)) ;
#69475=DIRECTION('center_axis',(2.11176968422134E-16,-0.951056516295154,
-0.309016994374948)) ;
#69476=DIRECTION('ref_axis',(-0.707106781186583,-0.2185080122244,0.672498511963923)) ;
#69477=DIRECTION('',(-2.11176968422134E-16,0.951056516295153,0.309016994374948)) ;
#69478=DIRECTION('center_axis',(-2.22044604925031E-16,1.,5.55111512312578E-17)) ;
#69479=DIRECTION('ref_axis',(-0.707106781186568,-1.17756934401289E-16,-0.707106781186527)) ;
#69480=DIRECTION('center_axis',(-1.,-2.22044604925031E-16,0.)) ;
#69481=DIRECTION('ref_axis',(0.,0.,1.)) ;
#69482=DIRECTION('center_axis',(-2.11176968422134E-16,0.951056516295154,
0.309016994374948)) ;
#69483=DIRECTION('ref_axis',(-0.707106781186557,-0.218508012224408,0.672498511963948)) ;
#69484=DIRECTION('center_axis',(2.22044604925031E-16,-1.,-2.22044604925031E-16)) ;
#69485=DIRECTION('ref_axis',(-0.707106781186568,-3.14018491736755E-16,0.707106781186527)) ;
#69486=DIRECTION('',(-2.22044604925031E-16,1.,2.22044604925031E-16)) ;
#69487=DIRECTION('center_axis',(-2.11176968422134E-16,0.951056516295154,
0.309016994374948)) ;
#69488=DIRECTION('ref_axis',(-0.707106781186557,0.218508012224408,-0.672498511963948)) ;
#69489=DIRECTION('center_axis',(-1.,-2.22044604925031E-16,0.)) ;
#69490=DIRECTION('ref_axis',(0.,0.,1.)) ;
#69491=DIRECTION('center_axis',(-1.79637858893621E-16,0.809016994374947,
0.587785252292473)) ;
#69492=DIRECTION('ref_axis',(-0.707106781186563,-0.415626937777444,0.572061402817672)) ;
#69493=DIRECTION('center_axis',(2.11176968422134E-16,-0.951056516295154,
0.309016994374947)) ;
#69494=DIRECTION('ref_axis',(-0.707106781186563,0.218508012224405,0.672498511963943)) ;
#69495=DIRECTION('',(-2.11176968422134E-16,0.951056516295154,-0.309016994374947)) ;
#69496=DIRECTION('center_axis',(-1.79637858893621E-16,0.809016994374947,
0.587785252292473)) ;
#69497=DIRECTION('ref_axis',(-0.707106781186568,0.415626937777441,-0.572061402817668)) ;
#69498=DIRECTION('center_axis',(-1.,-2.22044604925031E-16,0.)) ;
#69499=DIRECTION('ref_axis',(0.,0.,1.)) ;
#69500=DIRECTION('center_axis',(-1.30514544126042E-16,0.587785252292473,
0.809016994374948)) ;
#69501=DIRECTION('ref_axis',(-0.707106781186563,-0.572061402817672,0.415626937777444)) ;
#69502=DIRECTION('center_axis',(1.79637858893621E-16,-0.809016994374948,
0.587785252292473)) ;
#69503=DIRECTION('ref_axis',(-0.707106781186551,0.415626937777451,0.572061402817682)) ;
#69504=DIRECTION('',(-1.79637858893621E-16,0.809016994374948,-0.587785252292473)) ;
#69505=DIRECTION('center_axis',(-1.30514544126042E-16,0.587785252292473,
0.809016994374948)) ;
#69506=DIRECTION('ref_axis',(-0.707106781186551,0.572061402817682,-0.415626937777451)) ;
#69507=DIRECTION('center_axis',(-1.,-2.22044604925031E-16,0.)) ;
#69508=DIRECTION('ref_axis',(0.,0.,1.)) ;
#69509=DIRECTION('center_axis',(-6.86155564311058E-17,0.309016994374947,
0.951056516295154)) ;
#69510=DIRECTION('ref_axis',(-0.707106781186557,-0.672498511963948,0.218508012224407)) ;
#69511=DIRECTION('center_axis',(1.30514544126042E-16,-0.587785252292473,
0.809016994374947)) ;
#69512=DIRECTION('ref_axis',(-0.707106781186534,0.572061402817695,0.415626937777462)) ;
#69513=DIRECTION('',(-1.30514544126042E-16,0.587785252292473,-0.809016994374947)) ;
#69514=DIRECTION('center_axis',(-6.86155564311058E-17,0.309016994374947,
0.951056516295154)) ;
#69515=DIRECTION('ref_axis',(-0.707106781186557,0.672498511963948,-0.218508012224407)) ;
#69516=DIRECTION('center_axis',(-1.,-2.22044604925031E-16,0.)) ;
#69517=DIRECTION('ref_axis',(0.,0.,1.)) ;
#69518=DIRECTION('center_axis',(0.,0.,1.)) ;
#69519=DIRECTION('ref_axis',(-0.707106781186568,-0.707106781186527,0.)) ;
#69520=DIRECTION('center_axis',(6.86155564311059E-17,-0.309016994374948,
0.951056516295154)) ;
#69521=DIRECTION('ref_axis',(-0.707106781186557,0.672498511963948,0.218508012224408)) ;
#69522=DIRECTION('center_axis',(0.,0.,1.)) ;
#69523=DIRECTION('ref_axis',(-0.707106781186589,0.707106781186506,0.)) ;
#69524=DIRECTION('center_axis',(-1.,-2.22044604925031E-16,0.)) ;
#69525=DIRECTION('ref_axis',(0.,0.,1.)) ;
#69526=DIRECTION('center_axis',(6.86155564311059E-17,-0.309016994374948,
0.951056516295154)) ;
#69527=DIRECTION('ref_axis',(-0.707106781186557,-0.672498511963948,-0.218508012224408)) ;
#69528=DIRECTION('center_axis',(-1.,-2.22044604925031E-16,0.)) ;
#69529=DIRECTION('ref_axis',(0.,0.309016994374018,-0.951056516295456)) ;
#69530=DIRECTION('center_axis',(-1.,-2.22044604925031E-16,0.)) ;
#69531=DIRECTION('ref_axis',(0.,-3.41060513164848E-13,-1.)) ;
#69532=DIRECTION('center_axis',(-1.,-2.22044604925031E-16,0.)) ;
#69533=DIRECTION('ref_axis',(0.,0.,1.)) ;
#69534=DIRECTION('center_axis',(-1.,-2.22044604925031E-16,0.)) ;
#69535=DIRECTION('ref_axis',(-1.00806141154385E-16,0.453990499739547,-0.891006524188368)) ;
#69536=DIRECTION('center_axis',(1.30514544126042E-16,-0.587785252292473,
0.809016994374947)) ;
#69537=DIRECTION('ref_axis',(-0.707106781186534,-0.572061402817695,-0.415626937777461)) ;
#69538=DIRECTION('',(1.30514544126042E-16,-0.587785252292473,0.809016994374947)) ;
#69539=DIRECTION('center_axis',(-1.,-2.22044604925031E-16,0.)) ;
#69540=DIRECTION('ref_axis',(0.,0.587785252293422,-0.809016994374258)) ;
#69541=DIRECTION('center_axis',(-1.,-2.22044604925031E-16,0.)) ;
#69542=DIRECTION('ref_axis',(-1.30514544126041E-16,0.587785252292468,-0.809016994374951)) ;
#69543=DIRECTION('center_axis',(-1.,-2.22044604925031E-16,0.)) ;
#69544=DIRECTION('ref_axis',(0.,-0.309016994375666,-0.95105651629492)) ;
#69545=DIRECTION('center_axis',(-1.,-2.22044604925031E-16,0.)) ;
#69546=DIRECTION('ref_axis',(0.,0.,1.)) ;
#69547=DIRECTION('center_axis',(-1.,-2.22044604925031E-16,0.)) ;
#69548=DIRECTION('ref_axis',(-1.57009245868377E-16,0.707106781186547,-0.707106781186547)) ;
#69549=DIRECTION('center_axis',(1.79637858893621E-16,-0.809016994374948,
0.587785252292473)) ;
#69550=DIRECTION('ref_axis',(-0.707106781186575,-0.415626937777437,-0.572061402817662)) ;
#69551=DIRECTION('',(1.79637858893621E-16,-0.809016994374948,0.587785252292473)) ;
#69552=DIRECTION('center_axis',(-1.,-2.22044604925031E-16,0.)) ;
#69553=DIRECTION('ref_axis',(0.,0.809016994375283,-0.587785252292011)) ;
#69554=DIRECTION('center_axis',(-1.,-2.22044604925031E-16,0.)) ;
#69555=DIRECTION('ref_axis',(-1.79637858893621E-16,0.809016994374947,-0.587785252292474)) ;
#69556=DIRECTION('center_axis',(-1.,-2.22044604925031E-16,0.)) ;
#69557=DIRECTION('ref_axis',(0.,-0.587785252292347,-0.809016994375039)) ;
#69558=DIRECTION('center_axis',(-1.,-2.22044604925031E-16,0.)) ;
#69559=DIRECTION('ref_axis',(0.,0.,1.)) ;
#69560=DIRECTION('center_axis',(-1.,-2.22044604925031E-16,0.)) ;
#69561=DIRECTION('ref_axis',(-1.97843191649031E-16,0.891006524188368,-0.453990499739547)) ;
#69562=DIRECTION('center_axis',(2.11176968422134E-16,-0.951056516295154,
0.309016994374947)) ;
#69563=DIRECTION('ref_axis',(-0.707106781186563,-0.218508012224406,-0.672498511963943)) ;
#69564=DIRECTION('',(2.11176968422134E-16,-0.951056516295154,0.309016994374947)) ;
#69565=DIRECTION('center_axis',(-1.,-2.22044604925031E-16,0.)) ;
#69566=DIRECTION('ref_axis',(0.,0.951056516294897,-0.309016994375738)) ;
#69567=DIRECTION('center_axis',(-1.,-2.22044604925031E-16,0.)) ;
#69568=DIRECTION('ref_axis',(-2.11176968422134E-16,0.951056516295153,-0.309016994374948)) ;
#69569=DIRECTION('center_axis',(-1.,-2.22044604925031E-16,0.)) ;
#69570=DIRECTION('ref_axis',(0.,-0.809016994374792,-0.587785252292687)) ;
#69571=DIRECTION('center_axis',(-1.,-2.22044604925031E-16,0.)) ;
#69572=DIRECTION('ref_axis',(0.,0.,1.)) ;
#69573=DIRECTION('center_axis',(-1.,-2.22044604925031E-16,0.)) ;
#69574=DIRECTION('ref_axis',(-2.19310867376507E-16,0.987688340595138,-0.156434465040228)) ;
#69575=DIRECTION('center_axis',(2.22044604925031E-16,-1.,-2.22044604925031E-16)) ;
#69576=DIRECTION('ref_axis',(-0.707106781186568,-9.08458920382451E-30,-0.707106781186527)) ;
#69577=DIRECTION('',(2.22044604925031E-16,-1.,-2.22044604925031E-16)) ;
#69578=DIRECTION('center_axis',(-1.,-2.22044604925031E-16,0.)) ;
#69579=DIRECTION('ref_axis',(0.,1.,-4.9737991503207E-14)) ;
#69580=DIRECTION('center_axis',(-1.,-2.22044604925031E-16,0.)) ;
#69581=DIRECTION('ref_axis',(-2.22044604925031E-16,1.,0.)) ;
#69582=DIRECTION('center_axis',(-1.,-2.22044604925031E-16,0.)) ;
#69583=DIRECTION('ref_axis',(0.,-0.951056516295317,-0.309016994374445)) ;
#69584=DIRECTION('center_axis',(-1.,-2.22044604925031E-16,0.)) ;
#69585=DIRECTION('ref_axis',(0.,0.,1.)) ;
#69586=DIRECTION('center_axis',(-1.,-2.22044604925031E-16,0.)) ;
#69587=DIRECTION('ref_axis',(-2.19310867376507E-16,0.987688340595138,0.156434465040232)) ;
#69588=DIRECTION('center_axis',(2.11176968422134E-16,-0.951056516295154,
-0.309016994374948)) ;
#69589=DIRECTION('ref_axis',(-0.707106781186563,0.218508012224406,-0.672498511963942)) ;
#69590=DIRECTION('',(2.11176968422134E-16,-0.951056516295153,-0.309016994374948)) ;
#69591=DIRECTION('center_axis',(-1.,-2.22044604925031E-16,0.)) ;
#69592=DIRECTION('ref_axis',(0.,0.,1.)) ;
#69593=DIRECTION('center_axis',(-1.,-2.22044604925031E-16,0.)) ;
#69594=DIRECTION('ref_axis',(-2.11176968422134E-16,0.951056516295153,0.309016994374948)) ;
#69595=DIRECTION('center_axis',(-1.,-2.22044604925031E-16,0.)) ;
#69596=DIRECTION('ref_axis',(0.,-1.,5.04485342389671E-13)) ;
#69597=DIRECTION('center_axis',(-1.,-2.22044604925031E-16,0.)) ;
#69598=DIRECTION('ref_axis',(0.,0.,1.)) ;
#69599=DIRECTION('center_axis',(-1.,-2.22044604925031E-16,0.)) ;
#69600=DIRECTION('ref_axis',(-1.97843191649031E-16,0.891006524188368,0.453990499739546)) ;
#69601=DIRECTION('center_axis',(1.79637858893621E-16,-0.809016994374947,
-0.587785252292473)) ;
#69602=DIRECTION('ref_axis',(-0.707106781186592,0.415626937777427,-0.572061402817648)) ;
#69603=DIRECTION('',(1.79637858893621E-16,-0.809016994374947,-0.587785252292473)) ;
#69604=DIRECTION('center_axis',(-1.,-2.22044604925031E-16,0.)) ;
#69605=DIRECTION('ref_axis',(0.,0.,1.)) ;
#69606=DIRECTION('center_axis',(-1.,-2.22044604925031E-16,0.)) ;
#69607=DIRECTION('ref_axis',(-1.79637858893621E-16,0.809016994374947,0.587785252292474)) ;
#69608=DIRECTION('center_axis',(-1.,-2.22044604925031E-16,0.)) ;
#69609=DIRECTION('ref_axis',(0.,0.,1.)) ;
#69610=DIRECTION('center_axis',(-1.,-2.22044604925031E-16,0.)) ;
#69611=DIRECTION('ref_axis',(0.,0.,1.)) ;
#69612=DIRECTION('center_axis',(-1.,-2.22044604925031E-16,0.)) ;
#69613=DIRECTION('ref_axis',(-1.57009245868377E-16,0.707106781186548,0.707106781186547)) ;
#69614=DIRECTION('center_axis',(1.30514544126042E-16,-0.587785252292473,
-0.809016994374948)) ;
#69615=DIRECTION('ref_axis',(-0.707106781186568,0.572061402817668,-0.415626937777441)) ;
#69616=DIRECTION('',(1.30514544126042E-16,-0.587785252292473,-0.809016994374947)) ;
#69617=DIRECTION('center_axis',(-1.,-2.22044604925031E-16,0.)) ;
#69618=DIRECTION('ref_axis',(0.,0.,1.)) ;
#69619=DIRECTION('center_axis',(-1.,-2.22044604925031E-16,0.)) ;
#69620=DIRECTION('ref_axis',(-1.30514544126041E-16,0.587785252292468,0.809016994374951)) ;
#69621=DIRECTION('center_axis',(-1.,-2.22044604925031E-16,0.)) ;
#69622=DIRECTION('ref_axis',(0.,0.,1.)) ;
#69623=DIRECTION('center_axis',(-1.,-2.22044604925031E-16,0.)) ;
#69624=DIRECTION('ref_axis',(0.,0.,1.)) ;
#69625=DIRECTION('center_axis',(-1.,-2.22044604925031E-16,0.)) ;
#69626=DIRECTION('ref_axis',(-1.00806141154386E-16,0.453990499739549,0.891006524188367)) ;
#69627=DIRECTION('center_axis',(6.86155564311058E-17,-0.309016994374947,
-0.951056516295154)) ;
#69628=DIRECTION('ref_axis',(-0.707106781186557,0.672498511963948,-0.218508012224407)) ;
#69629=DIRECTION('',(6.86155564311058E-17,-0.309016994374947,-0.951056516295154)) ;
#69630=DIRECTION('center_axis',(-1.,-2.22044604925031E-16,0.)) ;
#69631=DIRECTION('ref_axis',(0.,0.,1.)) ;
#69632=DIRECTION('center_axis',(-1.,-2.22044604925031E-16,0.)) ;
#69633=DIRECTION('ref_axis',(-6.86155564311052E-17,0.309016994374945,0.951056516295154)) ;
#69634=DIRECTION('center_axis',(-1.,-2.22044604925031E-16,0.)) ;
#69635=DIRECTION('ref_axis',(0.,0.,1.)) ;
#69636=DIRECTION('center_axis',(-1.,-2.22044604925031E-16,0.)) ;
#69637=DIRECTION('ref_axis',(0.,0.,1.)) ;
#69638=DIRECTION('center_axis',(-1.,-2.22044604925031E-16,0.)) ;
#69639=DIRECTION('ref_axis',(-3.47354289865171E-17,0.156434465040233,0.987688340595137)) ;
#69640=DIRECTION('center_axis',(-2.46519032881566E-32,1.11022302462516E-16,
-1.)) ;
#69641=DIRECTION('ref_axis',(-0.707106781186589,0.707106781186506,7.85046229341844E-17)) ;
#69642=DIRECTION('',(-2.46519032881566E-32,1.11022302462516E-16,-1.)) ;
#69643=DIRECTION('center_axis',(-1.,-2.22044604925031E-16,0.)) ;
#69644=DIRECTION('ref_axis',(0.,0.,1.)) ;
#69645=DIRECTION('center_axis',(-1.,-2.22044604925031E-16,0.)) ;
#69646=DIRECTION('ref_axis',(0.,0.,1.)) ;
#69647=DIRECTION('center_axis',(-1.,-2.22044604925031E-16,0.)) ;
#69648=DIRECTION('ref_axis',(0.,0.,1.)) ;
#69649=DIRECTION('center_axis',(-1.,-2.22044604925031E-16,0.)) ;
#69650=DIRECTION('ref_axis',(6.86155564311052E-17,-0.309016994374945,0.951056516295154)) ;
#69651=DIRECTION('center_axis',(1.,2.22044604925031E-16,0.)) ;
#69652=DIRECTION('ref_axis',(2.22044604925031E-16,-1.,0.)) ;
#69653=DIRECTION('',(-1.,-2.22044604925031E-16,0.)) ;
#69654=DIRECTION('',(1.,2.22044604925031E-16,0.)) ;
#69655=DIRECTION('center_axis',(-2.11176968422134E-16,0.951056516295154,
0.309016994374948)) ;
#69656=DIRECTION('ref_axis',(6.86155564311058E-17,-0.309016994374948,0.951056516295154)) ;
#69657=DIRECTION('',(1.,2.22044604925031E-16,0.)) ;
#69658=DIRECTION('center_axis',(1.,2.22044604925031E-16,0.)) ;
#69659=DIRECTION('ref_axis',(6.8615556431103E-17,-0.309016994374935,0.951056516295158)) ;
#69660=DIRECTION('',(1.,2.22044604925031E-16,0.)) ;
#69661=DIRECTION('center_axis',(2.11176968422134E-16,-0.951056516295154,
-0.309016994374948)) ;
#69662=DIRECTION('ref_axis',(-6.86155564311058E-17,0.309016994374948,-0.951056516295154)) ;
#69663=DIRECTION('center_axis',(1.79637858893621E-16,-0.809016994374947,
-0.587785252292473)) ;
#69664=DIRECTION('ref_axis',(-1.30514544126042E-16,0.587785252292473,-0.809016994374947)) ;
#69665=DIRECTION('',(1.,2.22044604925031E-16,0.)) ;
#69666=DIRECTION('',(1.,2.22044604925031E-16,0.)) ;
#69667=DIRECTION('center_axis',(-1.79637858893621E-16,0.809016994374947,
0.587785252292473)) ;
#69668=DIRECTION('ref_axis',(1.30514544126042E-16,-0.587785252292473,0.809016994374947)) ;
#69669=DIRECTION('',(1.,2.22044604925031E-16,0.)) ;
#69670=DIRECTION('',(-1.,-2.22044604925031E-16,0.)) ;
#69671=DIRECTION('center_axis',(1.,2.22044604925031E-16,0.)) ;
#69672=DIRECTION('ref_axis',(-1.3051454412604E-16,0.587785252292467,-0.809016994374952)) ;
#69673=DIRECTION('center_axis',(1.30514544126042E-16,-0.587785252292473,
-0.809016994374948)) ;
#69674=DIRECTION('ref_axis',(-1.79637858893621E-16,0.809016994374948,-0.587785252292473)) ;
#69675=DIRECTION('',(1.,2.22044604925031E-16,0.)) ;
#69676=DIRECTION('',(1.,2.22044604925031E-16,0.)) ;
#69677=DIRECTION('center_axis',(-1.30514544126042E-16,0.587785252292473,
0.809016994374948)) ;
#69678=DIRECTION('ref_axis',(1.79637858893621E-16,-0.809016994374948,0.587785252292473)) ;
#69679=DIRECTION('',(1.,2.22044604925031E-16,0.)) ;
#69680=DIRECTION('',(-1.,-2.22044604925031E-16,0.)) ;
#69681=DIRECTION('center_axis',(1.,2.22044604925031E-16,0.)) ;
#69682=DIRECTION('ref_axis',(-1.79637858893622E-16,0.809016994374951,-0.587785252292468)) ;
#69683=DIRECTION('center_axis',(6.86155564311058E-17,-0.309016994374947,
-0.951056516295154)) ;
#69684=DIRECTION('ref_axis',(-2.11176968422134E-16,0.951056516295154,-0.309016994374947)) ;
#69685=DIRECTION('',(1.,2.22044604925031E-16,0.)) ;
#69686=DIRECTION('',(1.,2.22044604925031E-16,0.)) ;
#69687=DIRECTION('center_axis',(-6.86155564311058E-17,0.309016994374947,
0.951056516295154)) ;
#69688=DIRECTION('ref_axis',(2.11176968422134E-16,-0.951056516295154,0.309016994374947)) ;
#69689=DIRECTION('',(1.,2.22044604925031E-16,0.)) ;
#69690=DIRECTION('',(-1.,-2.22044604925031E-16,0.)) ;
#69691=DIRECTION('center_axis',(1.,2.22044604925031E-16,0.)) ;
#69692=DIRECTION('ref_axis',(-2.11176968422134E-16,0.951056516295157,-0.309016994374937)) ;
#69693=DIRECTION('center_axis',(-4.93038065763132E-32,2.22044604925031E-16,
-1.)) ;
#69694=DIRECTION('ref_axis',(-2.22044604925031E-16,1.,2.22044604925031E-16)) ;
#69695=DIRECTION('',(1.,2.22044604925031E-16,0.)) ;
#69696=DIRECTION('',(1.,2.22044604925031E-16,0.)) ;
#69697=DIRECTION('center_axis',(4.93038065763132E-32,-2.22044604925031E-16,
1.)) ;
#69698=DIRECTION('ref_axis',(2.22044604925031E-16,-1.,-2.22044604925031E-16)) ;
#69699=DIRECTION('',(1.,2.22044604925031E-16,0.)) ;
#69700=DIRECTION('',(-1.,-2.22044604925031E-16,0.)) ;
#69701=DIRECTION('center_axis',(1.,2.22044604925031E-16,0.)) ;
#69702=DIRECTION('ref_axis',(-2.22044604925031E-16,1.,-7.51101277651833E-17)) ;
#69703=DIRECTION('center_axis',(-6.86155564311059E-17,0.309016994374948,
-0.951056516295154)) ;
#69704=DIRECTION('ref_axis',(-2.11176968422134E-16,0.951056516295154,0.309016994374948)) ;
#69705=DIRECTION('',(1.,2.22044604925031E-16,0.)) ;
#69706=DIRECTION('',(1.,2.22044604925031E-16,0.)) ;
#69707=DIRECTION('center_axis',(6.86155564311059E-17,-0.309016994374948,
0.951056516295154)) ;
#69708=DIRECTION('ref_axis',(2.11176968422134E-16,-0.951056516295154,-0.309016994374948)) ;
#69709=DIRECTION('',(1.,2.22044604925031E-16,0.)) ;
#69710=DIRECTION('',(-1.,-2.22044604925031E-16,0.)) ;
#69711=DIRECTION('center_axis',(1.,2.22044604925031E-16,0.)) ;
#69712=DIRECTION('ref_axis',(-2.11176968422134E-16,0.951056516295157,0.309016994374937)) ;
#69713=DIRECTION('center_axis',(-1.30514544126042E-16,0.587785252292473,
-0.809016994374947)) ;
#69714=DIRECTION('ref_axis',(-1.79637858893621E-16,0.809016994374947,0.587785252292473)) ;
#69715=DIRECTION('',(1.,2.22044604925031E-16,0.)) ;
#69716=DIRECTION('',(1.,2.22044604925031E-16,0.)) ;
#69717=DIRECTION('center_axis',(1.30514544126042E-16,-0.587785252292473,
0.809016994374947)) ;
#69718=DIRECTION('ref_axis',(1.79637858893621E-16,-0.809016994374947,-0.587785252292473)) ;
#69719=DIRECTION('',(1.,2.22044604925031E-16,0.)) ;
#69720=DIRECTION('',(-1.,-2.22044604925031E-16,0.)) ;
#69721=DIRECTION('center_axis',(1.,2.22044604925031E-16,0.)) ;
#69722=DIRECTION('ref_axis',(-1.79637858893622E-16,0.80901699437495,0.587785252292469)) ;
#69723=DIRECTION('center_axis',(-1.79637858893621E-16,0.809016994374948,
-0.587785252292473)) ;
#69724=DIRECTION('ref_axis',(-1.30514544126042E-16,0.587785252292473,0.809016994374948)) ;
#69725=DIRECTION('',(1.,2.22044604925031E-16,0.)) ;
#69726=DIRECTION('',(1.,2.22044604925031E-16,0.)) ;
#69727=DIRECTION('center_axis',(1.79637858893621E-16,-0.809016994374948,
0.587785252292473)) ;
#69728=DIRECTION('ref_axis',(1.30514544126042E-16,-0.587785252292473,-0.809016994374948)) ;
#69729=DIRECTION('',(1.,2.22044604925031E-16,0.)) ;
#69730=DIRECTION('',(-1.,-2.22044604925031E-16,0.)) ;
#69731=DIRECTION('center_axis',(1.,2.22044604925031E-16,0.)) ;
#69732=DIRECTION('ref_axis',(-1.30514544126041E-16,0.587785252292468,0.809016994374951)) ;
#69733=DIRECTION('center_axis',(-2.11176968422134E-16,0.951056516295154,
-0.309016994374947)) ;
#69734=DIRECTION('ref_axis',(-6.86155564311058E-17,0.309016994374947,0.951056516295154)) ;
#69735=DIRECTION('',(1.,2.22044604925031E-16,0.)) ;
#69736=DIRECTION('',(1.,2.22044604925031E-16,0.)) ;
#69737=DIRECTION('center_axis',(2.11176968422134E-16,-0.951056516295154,
0.309016994374947)) ;
#69738=DIRECTION('ref_axis',(6.86155564311058E-17,-0.309016994374947,-0.951056516295154)) ;
#69739=DIRECTION('',(1.,2.22044604925031E-16,0.)) ;
#69740=DIRECTION('',(-1.,-2.22044604925031E-16,0.)) ;
#69741=DIRECTION('center_axis',(1.,2.22044604925031E-16,0.)) ;
#69742=DIRECTION('ref_axis',(-6.8615556431105E-17,0.309016994374944,0.951056516295155)) ;
#69743=DIRECTION('center_axis',(-2.22044604925031E-16,1.,1.11022302462516E-16)) ;
#69744=DIRECTION('ref_axis',(2.46519032881566E-32,-1.11022302462516E-16,
1.)) ;
#69745=DIRECTION('',(1.,2.22044604925031E-16,0.)) ;
#69746=DIRECTION('',(1.,2.22044604925031E-16,0.)) ;
#69747=DIRECTION('center_axis',(2.22044604925031E-16,-1.,-1.11022302462516E-16)) ;
#69748=DIRECTION('ref_axis',(-2.46519032881566E-32,1.11022302462516E-16,
-1.)) ;
#69749=DIRECTION('',(1.,2.22044604925031E-16,0.)) ;
#69750=DIRECTION('center_axis',(1.,2.22044604925031E-16,0.)) ;
#69751=DIRECTION('ref_axis',(-2.01194122103066E-30,9.06097773332504E-15,
1.)) ;
#69752=DIRECTION('center_axis',(1.,2.22044604925031E-16,0.)) ;
#69753=DIRECTION('ref_axis',(2.22044604925031E-16,-1.,0.)) ;
#69754=DIRECTION('center_axis',(1.,2.22044604925031E-16,0.)) ;
#69755=DIRECTION('ref_axis',(2.22044604925031E-16,-1.,0.)) ;
#69756=DIRECTION('center_axis',(1.,2.22044604925031E-16,0.)) ;
#69757=DIRECTION('ref_axis',(2.22044604925031E-16,-1.,0.)) ;
#69758=DIRECTION('center_axis',(1.,2.22044604925031E-16,0.)) ;
#69759=DIRECTION('ref_axis',(2.22044604925031E-16,-1.,0.)) ;
#69760=DIRECTION('center_axis',(1.,2.22044604925031E-16,0.)) ;
#69761=DIRECTION('ref_axis',(2.22044604925031E-16,-1.,0.)) ;
#69762=DIRECTION('center_axis',(1.,2.22044604925031E-16,0.)) ;
#69763=DIRECTION('ref_axis',(2.22044604925031E-16,-1.,0.)) ;
#69764=DIRECTION('center_axis',(1.,2.22044604925031E-16,0.)) ;
#69765=DIRECTION('ref_axis',(2.22044604925031E-16,-1.,0.)) ;
#69766=DIRECTION('center_axis',(1.,2.22044604925031E-16,0.)) ;
#69767=DIRECTION('ref_axis',(2.22044604925031E-16,-1.,0.)) ;
#69768=DIRECTION('center_axis',(1.,2.22044604925031E-16,0.)) ;
#69769=DIRECTION('ref_axis',(2.22044604925031E-16,-1.,0.)) ;
#69770=DIRECTION('center_axis',(1.,2.22044604925031E-16,0.)) ;
#69771=DIRECTION('ref_axis',(2.22044604925031E-16,-1.,0.)) ;
#69772=DIRECTION('',(1.,2.22044604925031E-16,0.)) ;
#105464=CARTESIAN_POINT('',(0.,0.,0.)) ;
#105465=CARTESIAN_POINT('Origin',(66.4402651077866,248.040265107786,23.0213203435596)) ;
#105466=CARTESIAN_POINT('',(66.1902651077865,245.040265107786,23.0213203435596)) ;
#105467=CARTESIAN_POINT('Origin',(66.1902651077865,248.040265107786,23.0213203435596)) ;
#105468=CARTESIAN_POINT('',(65.4402651077865,244.072019271234,23.0213203435596)) ;
#105469=CARTESIAN_POINT('Origin',(66.4402651077866,244.072019271234,23.0213203435596)) ;
#105470=CARTESIAN_POINT('Origin',(65.4402651077865,248.040265107786,23.0213203435596)) ;
#105471=CARTESIAN_POINT('Origin',(65.4402651077865,248.040265107786,23.0213203435596)) ;
#105472=CARTESIAN_POINT('',(65.4402651077865,252.442540694976,23.0172786696089)) ;
#105473=CARTESIAN_POINT('Ctrl Pts',(65.4402651077866,252.442540694976,23.0172786696089)) ;
#105474=CARTESIAN_POINT('Ctrl Pts',(65.4402651077866,252.44193825915,22.3610929985028)) ;
#105475=CARTESIAN_POINT('Ctrl Pts',(65.4402651077866,252.140233304353,21.0448319450019)) ;
#105476=CARTESIAN_POINT('Ctrl Pts',(65.4402651077865,250.873971934894,19.4582865154112)) ;
#105477=CARTESIAN_POINT('Ctrl Pts',(65.4402651077866,249.045854854551,18.5832034982517)) ;
#105478=CARTESIAN_POINT('Ctrl Pts',(65.4402651077866,247.020059922002,18.5850672640655)) ;
#105479=CARTESIAN_POINT('Ctrl Pts',(65.4402651077866,245.192236164937,19.4697890066313)) ;
#105480=CARTESIAN_POINT('Ctrl Pts',(65.4402651077866,243.935614231154,21.0547463401441)) ;
#105481=CARTESIAN_POINT('Ctrl Pts',(65.4402651077866,243.488804604471,23.0179171559172)) ;
#105482=CARTESIAN_POINT('Ctrl Pts',(65.4402651077866,243.938490009196,24.9980925373954)) ;
#105483=CARTESIAN_POINT('Ctrl Pts',(65.4402651077866,245.203459264903,26.5808573752723)) ;
#105484=CARTESIAN_POINT('Ctrl Pts',(65.4402651077866,247.029377891764,27.4604808473129)) ;
#105485=CARTESIAN_POINT('Ctrl Pts',(65.4402651077865,249.055861093547,27.4588462212786)) ;
#105486=CARTESIAN_POINT('Ctrl Pts',(65.4402651077866,250.87986399868,26.5790375520551)) ;
#105487=CARTESIAN_POINT('Ctrl Pts',(65.4402651077865,252.145441264101,24.9929395133859)) ;
#105488=CARTESIAN_POINT('Ctrl Pts',(65.4402651077865,252.443143130803,23.6734643407148)) ;
#105489=CARTESIAN_POINT('Ctrl Pts',(65.4402651077865,252.442540694976,23.0172786696089)) ;
#105490=CARTESIAN_POINT('Origin',(58.9402651077865,248.040265107786,23.0213203435596)) ;
#105491=CARTESIAN_POINT('',(59.9402651077865,248.040265107786,27.0213203435596)) ;
#105492=CARTESIAN_POINT('Origin',(59.9402651077865,248.040265107786,23.0213203435596)) ;
#105493=CARTESIAN_POINT('',(58.9402651077865,248.040265107786,26.0213203435596)) ;
#105494=CARTESIAN_POINT('Origin',(58.9402651077865,248.040265107786,27.0213203435596)) ;
#105495=CARTESIAN_POINT('Origin',(58.9402651077865,248.040265107786,23.0213203435596)) ;
#105496=CARTESIAN_POINT('Origin',(59.9402651077865,248.040265107786,23.0213203435596)) ;
#105497=CARTESIAN_POINT('',(59.9402651077865,252.442541339505,23.0245853614825)) ;
#105498=CARTESIAN_POINT('Ctrl Pts',(59.9402651077865,252.442541339505,23.0245853614825)) ;
#105499=CARTESIAN_POINT('Ctrl Pts',(59.9402651077865,252.442054668933,23.6807711286595)) ;
#105500=CARTESIAN_POINT('Ctrl Pts',(59.9402651077865,252.140582866504,24.9970918038166)) ;
#105501=CARTESIAN_POINT('Ctrl Pts',(59.9402651077865,250.874603529792,26.5838602800608)) ;
#105502=CARTESIAN_POINT('Ctrl Pts',(59.9402651077865,249.046642816666,27.4592688287601)) ;
#105503=CARTESIAN_POINT('Ctrl Pts',(59.9402651077865,247.02084725416,27.457759936616)) ;
#105504=CARTESIAN_POINT('Ctrl Pts',(59.9402651077865,245.192869526073,26.5733619136289)) ;
#105505=CARTESIAN_POINT('Ctrl Pts',(59.9402651077865,243.935964506927,24.9886198977872)) ;
#105506=CARTESIAN_POINT('Ctrl Pts',(59.9402651077865,243.488807364186,23.0255250811106)) ;
#105507=CARTESIAN_POINT('Ctrl Pts',(59.9402651077865,243.938143019334,21.0452698397019)) ;
#105508=CARTESIAN_POINT('Ctrl Pts',(59.9402651077865,245.202832783418,19.462280744107)) ;
#105509=CARTESIAN_POINT('Ctrl Pts',(59.9402651077865,247.028596667264,18.582335498899)) ;
#105510=CARTESIAN_POINT('Ctrl Pts',(59.9402651077865,249.055081848073,18.5836132230762)) ;
#105511=CARTESIAN_POINT('Ctrl Pts',(59.9402651077865,250.87923966532,19.4631003199451)) ;
#105512=CARTESIAN_POINT('Ctrl Pts',(59.9402651077865,252.145094800052,21.0489759066127)) ;
#105513=CARTESIAN_POINT('Ctrl Pts',(59.9402651077865,252.443028010077,22.3683995943057)) ;
#105514=CARTESIAN_POINT('Ctrl Pts',(59.9402651077865,252.442541339505,23.0245853614825)) ;
#105515=CARTESIAN_POINT('Origin',(58.9402651077865,248.040265107786,23.0213203435596)) ;
#105516=CARTESIAN_POINT('',(58.9402651077865,250.040265107786,23.0213203435596)) ;
#105517=CARTESIAN_POINT('Origin',(58.9402651077865,248.040265107786,23.0213203435596)) ;
#105518=CARTESIAN_POINT('Origin',(66.1902651077865,248.040265107786,23.0213203435596)) ;
#105519=CARTESIAN_POINT('',(66.1902651077865,250.040265107786,23.0213203435596)) ;
#105520=CARTESIAN_POINT('Origin',(66.1902651077865,248.040265107786,23.0213203435596)) ;
#105521=CARTESIAN_POINT('Ctrl Pts',(65.0766287441502,252.840884205283,23.0169129554328)) ;
#105522=CARTESIAN_POINT('Ctrl Pts',(65.0766287441502,252.841541153009,23.7324741241568)) ;
#105523=CARTESIAN_POINT('Ctrl Pts',(65.0766287441502,252.516901489192,25.1713430879785)) ;
#105524=CARTESIAN_POINT('Ctrl Pts',(65.0766287441502,251.136807428881,26.9009605060916)) ;
#105525=CARTESIAN_POINT('Ctrl Pts',(65.0766287441502,249.147758127707,27.8603793829806)) ;
#105526=CARTESIAN_POINT('Ctrl Pts',(65.0766287441502,246.937906934488,27.8621619194897)) ;
#105527=CARTESIAN_POINT('Ctrl Pts',(65.0766287441502,244.946768565938,26.9029449975024)) ;
#105528=CARTESIAN_POINT('Ctrl Pts',(65.0766287441502,243.567337531596,25.176962387584)) ;
#105529=CARTESIAN_POINT('Ctrl Pts',(65.0766287441502,243.076961974903,23.0176092156974)) ;
#105530=CARTESIAN_POINT('Ctrl Pts',(65.0766287441502,243.564201536425,20.8767992815642)) ;
#105531=CARTESIAN_POINT('Ctrl Pts',(65.0766287441502,244.934529934584,19.1484257862475)) ;
#105532=CARTESIAN_POINT('Ctrl Pts',(65.0766287441502,246.927745820604,18.1836492725528)) ;
#105533=CARTESIAN_POINT('Ctrl Pts',(65.0766287441502,249.136846465985,18.1816168623636)) ;
#105534=CARTESIAN_POINT('Ctrl Pts',(65.0766287441502,251.13038221688,19.1358824826931)) ;
#105535=CARTESIAN_POINT('Ctrl Pts',(65.0766287441502,252.511222282944,20.8659877742614)) ;
#105536=CARTESIAN_POINT('Ctrl Pts',(65.0766287441502,252.840227257557,22.3013517867086)) ;
#105537=CARTESIAN_POINT('Ctrl Pts',(65.0766287441502,252.840884205283,23.0169129554328)) ;
#105538=CARTESIAN_POINT('Ctrl Pts',(65.1748710205118,252.831915957252,23.0169211890687)) ;
#105539=CARTESIAN_POINT('Ctrl Pts',(65.1748710205118,252.832571765951,23.7312417059042)) ;
#105540=CARTESIAN_POINT('Ctrl Pts',(65.1748710205118,252.508661681794,25.1674922263976)) ;
#105541=CARTESIAN_POINT('Ctrl Pts',(65.1748710205118,251.131222805096,26.8940046369024)) ;
#105542=CARTESIAN_POINT('Ctrl Pts',(65.1748710205118,249.145626752009,27.851731242655)) ;
#105543=CARTESIAN_POINT('Ctrl Pts',(65.1748710205118,246.939810869674,27.8535478771211)) ;
#105544=CARTESIAN_POINT('Ctrl Pts',(65.1748710205118,244.952192187541,26.8960024422975)) ;
#105545=CARTESIAN_POINT('Ctrl Pts',(65.1748710205118,243.575204883934,25.173113845116)) ;
#105546=CARTESIAN_POINT('Ctrl Pts',(65.1748710205118,243.085737340501,23.0176042703897)) ;
#105547=CARTESIAN_POINT('Ctrl Pts',(65.1748710205118,243.572070300257,20.8805601134562)) ;
#105548=CARTESIAN_POINT('Ctrl Pts',(65.1748710205118,244.939993984156,19.1552952558752)) ;
#105549=CARTESIAN_POINT('Ctrl Pts',(65.1748710205118,246.929583107595,18.1921893326471)) ;
#105550=CARTESIAN_POINT('Ctrl Pts',(65.1748710205118,249.13471409468,18.1902224427852)) ;
#105551=CARTESIAN_POINT('Ctrl Pts',(65.1748710205118,251.124669629215,19.1427533342878)) ;
#105552=CARTESIAN_POINT('Ctrl Pts',(65.1748710205118,252.502921872703,20.869804047502)) ;
#105553=CARTESIAN_POINT('Ctrl Pts',(65.1748710205118,252.831260148553,22.3026006722331)) ;
#105554=CARTESIAN_POINT('Ctrl Pts',(65.1748710205118,252.831915957252,23.0169211890687)) ;
#105555=CARTESIAN_POINT('Ctrl Pts',(65.3636768956757,252.737773789869,23.0170076198108)) ;
#105556=CARTESIAN_POINT('Ctrl Pts',(65.3636768956757,252.738416598441,23.7171681269576)) ;
#105557=CARTESIAN_POINT('Ctrl Pts',(65.3636768956757,252.420709470249,25.1251094967809)) ;
#105558=CARTESIAN_POINT('Ctrl Pts',(65.3636768956758,251.070232680745,26.8175359526613)) ;
#105559=CARTESIAN_POINT('Ctrl Pts',(65.3636768956757,249.12399117821,27.7563151648642)) ;
#105560=CARTESIAN_POINT('Ctrl Pts',(65.3636768956758,246.961634836841,27.7580471751047)) ;
#105561=CARTESIAN_POINT('Ctrl Pts',(65.3636768956758,245.013328686296,26.8194722536279)) ;
#105562=CARTESIAN_POINT('Ctrl Pts',(65.3636768956758,243.663569427515,25.1306039104643)) ;
#105563=CARTESIAN_POINT('Ctrl Pts',(65.3636768956758,243.183729076732,23.0176928098972)) ;
#105564=CARTESIAN_POINT('Ctrl Pts',(65.3636768956758,243.660502243309,20.9229407854373)) ;
#105565=CARTESIAN_POINT('Ctrl Pts',(65.3636768956758,245.001347179161,19.2317295875749)) ;
#105566=CARTESIAN_POINT('Ctrl Pts',(65.3636768956758,246.951719972586,18.2877181762278)) ;
#105567=CARTESIAN_POINT('Ctrl Pts',(65.3636768956758,249.113320875214,18.2857092340863)) ;
#105568=CARTESIAN_POINT('Ctrl Pts',(65.3636768956758,251.063991246017,19.2194629073674)) ;
#105569=CARTESIAN_POINT('Ctrl Pts',(65.3636768956758,252.415175533547,20.9123499681276)) ;
#105570=CARTESIAN_POINT('Ctrl Pts',(65.3636768956758,252.737130981298,22.3168471126638)) ;
#105571=CARTESIAN_POINT('Ctrl Pts',(65.3636768956758,252.737773789869,23.0170076198108)) ;
#105572=CARTESIAN_POINT('Ctrl Pts',(65.4402651077865,252.541191423318,23.0171880996136)) ;
#105573=CARTESIAN_POINT('Ctrl Pts',(65.4402651077865,252.54180737839,23.6880992141914)) ;
#105574=CARTESIAN_POINT('Ctrl Pts',(65.4402651077865,252.237461144507,25.0371577162623)) ;
#105575=CARTESIAN_POINT('Ctrl Pts',(65.4402651077866,250.943540302405,26.6588261848968)) ;
#105576=CARTESIAN_POINT('Ctrl Pts',(65.4402651077865,249.078606004666,27.558372331764)) ;
#105577=CARTESIAN_POINT('Ctrl Pts',(65.4402651077866,247.006690998239,27.5600517492951)) ;
#105578=CARTESIAN_POINT('Ctrl Pts',(65.4402651077866,245.139811685101,26.6606905000547)) ;
#105579=CARTESIAN_POINT('Ctrl Pts',(65.4402651077866,243.846466640749,25.042429009221)) ;
#105580=CARTESIAN_POINT('Ctrl Pts',(65.4402651077866,243.386702460434,23.0178383037529)) ;
#105581=CARTESIAN_POINT('Ctrl Pts',(65.4402651077866,243.843525449649,21.0106238048176)) ;
#105582=CARTESIAN_POINT('Ctrl Pts',(65.4402651077866,245.128340916242,19.3901229016862)) ;
#105583=CARTESIAN_POINT('Ctrl Pts',(65.4402651077866,246.997145550192,18.485546674421)) ;
#105584=CARTESIAN_POINT('Ctrl Pts',(65.4402651077866,249.068370873645,18.4836546021279)) ;
#105585=CARTESIAN_POINT('Ctrl Pts',(65.4402651077865,250.937485683585,19.3783578426627)) ;
#105586=CARTESIAN_POINT('Ctrl Pts',(65.4402651077866,252.23212095168,21.0004949225647)) ;
#105587=CARTESIAN_POINT('Ctrl Pts',(65.4402651077866,252.540575468246,22.3462769850356)) ;
#105588=CARTESIAN_POINT('Ctrl Pts',(65.4402651077866,252.541191423318,23.0171880996136)) ;
#105589=CARTESIAN_POINT('Ctrl Pts',(65.4402651077865,252.442540694976,23.0172786696089)) ;
#105590=CARTESIAN_POINT('Ctrl Pts',(65.4402651077865,252.443143130803,23.6734643407148)) ;
#105591=CARTESIAN_POINT('Ctrl Pts',(65.4402651077865,252.145441264101,24.9929395133859)) ;
#105592=CARTESIAN_POINT('Ctrl Pts',(65.4402651077866,250.87986399868,26.5790375520551)) ;
#105593=CARTESIAN_POINT('Ctrl Pts',(65.4402651077865,249.055861093547,27.4588462212786)) ;
#105594=CARTESIAN_POINT('Ctrl Pts',(65.4402651077866,247.029377891764,27.4604808473129)) ;
#105595=CARTESIAN_POINT('Ctrl Pts',(65.4402651077866,245.203459264903,26.5808573752723)) ;
#105596=CARTESIAN_POINT('Ctrl Pts',(65.4402651077866,243.938490009196,24.9980925373954)) ;
#105597=CARTESIAN_POINT('Ctrl Pts',(65.4402651077866,243.488804604471,23.0179171559172)) ;
#105598=CARTESIAN_POINT('Ctrl Pts',(65.4402651077866,243.935614231154,21.0547463401441)) ;
#105599=CARTESIAN_POINT('Ctrl Pts',(65.4402651077866,245.192236164937,19.4697890066313)) ;
#105600=CARTESIAN_POINT('Ctrl Pts',(65.4402651077866,247.020059922002,18.5850672640655)) ;
#105601=CARTESIAN_POINT('Ctrl Pts',(65.4402651077866,249.045854854551,18.5832034982517)) ;
#105602=CARTESIAN_POINT('Ctrl Pts',(65.4402651077865,250.873971934894,19.4582865154112)) ;
#105603=CARTESIAN_POINT('Ctrl Pts',(65.4402651077866,252.140233304353,21.0448319450019)) ;
#105604=CARTESIAN_POINT('Ctrl Pts',(65.4402651077866,252.44193825915,22.3610929985028)) ;
#105605=CARTESIAN_POINT('Ctrl Pts',(65.4402651077866,252.442540694976,23.0172786696089)) ;
#105606=CARTESIAN_POINT('',(65.0766287441502,252.840884205283,23.0169129554328)) ;
#105607=CARTESIAN_POINT('Ctrl Pts',(65.4402651077865,252.442540694976,23.0172786696089)) ;
#105608=CARTESIAN_POINT('Ctrl Pts',(65.4402651077865,252.541191423318,23.0171880996136)) ;
#105609=CARTESIAN_POINT('Ctrl Pts',(65.3636768956757,252.737773789869,23.0170076198108)) ;
#105610=CARTESIAN_POINT('Ctrl Pts',(65.1748710205118,252.831915957252,23.0169211890687)) ;
#105611=CARTESIAN_POINT('Ctrl Pts',(65.0766287441502,252.840884205283,23.0169129554328)) ;
#105612=CARTESIAN_POINT('',(65.0766287441502,248.040357057742,27.8212999984394)) ;
#105613=CARTESIAN_POINT('Ctrl Pts',(65.0766287441502,252.840884205283,23.0169129554328)) ;
#105614=CARTESIAN_POINT('Ctrl Pts',(65.0766287441502,252.841541153009,23.7324741241568)) ;
#105615=CARTESIAN_POINT('Ctrl Pts',(65.0766287441502,252.516901489192,25.1713430879785)) ;
#105616=CARTESIAN_POINT('Ctrl Pts',(65.0766287441502,251.136807428881,26.9009605060916)) ;
#105617=CARTESIAN_POINT('Ctrl Pts',(65.0766287441502,249.478518089747,27.700837157902)) ;
#105618=CARTESIAN_POINT('Ctrl Pts',(65.0766287441502,248.400319833693,27.8212533107379)) ;
#105619=CARTESIAN_POINT('Ctrl Pts',(65.0766287441502,248.040357057742,27.8212999984394)) ;
#105620=CARTESIAN_POINT('Ctrl Pts',(65.0766287441502,248.040357057742,27.8212999984394)) ;
#105621=CARTESIAN_POINT('Ctrl Pts',(65.0766287441502,247.682015582841,27.8213464758557)) ;
#105622=CARTESIAN_POINT('Ctrl Pts',(65.0766287441502,246.605301499027,27.7019315873951)) ;
#105623=CARTESIAN_POINT('Ctrl Pts',(65.0766287441502,244.946768565938,26.9029449975024)) ;
#105624=CARTESIAN_POINT('Ctrl Pts',(65.0766287441502,243.567337531596,25.176962387584)) ;
#105625=CARTESIAN_POINT('Ctrl Pts',(65.0766287441502,243.076961974903,23.0176092156974)) ;
#105626=CARTESIAN_POINT('Ctrl Pts',(65.0766287441502,243.564201536425,20.8767992815642)) ;
#105627=CARTESIAN_POINT('Ctrl Pts',(65.0766287441502,244.934529934584,19.1484257862475)) ;
#105628=CARTESIAN_POINT('Ctrl Pts',(65.0766287441502,246.927745820604,18.1836492725528)) ;
#105629=CARTESIAN_POINT('Ctrl Pts',(65.0766287441502,249.136846465985,18.1816168623636)) ;
#105630=CARTESIAN_POINT('Ctrl Pts',(65.0766287441502,251.13038221688,19.1358824826931)) ;
#105631=CARTESIAN_POINT('Ctrl Pts',(65.0766287441502,252.511222282944,20.8659877742614)) ;
#105632=CARTESIAN_POINT('Ctrl Pts',(65.0766287441502,252.840227257557,22.3013517867086)) ;
#105633=CARTESIAN_POINT('Ctrl Pts',(65.0766287441502,252.840884205283,23.0169129554328)) ;
#105634=CARTESIAN_POINT('Ctrl Pts',(60.3039014714229,252.840884908133,23.0248807993021)) ;
#105635=CARTESIAN_POINT('Ctrl Pts',(60.3039014714229,252.841415615489,22.3093195258141)) ;
#105636=CARTESIAN_POINT('Ctrl Pts',(60.3039014714229,252.516523675061,20.8705067056309)) ;
#105637=CARTESIAN_POINT('Ctrl Pts',(60.3039014714229,251.136126602205,19.141131868271)) ;
#105638=CARTESIAN_POINT('Ctrl Pts',(60.3039014714229,249.146908371569,18.1820636614743)) ;
#105639=CARTESIAN_POINT('Ctrl Pts',(60.3039014714228,246.937055020249,18.180670321379)) ;
#105640=CARTESIAN_POINT('Ctrl Pts',(60.3039014714228,244.946085396763,19.1402381324422)) ;
#105641=CARTESIAN_POINT('Ctrl Pts',(60.3039014714229,243.566959144073,20.8664652922218)) ;
#105642=CARTESIAN_POINT('Ctrl Pts',(60.3039014714228,243.076964984333,23.02590555023)) ;
#105643=CARTESIAN_POINT('Ctrl Pts',(60.3039014714229,243.564583507187,25.1666326084264)) ;
#105644=CARTESIAN_POINT('Ctrl Pts',(60.3039014714229,244.935220605921,26.8947713028763)) ;
#105645=CARTESIAN_POINT('Ctrl Pts',(60.3039014714229,246.928604395157,27.859194804961)) ;
#105646=CARTESIAN_POINT('Ctrl Pts',(60.3039014714229,249.137705727497,27.8608402304461)) ;
#105647=CARTESIAN_POINT('Ctrl Pts',(60.3039014714229,251.131070962159,26.9062196225889)) ;
#105648=CARTESIAN_POINT('Ctrl Pts',(60.3039014714229,252.511603475512,25.175871101808)) ;
#105649=CARTESIAN_POINT('Ctrl Pts',(60.3039014714229,252.840354200776,23.7404420727902)) ;
#105650=CARTESIAN_POINT('Ctrl Pts',(60.3039014714229,252.840884908133,23.0248807993021)) ;
#105651=CARTESIAN_POINT('Ctrl Pts',(60.2056591950613,252.831916658789,23.0248741478579)) ;
#105652=CARTESIAN_POINT('Ctrl Pts',(60.2056591950613,252.832446445996,22.31055352644)) ;
#105653=CARTESIAN_POINT('Ctrl Pts',(60.2056591950613,252.508284848399,20.8743600638376)) ;
#105654=CARTESIAN_POINT('Ctrl Pts',(60.2056591950612,251.130544493213,19.1480906302711)) ;
#105655=CARTESIAN_POINT('Ctrl Pts',(60.2056591950613,249.144779759817,18.1907143485154)) ;
#105656=CARTESIAN_POINT('Ctrl Pts',(60.2056591950612,246.938963013392,18.1892858361865)) ;
#105657=CARTESIAN_POINT('Ctrl Pts',(60.2056591950612,244.951513228265,19.1471814493788)) ;
#105658=CARTESIAN_POINT('Ctrl Pts',(60.2056591950613,243.574830611665,20.8703131984953)) ;
#105659=CARTESIAN_POINT('Ctrl Pts',(60.2056591950613,243.085744226675,23.0259087382533)) ;
#105660=CARTESIAN_POINT('Ctrl Pts',(60.2056591950613,243.572455132768,25.1628696592994)) ;
#105661=CARTESIAN_POINT('Ctrl Pts',(60.2056591950613,244.940686770073,26.8878990509792)) ;
#105662=CARTESIAN_POINT('Ctrl Pts',(60.2056591950613,246.9304425947,27.8506526804878)) ;
#105663=CARTESIAN_POINT('Ctrl Pts',(60.2056591950613,249.135573431834,27.8522327343816)) ;
#105664=CARTESIAN_POINT('Ctrl Pts',(60.2056591950613,251.125358278647,26.8993483215869)) ;
#105665=CARTESIAN_POINT('Ctrl Pts',(60.2056591950613,252.503302661219,25.1720554371834)) ;
#105666=CARTESIAN_POINT('Ctrl Pts',(60.2056591950613,252.831386871581,23.7391947692758)) ;
#105667=CARTESIAN_POINT('Ctrl Pts',(60.2056591950613,252.831916658789,23.0248741478579)) ;
#105668=CARTESIAN_POINT('Ctrl Pts',(60.0168530828095,252.737774694053,23.024804325978)) ;
#105669=CARTESIAN_POINT('Ctrl Pts',(60.0168530828095,252.738293979264,22.3246437163219)) ;
#105670=CARTESIAN_POINT('Ctrl Pts',(60.0168530828095,252.420339841483,20.9167569091084)) ;
#105671=CARTESIAN_POINT('Ctrl Pts',(60.0168530828094,251.069566142761,19.2245675100239)) ;
#105672=CARTESIAN_POINT('Ctrl Pts',(60.0168530828095,249.123159359322,18.2861313252103)) ;
#105673=CARTESIAN_POINT('Ctrl Pts',(60.0168530828094,246.960800415503,18.2847802781622)) ;
#105674=CARTESIAN_POINT('Ctrl Pts',(60.0168530828094,245.012659210062,19.2236985730182)) ;
#105675=CARTESIAN_POINT('Ctrl Pts',(60.0168530828094,243.663198013795,20.9128065556026)) ;
#105676=CARTESIAN_POINT('Ctrl Pts',(60.0168530828094,243.18373069356,23.0258032190076)) ;
#105677=CARTESIAN_POINT('Ctrl Pts',(60.0168530828094,243.660874803201,25.1204743342267)) ;
#105678=CARTESIAN_POINT('Ctrl Pts',(60.0168530828094,245.002021874673,26.8114561732744)) ;
#105679=CARTESIAN_POINT('Ctrl Pts',(60.0168530828095,246.952559313171,27.7551221353331)) ;
#105680=CARTESIAN_POINT('Ctrl Pts',(60.0168530828094,249.114161208371,27.7567526134108)) ;
#105681=CARTESIAN_POINT('Ctrl Pts',(60.0168530828094,251.064664927345,26.8226512873956)) ;
#105682=CARTESIAN_POINT('Ctrl Pts',(60.0168530828095,252.415548621932,25.1295260055957)) ;
#105683=CARTESIAN_POINT('Ctrl Pts',(60.0168530828095,252.737255408843,23.7249649356341)) ;
#105684=CARTESIAN_POINT('Ctrl Pts',(60.0168530828095,252.737774694053,23.024804325978)) ;
#105685=CARTESIAN_POINT('Ctrl Pts',(59.9402651077865,252.54119208229,23.0246585273691)) ;
#105686=CARTESIAN_POINT('Ctrl Pts',(59.9402651077865,252.541689674222,22.3537473145644)) ;
#105687=CARTESIAN_POINT('Ctrl Pts',(59.9402651077865,252.237106976482,21.0047416734212)) ;
#105688=CARTESIAN_POINT('Ctrl Pts',(59.9402651077865,250.942902249354,19.3833008269238)) ;
#105689=CARTESIAN_POINT('Ctrl Pts',(59.9402651077865,249.077809553585,18.4840835259144)) ;
#105690=CARTESIAN_POINT('Ctrl Pts',(59.9402651077865,247.005892805063,18.4827689323583)) ;
#105691=CARTESIAN_POINT('Ctrl Pts',(59.9402651077865,245.139171804449,19.3824591533555)) ;
#105692=CARTESIAN_POINT('Ctrl Pts',(59.9402651077865,243.84611261837,21.000949722106)) ;
#105693=CARTESIAN_POINT('Ctrl Pts',(59.9402651077865,243.386706128535,23.0256218681107)) ;
#105694=CARTESIAN_POINT('Ctrl Pts',(59.9402651077865,243.843884354356,25.0327585526377)) ;
#105695=CARTESIAN_POINT('Ctrl Pts',(59.9402651077865,245.12898921281,26.6530390723829)) ;
#105696=CARTESIAN_POINT('Ctrl Pts',(59.9402651077865,246.997951074417,27.5572843385644)) ;
#105697=CARTESIAN_POINT('Ctrl Pts',(59.9402651077865,249.069176859737,27.558813459608)) ;
#105698=CARTESIAN_POINT('Ctrl Pts',(59.9402651077865,250.938131691571,26.6637775677947)) ;
#105699=CARTESIAN_POINT('Ctrl Pts',(59.9402651077865,252.232478414354,25.0414125746018)) ;
#105700=CARTESIAN_POINT('Ctrl Pts',(59.9402651077865,252.540694490358,23.6955697401738)) ;
#105701=CARTESIAN_POINT('Ctrl Pts',(59.9402651077865,252.54119208229,23.0246585273691)) ;
#105702=CARTESIAN_POINT('Ctrl Pts',(59.9402651077865,252.442541339505,23.0245853614825)) ;
#105703=CARTESIAN_POINT('Ctrl Pts',(59.9402651077865,252.443028010077,22.3683995943057)) ;
#105704=CARTESIAN_POINT('Ctrl Pts',(59.9402651077865,252.145094800052,21.0489759066127)) ;
#105705=CARTESIAN_POINT('Ctrl Pts',(59.9402651077865,250.87923966532,19.4631003199451)) ;
#105706=CARTESIAN_POINT('Ctrl Pts',(59.9402651077865,249.055081848073,18.5836132230762)) ;
#105707=CARTESIAN_POINT('Ctrl Pts',(59.9402651077865,247.028596667264,18.582335498899)) ;
#105708=CARTESIAN_POINT('Ctrl Pts',(59.9402651077865,245.202832783418,19.462280744107)) ;
#105709=CARTESIAN_POINT('Ctrl Pts',(59.9402651077865,243.938143019334,21.0452698397019)) ;
#105710=CARTESIAN_POINT('Ctrl Pts',(59.9402651077865,243.488807364186,23.0255250811106)) ;
#105711=CARTESIAN_POINT('Ctrl Pts',(59.9402651077865,243.935964506927,24.9886198977872)) ;
#105712=CARTESIAN_POINT('Ctrl Pts',(59.9402651077865,245.192869526073,26.5733619136289)) ;
#105713=CARTESIAN_POINT('Ctrl Pts',(59.9402651077865,247.02084725416,27.457759936616)) ;
#105714=CARTESIAN_POINT('Ctrl Pts',(59.9402651077865,249.046642816666,27.4592688287601)) ;
#105715=CARTESIAN_POINT('Ctrl Pts',(59.9402651077865,250.874603529792,26.5838602800608)) ;
#105716=CARTESIAN_POINT('Ctrl Pts',(59.9402651077865,252.140582866504,24.9970918038166)) ;
#105717=CARTESIAN_POINT('Ctrl Pts',(59.9402651077865,252.442054668933,23.6807711286595)) ;
#105718=CARTESIAN_POINT('Ctrl Pts',(59.9402651077865,252.442541339505,23.0245853614825)) ;
#105719=CARTESIAN_POINT('',(60.3039014714229,252.840884908133,23.0248807993021)) ;
#105720=CARTESIAN_POINT('Ctrl Pts',(59.9402651077865,252.442541339505,23.0245853614825)) ;
#105721=CARTESIAN_POINT('Ctrl Pts',(59.9402651077865,252.54119208229,23.0246585273691)) ;
#105722=CARTESIAN_POINT('Ctrl Pts',(60.0168530828095,252.737774694053,23.024804325978)) ;
#105723=CARTESIAN_POINT('Ctrl Pts',(60.2056591950613,252.831916658789,23.0248741478579)) ;
#105724=CARTESIAN_POINT('Ctrl Pts',(60.3039014714229,252.840884908133,23.0248807993021)) ;
#105725=CARTESIAN_POINT('',(60.3039014714229,248.040364444053,18.2213381124782)) ;
#105726=CARTESIAN_POINT('Ctrl Pts',(60.3039014714229,252.840884908133,23.0248807993021)) ;
#105727=CARTESIAN_POINT('Ctrl Pts',(60.3039014714229,252.841415615489,22.3093195258141)) ;
#105728=CARTESIAN_POINT('Ctrl Pts',(60.3039014714229,252.516523675061,20.8705067056309)) ;
#105729=CARTESIAN_POINT('Ctrl Pts',(60.3039014714229,251.136126602205,19.141131868271)) ;
#105730=CARTESIAN_POINT('Ctrl Pts',(60.3039014714229,249.477958337868,18.3416738503658)) ;
#105731=CARTESIAN_POINT('Ctrl Pts',(60.3039014714229,248.400043702177,18.2213846529397)) ;
#105732=CARTESIAN_POINT('Ctrl Pts',(60.3039014714229,248.040364444053,18.2213381124782)) ;
#105733=CARTESIAN_POINT('Ctrl Pts',(60.3039014714229,248.040364444053,18.2213381124782)) ;
#105734=CARTESIAN_POINT('Ctrl Pts',(60.3039014714229,247.681739029051,18.2212917083782)) ;
#105735=CARTESIAN_POINT('Ctrl Pts',(60.3039014714228,246.604739915942,18.3408329242945)) ;
#105736=CARTESIAN_POINT('Ctrl Pts',(60.3039014714228,244.946085396763,19.1402381324422)) ;
#105737=CARTESIAN_POINT('Ctrl Pts',(60.3039014714229,243.566959144073,20.8664652922218)) ;
#105738=CARTESIAN_POINT('Ctrl Pts',(60.3039014714228,243.076964984333,23.02590555023)) ;
#105739=CARTESIAN_POINT('Ctrl Pts',(60.3039014714229,243.564583507187,25.1666326084264)) ;
#105740=CARTESIAN_POINT('Ctrl Pts',(60.3039014714229,244.935220605921,26.8947713028763)) ;
#105741=CARTESIAN_POINT('Ctrl Pts',(60.3039014714229,246.928604395157,27.859194804961)) ;
#105742=CARTESIAN_POINT('Ctrl Pts',(60.3039014714229,249.137705727497,27.8608402304461)) ;
#105743=CARTESIAN_POINT('Ctrl Pts',(60.3039014714229,251.131070962159,26.9062196225889)) ;
#105744=CARTESIAN_POINT('Ctrl Pts',(60.3039014714229,252.511603475512,25.175871101808)) ;
#105745=CARTESIAN_POINT('Ctrl Pts',(60.3039014714229,252.840354200776,23.7404420727902)) ;
#105746=CARTESIAN_POINT('Ctrl Pts',(60.3039014714229,252.840884908133,23.0248807993021)) ;
#105747=CARTESIAN_POINT('Origin',(64.7902651077865,248.040265107786,23.0213203435596)) ;
#105748=CARTESIAN_POINT('',(64.9402651077865,246.182069881617,27.6093057948708)) ;
#105749=CARTESIAN_POINT('',(64.9402651077865,245.420726657552,27.2213820464094)) ;
#105750=CARTESIAN_POINT('Origin',(64.9402651077865,248.040265107786,23.0213203435596)) ;
#105751=CARTESIAN_POINT('',(64.7902651077865,245.996818189747,27.694041680549)) ;
#105752=CARTESIAN_POINT('Ctrl Pts',(64.9402651077865,246.182069881617,27.6093057948708)) ;
#105753=CARTESIAN_POINT('Ctrl Pts',(64.9402651077865,246.181354905733,27.6096388244826)) ;
#105754=CARTESIAN_POINT('Ctrl Pts',(64.940261777681,246.180639897624,27.6099717982194)) ;
#105755=CARTESIAN_POINT('Ctrl Pts',(64.9400834366345,246.161498924883,27.6188837045809)) ;
#105756=CARTESIAN_POINT('Ctrl Pts',(64.9376982652988,246.142984930219,27.6274555764536)) ;
#105757=CARTESIAN_POINT('Ctrl Pts',(64.9285249168183,246.107849325612,27.6436380121775)) ;
#105758=CARTESIAN_POINT('Ctrl Pts',(64.9218878905886,246.091024885902,27.6513456347974)) ;
#105759=CARTESIAN_POINT('Ctrl Pts',(64.9030518920066,246.057970599548,27.6664219076507)) ;
#105760=CARTESIAN_POINT('Ctrl Pts',(64.8902415596279,246.04185831974,27.6737287158086)) ;
#105761=CARTESIAN_POINT('Ctrl Pts',(64.8622234505159,246.018444687196,27.6843112161272)) ;
#105762=CARTESIAN_POINT('Ctrl Pts',(64.8483068832618,246.010067315225,27.6880838741351)) ;
#105763=CARTESIAN_POINT('Ctrl Pts',(64.8193104176513,245.999468779803,27.6928518010587)) ;
#105764=CARTESIAN_POINT('Ctrl Pts',(64.8049443310403,245.996818189747,27.694041680549)) ;
#105765=CARTESIAN_POINT('Ctrl Pts',(64.7902651077865,245.996818189747,27.694041680549)) ;
#105766=CARTESIAN_POINT('',(64.7902651077865,245.461062098449,27.4210603173112)) ;
#105767=CARTESIAN_POINT('Origin',(64.7902651077865,248.040265107786,23.0213203435596)) ;
#105768=CARTESIAN_POINT('Ctrl Pts',(64.9402651077865,245.420726657552,27.2213820464094)) ;
#105769=CARTESIAN_POINT('Ctrl Pts',(64.9402651077865,245.420877483218,27.2221562239469)) ;
#105770=CARTESIAN_POINT('Ctrl Pts',(64.9402617776811,245.421028373027,27.2229303947064)) ;
#105771=CARTESIAN_POINT('Ctrl Pts',(64.9400834366345,245.425069270822,27.2436540540753)) ;
#105772=CARTESIAN_POINT('Ctrl Pts',(64.9376982652987,245.429016733827,27.2636706102621)) ;
#105773=CARTESIAN_POINT('Ctrl Pts',(64.9285249168183,245.436577058534,27.3016077085614)) ;
#105774=CARTESIAN_POINT('Ctrl Pts',(64.9218878905886,245.440230618388,27.3197493931139)) ;
#105775=CARTESIAN_POINT('Ctrl Pts',(64.9030518920066,245.447462479482,27.3553524833539)) ;
#105776=CARTESIAN_POINT('Ctrl Pts',(64.8902415596279,245.451021707959,27.372682425613)) ;
#105777=CARTESIAN_POINT('Ctrl Pts',(64.8622234505159,245.45622247327,27.3978446898608)) ;
#105778=CARTESIAN_POINT('Ctrl Pts',(64.8483068832618,245.458094424526,27.406839638893)) ;
#105779=CARTESIAN_POINT('Ctrl Pts',(64.8193104176514,245.460466753434,27.4182165512944)) ;
#105780=CARTESIAN_POINT('Ctrl Pts',(64.8049443310403,245.461062098449,27.4210603173112)) ;
#105781=CARTESIAN_POINT('Ctrl Pts',(64.7902651077865,245.461062098449,27.4210603173112)) ;
#105782=CARTESIAN_POINT('Origin',(64.7902651077865,246.861601651513,25.5179220536754)) ;
#105783=CARTESIAN_POINT('',(64.9402651077865,246.014168667474,28.1260525975113)) ;
#105784=CARTESIAN_POINT('',(64.9402651077865,246.861601651513,25.5179220536754)) ;
#105785=CARTESIAN_POINT('',(64.7902651077865,245.872657996292,28.0761674639184)) ;
#105786=CARTESIAN_POINT('Ctrl Pts',(64.9402651077865,246.014168667474,28.1260525975113)) ;
#105787=CARTESIAN_POINT('Ctrl Pts',(64.9402651077865,246.012794157307,28.1255643186931)) ;
#105788=CARTESIAN_POINT('Ctrl Pts',(64.940243846551,246.011419678562,28.1250761825186)) ;
#105789=CARTESIAN_POINT('Ctrl Pts',(64.9402013305492,246.010045670283,28.1245883423369)) ;
#105790=CARTESIAN_POINT('Ctrl Pts',(64.939655139511,245.992394174936,28.1183211976405)) ;
#105791=CARTESIAN_POINT('Ctrl Pts',(64.9356062703199,245.97498719514,28.1121625030257)) ;
#105792=CARTESIAN_POINT('Ctrl Pts',(64.928263675975,245.958729638151,28.1064243414529)) ;
#105793=CARTESIAN_POINT('Ctrl Pts',(64.9206090302591,245.94178115467,28.1004423149597)) ;
#105794=CARTESIAN_POINT('Ctrl Pts',(64.9095180038061,245.926399208258,28.095028961218)) ;
#105795=CARTESIAN_POINT('Ctrl Pts',(64.8956136387304,245.913453339836,28.0904794283363)) ;
#105796=CARTESIAN_POINT('Ctrl Pts',(64.8817129938792,245.900510935184,28.0859311127188)) ;
#105797=CARTESIAN_POINT('Ctrl Pts',(64.8652664191736,245.890251001563,28.0823329269323)) ;
#105798=CARTESIAN_POINT('Ctrl Pts',(64.8471986491033,245.883254040199,28.0798802263625)) ;
#105799=CARTESIAN_POINT('Ctrl Pts',(64.8291331055125,245.876257941067,28.0774278280374)) ;
#105800=CARTESIAN_POINT('Ctrl Pts',(64.8097925816883,245.872657996292,28.0761674639184)) ;
#105801=CARTESIAN_POINT('Ctrl Pts',(64.7902651077865,245.872657996292,28.0761674639184)) ;
#105802=CARTESIAN_POINT('',(64.7902651077865,246.718943174069,25.4715695045192)) ;
#105803=CARTESIAN_POINT('Origin',(64.7902651077865,246.340671638724,28.252131183183)) ;
#105804=CARTESIAN_POINT('',(64.9402651077865,246.678925224467,28.3420450960781)) ;
#105805=CARTESIAN_POINT('Origin',(64.9402651077865,246.340671638724,28.252131183183)) ;
#105806=CARTESIAN_POINT('',(64.7902651077865,246.822731508173,28.3848650607978)) ;
#105807=CARTESIAN_POINT('Ctrl Pts',(64.9402651077865,246.678925224469,28.3420450960789)) ;
#105808=CARTESIAN_POINT('Ctrl Pts',(64.9402651077865,246.680324229641,28.3424579870221)) ;
#105809=CARTESIAN_POINT('Ctrl Pts',(64.9402438465509,246.681723125548,28.3428709748967)) ;
#105810=CARTESIAN_POINT('Ctrl Pts',(64.9402013305491,246.683121466859,28.343283925702)) ;
#105811=CARTESIAN_POINT('Ctrl Pts',(64.9396551395109,246.701085561798,28.3485889877857)) ;
#105812=CARTESIAN_POINT('Ctrl Pts',(64.9356062703199,246.718788094141,28.3538380651884)) ;
#105813=CARTESIAN_POINT('Ctrl Pts',(64.9282636759749,246.73531354078,28.3587517471959)) ;
#105814=CARTESIAN_POINT('Ctrl Pts',(64.920609030259,246.752541298897,28.3638742547404)) ;
#105815=CARTESIAN_POINT('Ctrl Pts',(64.9095180038064,246.768167444445,28.3685360408182)) ;
#105816=CARTESIAN_POINT('Ctrl Pts',(64.8956136387306,246.781315020339,28.3724647819376)) ;
#105817=CARTESIAN_POINT('Ctrl Pts',(64.8817129938792,246.794459078493,28.3763924718907)) ;
#105818=CARTESIAN_POINT('Ctrl Pts',(64.8652664191735,246.804874499694,28.3795121161122)) ;
#105819=CARTESIAN_POINT('Ctrl Pts',(64.8471986491031,246.811976821569,28.3816405503697)) ;
#105820=CARTESIAN_POINT('Ctrl Pts',(64.8291331055123,246.81907826823,28.3837687223415)) ;
#105821=CARTESIAN_POINT('Ctrl Pts',(64.8097925816884,246.822731508174,28.3848650607972)) ;
#105822=CARTESIAN_POINT('Ctrl Pts',(64.7902651077865,246.822731508174,28.3848650607972)) ;
#105823=CARTESIAN_POINT('Origin',(64.7902651077865,246.340671638724,28.252131183183)) ;
#105824=CARTESIAN_POINT('Origin',(64.7902651077865,247.635028874288,25.3994606331908)) ;
#105825=CARTESIAN_POINT('',(64.9402651077865,246.84682643861,27.8252982934377)) ;
#105826=CARTESIAN_POINT('',(64.9402651077865,247.635028874288,25.3994606331908)) ;
#105827=CARTESIAN_POINT('',(64.7902651077865,246.946891701628,28.0027392774284)) ;
#105828=CARTESIAN_POINT('Ctrl Pts',(64.9402651077865,246.84682643861,27.8252982934377)) ;
#105829=CARTESIAN_POINT('Ctrl Pts',(64.9402651077865,246.847209116357,27.8259879723329)) ;
#105830=CARTESIAN_POINT('Ctrl Pts',(64.940261777681,246.847591853015,27.8266776249647)) ;
#105831=CARTESIAN_POINT('Ctrl Pts',(64.9400834366348,246.857838938123,27.8451382901555)) ;
#105832=CARTESIAN_POINT('Ctrl Pts',(64.9376982652992,246.867778654567,27.8629553331985)) ;
#105833=CARTESIAN_POINT('Ctrl Pts',(64.9285249168188,246.886692158738,27.896699388929)) ;
#105834=CARTESIAN_POINT('Ctrl Pts',(64.921887890589,246.895772989479,27.9128241441551)) ;
#105835=CARTESIAN_POINT('Ctrl Pts',(64.9030518920066,246.913652858034,27.9444499271496)) ;
#105836=CARTESIAN_POINT('Ctrl Pts',(64.890241559628,246.92239313214,27.9598318195758)) ;
#105837=CARTESIAN_POINT('Ctrl Pts',(64.8622234505159,246.935114921148,27.9821554300886)) ;
#105838=CARTESIAN_POINT('Ctrl Pts',(64.8483068832618,246.939674844702,27.9901316702288)) ;
#105839=CARTESIAN_POINT('Ctrl Pts',(64.8193104176513,246.945446722844,28.0002186669547)) ;
#105840=CARTESIAN_POINT('Ctrl Pts',(64.8049443310403,246.946891701628,28.0027392774284)) ;
#105841=CARTESIAN_POINT('Ctrl Pts',(64.7902651077865,246.946891701628,28.0027392774284)) ;
#105842=CARTESIAN_POINT('',(64.7902651077865,247.777687351732,25.445813182347)) ;
#105843=CARTESIAN_POINT('Origin',(64.7902651077865,248.040265107786,23.0213203435596)) ;
#105844=CARTESIAN_POINT('',(64.9402651077865,247.69078190379,27.9589677074491)) ;
#105845=CARTESIAN_POINT('Origin',(64.9402651077865,248.040265107786,23.0213203435596)) ;
#105846=CARTESIAN_POINT('',(64.7902651077865,247.54078190379,28.096802244712)) ;
#105847=CARTESIAN_POINT('Ctrl Pts',(64.9402651077865,247.69078190379,27.9589677074491)) ;
#105848=CARTESIAN_POINT('Ctrl Pts',(64.9402651077865,247.690204833126,27.9595053771295)) ;
#105849=CARTESIAN_POINT('Ctrl Pts',(64.940261777681,247.68962771455,27.9600430036272)) ;
#105850=CARTESIAN_POINT('Ctrl Pts',(64.9400834366348,247.674177498214,27.9744336161108)) ;
#105851=CARTESIAN_POINT('Ctrl Pts',(64.9376982652992,247.659218497029,27.9883070896973)) ;
#105852=CARTESIAN_POINT('Ctrl Pts',(64.9285249168187,247.630803198961,28.0145549995742)) ;
#105853=CARTESIAN_POINT('Ctrl Pts',(64.9218878905889,247.617183992317,28.0270844220837)) ;
#105854=CARTESIAN_POINT('Ctrl Pts',(64.9030518920067,247.590406322412,28.0516371458428)) ;
#105855=CARTESIAN_POINT('Ctrl Pts',(64.890241559628,247.577340561604,28.0635653016335)) ;
#105856=CARTESIAN_POINT('Ctrl Pts',(64.8622234505159,247.558343046244,28.0808650678764)) ;
#105857=CARTESIAN_POINT('Ctrl Pts',(64.8483068832618,247.55154150748,28.087041829166)) ;
#105858=CARTESIAN_POINT('Ctrl Pts',(64.8193104176513,247.542935071751,28.0948515246968)) ;
#105859=CARTESIAN_POINT('Ctrl Pts',(64.8049443310403,247.54078190379,28.096802244712)) ;
#105860=CARTESIAN_POINT('Ctrl Pts',(64.7902651077865,247.54078190379,28.096802244712)) ;
#105861=CARTESIAN_POINT('Origin',(64.7902651077865,248.040265107786,23.0213203435596)) ;
#105862=CARTESIAN_POINT('Origin',(64.7902651077865,247.69078190379,25.759956707196)) ;
#105863=CARTESIAN_POINT('',(64.9402651077865,247.69078190379,28.5023074499214)) ;
#105864=CARTESIAN_POINT('',(64.9402651077865,247.69078190379,25.759956707196)) ;
#105865=CARTESIAN_POINT('',(64.7902651077865,247.54078190379,28.4985930708324)) ;
#105866=CARTESIAN_POINT('Ctrl Pts',(64.9402651077865,247.69078190379,28.5023074499214)) ;
#105867=CARTESIAN_POINT('Ctrl Pts',(64.9402651077865,247.689323780486,28.5022678161701)) ;
#105868=CARTESIAN_POINT('Ctrl Pts',(64.940243846551,247.687865731145,28.5022283083713)) ;
#105869=CARTESIAN_POINT('Ctrl Pts',(64.9402013305491,247.686408220711,28.5021889366962)) ;
#105870=CARTESIAN_POINT('Ctrl Pts',(64.9396551395109,247.667683996822,28.5016831399336)) ;
#105871=CARTESIAN_POINT('Ctrl Pts',(64.9356062703199,247.649225833959,28.5012049258669)) ;
#105872=CARTESIAN_POINT('Ctrl Pts',(64.928263675975,247.631990789003,28.5007714713078)) ;
#105873=CARTESIAN_POINT('Ctrl Pts',(64.9206090302591,247.6140232755,28.5003195954547)) ;
#105874=CARTESIAN_POINT('Ctrl Pts',(64.9095180038061,247.597721356829,28.49992447295)) ;
#105875=CARTESIAN_POINT('Ctrl Pts',(64.8956136387305,247.58400322133,28.4995981034064)) ;
#105876=CARTESIAN_POINT('Ctrl Pts',(64.8817129938794,247.570288756228,28.4992718211856)) ;
#105877=CARTESIAN_POINT('Ctrl Pts',(64.8652664191737,247.559419078944,28.4990202369966)) ;
#105878=CARTESIAN_POINT('Ctrl Pts',(64.8471986491032,247.552006647086,28.4988497601076)) ;
#105879=CARTESIAN_POINT('Ctrl Pts',(64.8291331055122,247.544595128658,28.4986793042264)) ;
#105880=CARTESIAN_POINT('Ctrl Pts',(64.8097925816883,247.54078190379,28.4985930708322)) ;
#105881=CARTESIAN_POINT('Ctrl Pts',(64.7902651077865,247.54078190379,28.4985930708322)) ;
#105882=CARTESIAN_POINT('',(64.7902651077865,247.54078190379,25.759956707196)) ;
#105883=CARTESIAN_POINT('Origin',(64.7902651077865,248.040265107786,28.5213203435596)) ;
#105884=CARTESIAN_POINT('',(64.9402651077865,248.389748311783,28.5023074499214)) ;
#105885=CARTESIAN_POINT('Origin',(64.9402651077865,248.040265107786,28.5213203435596)) ;
#105886=CARTESIAN_POINT('',(64.7902651077865,248.539748311783,28.4985930708324)) ;
#105887=CARTESIAN_POINT('Ctrl Pts',(64.9402651077865,248.389748311783,28.5023074499214)) ;
#105888=CARTESIAN_POINT('Ctrl Pts',(64.9402651077865,248.391206435086,28.5022678161702)) ;
#105889=CARTESIAN_POINT('Ctrl Pts',(64.940243846551,248.392664484427,28.5022283083715)) ;
#105890=CARTESIAN_POINT('Ctrl Pts',(64.9402013305492,248.394121994861,28.5021889366964)) ;
#105891=CARTESIAN_POINT('Ctrl Pts',(64.939655139511,248.412846218751,28.5016831399329)) ;
#105892=CARTESIAN_POINT('Ctrl Pts',(64.9356062703199,248.431304381614,28.5012049258645)) ;
#105893=CARTESIAN_POINT('Ctrl Pts',(64.9282636759751,248.44853942657,28.500771471306)) ;
#105894=CARTESIAN_POINT('Ctrl Pts',(64.9206090302595,248.466506940072,28.5003195954534)) ;
#105895=CARTESIAN_POINT('Ctrl Pts',(64.9095180038067,248.482808858743,28.4999244729504)) ;
#105896=CARTESIAN_POINT('Ctrl Pts',(64.8956136387307,248.496526994243,28.4995981034069)) ;
#105897=CARTESIAN_POINT('Ctrl Pts',(64.8817129938793,248.510241459345,28.4992718211861)) ;
#105898=CARTESIAN_POINT('Ctrl Pts',(64.8652664191737,248.521111136629,28.4990202369969)) ;
#105899=CARTESIAN_POINT('Ctrl Pts',(64.8471986491033,248.528523568487,28.4988497601079)) ;
#105900=CARTESIAN_POINT('Ctrl Pts',(64.8291331055125,248.535935086915,28.4986793042266)) ;
#105901=CARTESIAN_POINT('Ctrl Pts',(64.8097925816883,248.539748311783,28.4985930708331)) ;
#105902=CARTESIAN_POINT('Ctrl Pts',(64.7902651077865,248.539748311783,28.4985930708331)) ;
#105903=CARTESIAN_POINT('Origin',(64.7902651077865,248.040265107786,28.5213203435596)) ;
#105904=CARTESIAN_POINT('Origin',(64.7902651077865,248.389748311783,25.4082910455649)) ;
#105905=CARTESIAN_POINT('',(64.9402651077865,248.389748311783,27.9589677074491)) ;
#105906=CARTESIAN_POINT('',(64.9402651077865,248.389748311783,25.4082910455649)) ;
#105907=CARTESIAN_POINT('',(64.7902651077865,248.539748311783,28.096802244712)) ;
#105908=CARTESIAN_POINT('Ctrl Pts',(64.9402651077865,248.389748311783,27.9589677074491)) ;
#105909=CARTESIAN_POINT('Ctrl Pts',(64.9402651077865,248.390325382447,27.9595053771305)) ;
#105910=CARTESIAN_POINT('Ctrl Pts',(64.940261777681,248.390902501024,27.9600430036291)) ;
#105911=CARTESIAN_POINT('Ctrl Pts',(64.9400834366345,248.406352717361,27.974433616113)) ;
#105912=CARTESIAN_POINT('Ctrl Pts',(64.9376982652987,248.421311718545,27.9883070896991)) ;
#105913=CARTESIAN_POINT('Ctrl Pts',(64.9285249168183,248.449727016612,28.014554999575)) ;
#105914=CARTESIAN_POINT('Ctrl Pts',(64.9218878905887,248.463346223256,28.027084422084)) ;
#105915=CARTESIAN_POINT('Ctrl Pts',(64.9030518920067,248.490123893161,28.0516371458428)) ;
#105916=CARTESIAN_POINT('Ctrl Pts',(64.890241559628,248.503189653969,28.0635653016335)) ;
#105917=CARTESIAN_POINT('Ctrl Pts',(64.8622234505159,248.522187169328,28.0808650678765)) ;
#105918=CARTESIAN_POINT('Ctrl Pts',(64.8483068832618,248.528988708093,28.087041829166)) ;
#105919=CARTESIAN_POINT('Ctrl Pts',(64.8193104176513,248.537595143822,28.0948515246968)) ;
#105920=CARTESIAN_POINT('Ctrl Pts',(64.8049443310403,248.539748311783,28.096802244712)) ;
#105921=CARTESIAN_POINT('Ctrl Pts',(64.7902651077865,248.539748311783,28.096802244712)) ;
#105922=CARTESIAN_POINT('',(64.7902651077865,248.539748311783,25.4082910455649)) ;
#105923=CARTESIAN_POINT('Origin',(64.7902651077865,248.040265107786,23.0213203435596)) ;
#105924=CARTESIAN_POINT('',(64.9402651077865,249.233703776962,27.8252982934377)) ;
#105925=CARTESIAN_POINT('Origin',(64.9402651077865,248.040265107786,23.0213203435596)) ;
#105926=CARTESIAN_POINT('',(64.7902651077865,249.133638513944,28.0027392774284)) ;
#105927=CARTESIAN_POINT('Ctrl Pts',(64.9402651077865,249.233703776962,27.8252982934377)) ;
#105928=CARTESIAN_POINT('Ctrl Pts',(64.9402651077865,249.233321099216,27.8259879723329)) ;
#105929=CARTESIAN_POINT('Ctrl Pts',(64.940261777681,249.232938362558,27.8266776249647)) ;
#105930=CARTESIAN_POINT('Ctrl Pts',(64.9400834366348,249.22269127745,27.8451382901554)) ;
#105931=CARTESIAN_POINT('Ctrl Pts',(64.9376982652992,249.212751561005,27.8629553331984)) ;
#105932=CARTESIAN_POINT('Ctrl Pts',(64.9285249168188,249.193838056834,27.896699388929)) ;
#105933=CARTESIAN_POINT('Ctrl Pts',(64.921887890589,249.184757226094,27.9128241441551)) ;
#105934=CARTESIAN_POINT('Ctrl Pts',(64.9030518920067,249.166877357539,27.9444499271496)) ;
#105935=CARTESIAN_POINT('Ctrl Pts',(64.890241559628,249.158137083433,27.9598318195758)) ;
#105936=CARTESIAN_POINT('Ctrl Pts',(64.8622234505159,249.145415294424,27.9821554300886)) ;
#105937=CARTESIAN_POINT('Ctrl Pts',(64.8483068832618,249.14085537087,27.9901316702287)) ;
#105938=CARTESIAN_POINT('Ctrl Pts',(64.8193104176513,249.135083492728,28.0002186669547)) ;
#105939=CARTESIAN_POINT('Ctrl Pts',(64.8049443310403,249.133638513944,28.0027392774284)) ;
#105940=CARTESIAN_POINT('Ctrl Pts',(64.7902651077865,249.133638513944,28.0027392774284)) ;
#105941=CARTESIAN_POINT('Origin',(64.7902651077865,248.040265107786,23.0213203435596)) ;
#105942=CARTESIAN_POINT('Origin',(64.7902651077865,248.554172007067,25.7339145522423)) ;
#105943=CARTESIAN_POINT('',(64.9402651077865,249.401604991106,28.342045096078)) ;
#105944=CARTESIAN_POINT('',(64.9402651077865,248.554172007067,25.7339145522423)) ;
#105945=CARTESIAN_POINT('',(64.7902651077865,249.257798707399,28.3848650607978)) ;
#105946=CARTESIAN_POINT('Ctrl Pts',(64.9402651077865,249.401604991106,28.342045096078)) ;
#105947=CARTESIAN_POINT('Ctrl Pts',(64.9402651077865,249.400205985933,28.3424579870215)) ;
#105948=CARTESIAN_POINT('Ctrl Pts',(64.940243846551,249.398807090025,28.3428709748967)) ;
#105949=CARTESIAN_POINT('Ctrl Pts',(64.9402013305491,249.397408748713,28.3432839257022)) ;
#105950=CARTESIAN_POINT('Ctrl Pts',(64.9396551395108,249.379444653775,28.3485889877849)) ;
#105951=CARTESIAN_POINT('Ctrl Pts',(64.9356062703196,249.361742121431,28.3538380651888)) ;
#105952=CARTESIAN_POINT('Ctrl Pts',(64.9282636759748,249.345216674792,28.3587517471961)) ;
#105953=CARTESIAN_POINT('Ctrl Pts',(64.920609030259,249.327988916676,28.3638742547405)) ;
#105954=CARTESIAN_POINT('Ctrl Pts',(64.909518003806,249.312362771127,28.368536040818)) ;
#105955=CARTESIAN_POINT('Ctrl Pts',(64.8956136387302,249.299215195234,28.3724647819372)) ;
#105956=CARTESIAN_POINT('Ctrl Pts',(64.8817129938788,249.286071137079,28.3763924718902)) ;
#105957=CARTESIAN_POINT('Ctrl Pts',(64.8652664191736,249.275655715879,28.3795121161121)) ;
#105958=CARTESIAN_POINT('Ctrl Pts',(64.8471986491032,249.268553394004,28.3816405503694)) ;
#105959=CARTESIAN_POINT('Ctrl Pts',(64.8291331055125,249.261451947343,28.3837687223412)) ;
#105960=CARTESIAN_POINT('Ctrl Pts',(64.8097925816883,249.257798707399,28.3848650607976)) ;
#105961=CARTESIAN_POINT('Ctrl Pts',(64.7902651077865,249.257798707399,28.3848650607976)) ;
#105962=CARTESIAN_POINT('',(64.7902651077865,248.411513529623,25.7802671013986)) ;
#105963=CARTESIAN_POINT('Origin',(64.7902651077865,249.739858576849,28.252131183183)) ;
#105964=CARTESIAN_POINT('',(64.9402651077865,250.066361548098,28.1260525975114)) ;
#105965=CARTESIAN_POINT('Origin',(64.9402651077865,249.739858576849,28.252131183183)) ;
#105966=CARTESIAN_POINT('',(64.7902651077865,250.207872219281,28.0761674639184)) ;
#105967=CARTESIAN_POINT('Ctrl Pts',(64.9402651077865,250.066361548098,28.1260525975114)) ;
#105968=CARTESIAN_POINT('Ctrl Pts',(64.9402651077865,250.067736058265,28.1255643186932)) ;
#105969=CARTESIAN_POINT('Ctrl Pts',(64.940243846551,250.069110537011,28.1250761825189)) ;
#105970=CARTESIAN_POINT('Ctrl Pts',(64.9402013305491,250.070484545289,28.1245883423371)) ;
#105971=CARTESIAN_POINT('Ctrl Pts',(64.9396551395109,250.088136040636,28.1183211976397)) ;
#105972=CARTESIAN_POINT('Ctrl Pts',(64.9356062703197,250.105543020433,28.112162503026)) ;
#105973=CARTESIAN_POINT('Ctrl Pts',(64.9282636759749,250.121800577422,28.1064243414531)) ;
#105974=CARTESIAN_POINT('Ctrl Pts',(64.9206090302592,250.138749060902,28.1004423149599)) ;
#105975=CARTESIAN_POINT('Ctrl Pts',(64.9095180038062,250.154131007314,28.095028961218)) ;
#105976=CARTESIAN_POINT('Ctrl Pts',(64.8956136387303,250.167076875737,28.0904794283365)) ;
#105977=CARTESIAN_POINT('Ctrl Pts',(64.8817129938789,250.180019280389,28.085931112719)) ;
#105978=CARTESIAN_POINT('Ctrl Pts',(64.8652664191733,250.190279214009,28.0823329269325)) ;
#105979=CARTESIAN_POINT('Ctrl Pts',(64.847198649103,250.197276175373,28.0798802263628)) ;
#105980=CARTESIAN_POINT('Ctrl Pts',(64.8291331055122,250.204272274506,28.0774278280377)) ;
#105981=CARTESIAN_POINT('Ctrl Pts',(64.8097925816882,250.20787221928,28.0761674639187)) ;
#105982=CARTESIAN_POINT('Ctrl Pts',(64.7902651077865,250.20787221928,28.0761674639188)) ;
#105983=CARTESIAN_POINT('Origin',(64.7902651077865,249.739858576849,28.252131183183)) ;
#105984=CARTESIAN_POINT('Origin',(64.7902651077865,249.110257898277,25.1834681346239)) ;
#105985=CARTESIAN_POINT('',(64.9402651077865,249.898460333955,27.6093057948708)) ;
#105986=CARTESIAN_POINT('',(64.9402651077865,249.110257898277,25.1834681346239)) ;
#105987=CARTESIAN_POINT('',(64.7902651077865,250.083712025826,27.694041680549)) ;
#105988=CARTESIAN_POINT('Ctrl Pts',(64.9402651077865,249.898460333955,27.6093057948708)) ;
#105989=CARTESIAN_POINT('Ctrl Pts',(64.9402651077865,249.89917530984,27.6096388244826)) ;
#105990=CARTESIAN_POINT('Ctrl Pts',(64.940261777681,249.899890317948,27.6099717982194)) ;
#105991=CARTESIAN_POINT('Ctrl Pts',(64.9400834366345,249.91903129069,27.6188837045809)) ;
#105992=CARTESIAN_POINT('Ctrl Pts',(64.9376982652987,249.937545285353,27.6274555764536)) ;
#105993=CARTESIAN_POINT('Ctrl Pts',(64.9285249168183,249.97268088996,27.6436380121774)) ;
#105994=CARTESIAN_POINT('Ctrl Pts',(64.9218878905887,249.98950532967,27.6513456347973)) ;
#105995=CARTESIAN_POINT('Ctrl Pts',(64.9030518920066,250.022559616025,27.6664219076506)) ;
#105996=CARTESIAN_POINT('Ctrl Pts',(64.890241559628,250.038671895832,27.6737287158085)) ;
#105997=CARTESIAN_POINT('Ctrl Pts',(64.862223450516,250.062085528376,27.6843112161272)) ;
#105998=CARTESIAN_POINT('Ctrl Pts',(64.8483068832619,250.070462900348,27.6880838741351)) ;
#105999=CARTESIAN_POINT('Ctrl Pts',(64.8193104176514,250.08106143577,27.6928518010587)) ;
#106000=CARTESIAN_POINT('Ctrl Pts',(64.8049443310404,250.083712025825,27.6940416805491)) ;
#106001=CARTESIAN_POINT('Ctrl Pts',(64.7902651077866,250.083712025825,27.6940416805491)) ;
#106002=CARTESIAN_POINT('',(64.7902651077865,249.252916375722,25.1371155854676)) ;
#106003=CARTESIAN_POINT('Origin',(64.7902651077865,248.040265107786,23.0213203435596)) ;
#106004=CARTESIAN_POINT('',(64.9402651077865,250.65980355802,27.2213820464098)) ;
#106005=CARTESIAN_POINT('Origin',(64.9402651077865,248.040265107786,23.0213203435596)) ;
#106006=CARTESIAN_POINT('',(64.7902651077865,250.619468117123,27.4210603173112)) ;
#106007=CARTESIAN_POINT('Ctrl Pts',(64.9402651077865,250.65980355802,27.2213820464098)) ;
#106008=CARTESIAN_POINT('Ctrl Pts',(64.9402651077865,250.659652732354,27.222156223949)) ;
#106009=CARTESIAN_POINT('Ctrl Pts',(64.9402617776811,250.659501842545,27.2229303947088)) ;
#106010=CARTESIAN_POINT('Ctrl Pts',(64.9400834366342,250.655460944751,27.2436540540784)) ;
#106011=CARTESIAN_POINT('Ctrl Pts',(64.9376982652983,250.651513481746,27.2636706102647)) ;
#106012=CARTESIAN_POINT('Ctrl Pts',(64.9285249168178,250.643953157038,27.3016077085626)) ;
#106013=CARTESIAN_POINT('Ctrl Pts',(64.9218878905883,250.640299597185,27.3197493931144)) ;
#106014=CARTESIAN_POINT('Ctrl Pts',(64.9030518920067,250.633067736091,27.3553524833538)) ;
#106015=CARTESIAN_POINT('Ctrl Pts',(64.890241559628,250.629508507613,27.3726824256129)) ;
#106016=CARTESIAN_POINT('Ctrl Pts',(64.8622234505159,250.624307742302,27.3978446898607)) ;
#106017=CARTESIAN_POINT('Ctrl Pts',(64.8483068832619,250.622435791047,27.4068396388929)) ;
#106018=CARTESIAN_POINT('Ctrl Pts',(64.8193104176513,250.620063462139,27.4182165512944)) ;
#106019=CARTESIAN_POINT('Ctrl Pts',(64.8049443310403,250.619468117123,27.4210603173112)) ;
#106020=CARTESIAN_POINT('Ctrl Pts',(64.7902651077865,250.619468117123,27.4210603173112)) ;
#106021=CARTESIAN_POINT('Origin',(64.7902651077865,248.040265107786,23.0213203435596)) ;
#106022=CARTESIAN_POINT('Origin',(64.7902651077865,249.367257322442,25.4423447763876)) ;
#106023=CARTESIAN_POINT('',(64.9402651077865,250.979170645629,27.6609531317893)) ;
#106024=CARTESIAN_POINT('',(64.9402651077865,249.367257322442,25.4423447763876)) ;
#106025=CARTESIAN_POINT('',(64.7902651077865,250.855634839223,27.7461159238265)) ;
#106026=CARTESIAN_POINT('Ctrl Pts',(64.9402651077865,250.979170645629,27.6609531317893)) ;
#106027=CARTESIAN_POINT('Ctrl Pts',(64.9402651077865,250.977967702962,27.661778130785)) ;
#106028=CARTESIAN_POINT('Ctrl Pts',(64.940243846551,250.976764894165,27.6626031882036)) ;
#106029=CARTESIAN_POINT('Ctrl Pts',(64.9402013305491,250.975562601365,27.6634280389876)) ;
#106030=CARTESIAN_POINT('Ctrl Pts',(64.9396551395109,250.960117086155,27.6740246634766)) ;
#106031=CARTESIAN_POINT('Ctrl Pts',(64.9356062703198,250.944903031536,27.6844872160811)) ;
#106032=CARTESIAN_POINT('Ctrl Pts',(64.928263675975,250.93070480907,27.6942670492246)) ;
#106033=CARTESIAN_POINT('Ctrl Pts',(64.9206090302591,250.915903179338,27.7044625134376)) ;
#106034=CARTESIAN_POINT('Ctrl Pts',(64.9095180038061,250.902482402912,27.7137248799966)) ;
#106035=CARTESIAN_POINT('Ctrl Pts',(64.8956136387304,250.891192362958,27.721524159225)) ;
#106036=CARTESIAN_POINT('Ctrl Pts',(64.8817129938793,250.879905343744,27.7293213516936)) ;
#106037=CARTESIAN_POINT('Ctrl Pts',(64.8652664191737,250.870963712622,27.7355068518136)) ;
#106038=CARTESIAN_POINT('Ctrl Pts',(64.8471986491032,250.864866725478,27.7397258512424)) ;
#106039=CARTESIAN_POINT('Ctrl Pts',(64.8291331055123,250.858770489662,27.7439443307667)) ;
#106040=CARTESIAN_POINT('Ctrl Pts',(64.8097925816884,250.855634839223,27.7461159238267)) ;
#106041=CARTESIAN_POINT('Ctrl Pts',(64.7902651077866,250.855634839223,27.7461159238267)) ;
#106042=CARTESIAN_POINT('',(64.7902651077865,249.245904773286,25.5305125642315)) ;
#106043=CARTESIAN_POINT('Origin',(64.7902651077865,251.273083995395,27.4709138126218)) ;
#106044=CARTESIAN_POINT('',(64.9402651077865,251.544646348192,27.2501109853232)) ;
#106045=CARTESIAN_POINT('Origin',(64.9402651077865,251.273083995395,27.4709138126218)) ;
#106046=CARTESIAN_POINT('',(64.7902651077865,251.663815640099,27.1589382016729)) ;
#106047=CARTESIAN_POINT('Ctrl Pts',(64.9402651077865,251.544646348192,27.2501109853233)) ;
#106048=CARTESIAN_POINT('Ctrl Pts',(64.9402651077865,251.545802698591,27.2492218575708)) ;
#106049=CARTESIAN_POINT('Ctrl Pts',(64.940243846551,251.546959063183,27.2483328751889)) ;
#106050=CARTESIAN_POINT('Ctrl Pts',(64.9402013305491,251.548115071804,27.2474443196972)) ;
#106051=CARTESIAN_POINT('Ctrl Pts',(64.9396551395109,251.562965987268,27.2360292988668)) ;
#106052=CARTESIAN_POINT('Ctrl Pts',(64.9356062703198,251.577617867525,27.2247929796351)) ;
#106053=CARTESIAN_POINT('Ctrl Pts',(64.928263675975,251.591306533596,27.2143118022833)) ;
#106054=CARTESIAN_POINT('Ctrl Pts',(64.9206090302591,251.605576951405,27.203385187582)) ;
#106055=CARTESIAN_POINT('Ctrl Pts',(64.9095180038061,251.61853323347,27.1934834993828)) ;
#106056=CARTESIAN_POINT('Ctrl Pts',(64.8956136387304,251.629439603015,27.1851561431399)) ;
#106057=CARTESIAN_POINT('Ctrl Pts',(64.8817129938793,251.640343054474,27.1768310149481)) ;
#106058=CARTESIAN_POINT('Ctrl Pts',(64.8652664191738,251.648988930644,27.1702384430593)) ;
#106059=CARTESIAN_POINT('Ctrl Pts',(64.8471986491033,251.654885510185,27.1657436062294)) ;
#106060=CARTESIAN_POINT('Ctrl Pts',(64.8291331055125,251.660781363094,27.1612493232952)) ;
#106061=CARTESIAN_POINT('Ctrl Pts',(64.8097925816883,251.663815640098,27.1589382016717)) ;
#106062=CARTESIAN_POINT('Ctrl Pts',(64.7902651077865,251.663815640098,27.1589382016716)) ;
#106063=CARTESIAN_POINT('Origin',(64.7902651077865,251.273083995395,27.4709138126218)) ;
#106064=CARTESIAN_POINT('Origin',(64.7902651077865,249.726029135361,24.746999133324)) ;
#106065=CARTESIAN_POINT('',(64.9402651077865,251.225279260583,26.8105398999439)) ;
#106066=CARTESIAN_POINT('',(64.9402651077865,249.726029135361,24.746999133324)) ;
#106067=CARTESIAN_POINT('',(64.7902651077865,251.427648917999,26.8338825951576)) ;
#106068=CARTESIAN_POINT('Ctrl Pts',(64.9402651077865,251.225279260583,26.8105398999439)) ;
#106069=CARTESIAN_POINT('Ctrl Pts',(64.9402651077865,251.226062154865,26.8106356902272)) ;
#106070=CARTESIAN_POINT('Ctrl Pts',(64.940261777681,251.226845062528,26.8107314174126)) ;
#106071=CARTESIAN_POINT('Ctrl Pts',(64.9400834366348,251.247803139901,26.8132922581638)) ;
#106072=CARTESIAN_POINT('Ctrl Pts',(64.9376982652992,251.26805984925,26.815723453781)) ;
#106073=CARTESIAN_POINT('Ctrl Pts',(64.9285249168187,251.306476442616,26.8202563657946)) ;
#106074=CARTESIAN_POINT('Ctrl Pts',(64.9218878905889,251.324859222012,26.8223877127212)) ;
#106075=CARTESIAN_POINT('Ctrl Pts',(64.9030518920067,251.360954540964,26.8265117640394)) ;
#106076=CARTESIAN_POINT('Ctrl Pts',(64.890241559628,251.378536157563,26.8284819832727)) ;
#106077=CARTESIAN_POINT('Ctrl Pts',(64.8622234505159,251.404074017806,26.8313113288033)) ;
#106078=CARTESIAN_POINT('Ctrl Pts',(64.8483068832618,251.413207187447,26.832310589478)) ;
#106079=CARTESIAN_POINT('Ctrl Pts',(64.8193104176513,251.42476036407,26.8335700298871)) ;
#106080=CARTESIAN_POINT('Ctrl Pts',(64.8049443310403,251.427648917999,26.8338825951576)) ;
#106081=CARTESIAN_POINT('Ctrl Pts',(64.7902651077865,251.427648917999,26.8338825951576)) ;
#106082=CARTESIAN_POINT('',(64.7902651077865,249.847381684517,24.6588313454802)) ;
#106083=CARTESIAN_POINT('Origin',(64.7902651077865,248.040265107786,23.0213203435596)) ;
#106084=CARTESIAN_POINT('',(64.9402651077865,251.829484664171,26.2063344963563)) ;
#106085=CARTESIAN_POINT('Origin',(64.9402651077865,248.040265107786,23.0213203435596)) ;
#106086=CARTESIAN_POINT('',(64.7902651077865,251.852827359384,26.4087041537722)) ;
#106087=CARTESIAN_POINT('Ctrl Pts',(64.9402651077865,251.829484664171,26.2063344963563)) ;
#106088=CARTESIAN_POINT('Ctrl Pts',(64.9402651077865,251.829580454454,26.2071173906402)) ;
#106089=CARTESIAN_POINT('Ctrl Pts',(64.940261777681,251.82967618164,26.2079002983041)) ;
#106090=CARTESIAN_POINT('Ctrl Pts',(64.9400834366345,251.832237022391,26.2288583756769)) ;
#106091=CARTESIAN_POINT('Ctrl Pts',(64.9376982652987,251.834668218008,26.2491150850258)) ;
#106092=CARTESIAN_POINT('Ctrl Pts',(64.9285249168183,251.839201130021,26.2875316783904)) ;
#106093=CARTESIAN_POINT('Ctrl Pts',(64.9218878905886,251.841332476948,26.3059144577855)) ;
#106094=CARTESIAN_POINT('Ctrl Pts',(64.9030518920066,251.845456528266,26.3420097767375)) ;
#106095=CARTESIAN_POINT('Ctrl Pts',(64.8902415596279,251.847426747499,26.3595913933363)) ;
#106096=CARTESIAN_POINT('Ctrl Pts',(64.862223450516,251.85025609303,26.3851292535788)) ;
#106097=CARTESIAN_POINT('Ctrl Pts',(64.8483068832619,251.851255353705,26.3942624232203)) ;
#106098=CARTESIAN_POINT('Ctrl Pts',(64.8193104176513,251.852514794114,26.4058155998437)) ;
#106099=CARTESIAN_POINT('Ctrl Pts',(64.8049443310403,251.852827359384,26.4087041537722)) ;
#106100=CARTESIAN_POINT('Ctrl Pts',(64.7902651077865,251.852827359384,26.4087041537722)) ;
#106101=CARTESIAN_POINT('Origin',(64.7902651077865,248.040265107786,23.0213203435596)) ;
#106102=CARTESIAN_POINT('Origin',(64.7902651077865,250.050447394148,24.9137882607786)) ;
#106103=CARTESIAN_POINT('',(64.9402651077865,252.26905574955,26.5257015839661)) ;
#106104=CARTESIAN_POINT('',(64.9402651077865,250.050447394148,24.9137882607786)) ;
#106105=CARTESIAN_POINT('',(64.7902651077865,252.1778829659,26.6448708758722)) ;
#106106=CARTESIAN_POINT('Ctrl Pts',(64.9402651077865,252.26905574955,26.5257015839661)) ;
#106107=CARTESIAN_POINT('Ctrl Pts',(64.9402651077865,252.268166621798,26.5268579343644)) ;
#106108=CARTESIAN_POINT('Ctrl Pts',(64.940243846551,252.267277639417,26.5280142989575)) ;
#106109=CARTESIAN_POINT('Ctrl Pts',(64.9402013305492,252.266389083925,26.5291703075781)) ;
#106110=CARTESIAN_POINT('Ctrl Pts',(64.9396551395109,252.254974063088,26.544021223037)) ;
#106111=CARTESIAN_POINT('Ctrl Pts',(64.9356062703198,252.243737743861,26.558673103298)) ;
#106112=CARTESIAN_POINT('Ctrl Pts',(64.928263675975,252.233256566509,26.5723617693692)) ;
#106113=CARTESIAN_POINT('Ctrl Pts',(64.9206090302592,252.222329951808,26.5866321871775)) ;
#106114=CARTESIAN_POINT('Ctrl Pts',(64.9095180038065,252.21242826361,26.5995884692432)) ;
#106115=CARTESIAN_POINT('Ctrl Pts',(64.8956136387306,252.204100907367,26.6104948387888)) ;
#106116=CARTESIAN_POINT('Ctrl Pts',(64.8817129938792,252.195775779175,26.6213982902478)) ;
#106117=CARTESIAN_POINT('Ctrl Pts',(64.8652664191737,252.189183207286,26.6300441664177)) ;
#106118=CARTESIAN_POINT('Ctrl Pts',(64.8471986491032,252.184688370456,26.6359407459586)) ;
#106119=CARTESIAN_POINT('Ctrl Pts',(64.8291331055124,252.180194087522,26.6418365988679)) ;
#106120=CARTESIAN_POINT('Ctrl Pts',(64.8097925816884,252.1778829659,26.6448708758726)) ;
#106121=CARTESIAN_POINT('Ctrl Pts',(64.7902651077865,252.1778829659,26.6448708758726)) ;
#106122=CARTESIAN_POINT('',(64.7902651077865,249.962279606305,25.0351408099348)) ;
#106123=CARTESIAN_POINT('Origin',(64.7902651077865,252.489858576849,26.2541392311682)) ;
#106124=CARTESIAN_POINT('',(64.9402651077865,252.679897896016,25.9602258814027)) ;
#106125=CARTESIAN_POINT('Origin',(64.9402651077865,252.489858576849,26.2541392311682)) ;
#106126=CARTESIAN_POINT('',(64.7902651077865,252.765060688053,25.8366900749965)) ;
#106127=CARTESIAN_POINT('Ctrl Pts',(64.9402651077865,252.67989789602,25.9602258813973)) ;
#106128=CARTESIAN_POINT('Ctrl Pts',(64.9402651077864,252.680722895014,25.9590229387317)) ;
#106129=CARTESIAN_POINT('Ctrl Pts',(64.9402438465509,252.68154795243,25.957820129936)) ;
#106130=CARTESIAN_POINT('Ctrl Pts',(64.9402013305492,252.682372803213,25.9566178371377)) ;
#106131=CARTESIAN_POINT('Ctrl Pts',(64.9396551395109,252.692969427709,25.9411723219305)) ;
#106132=CARTESIAN_POINT('Ctrl Pts',(64.9356062703198,252.703431980308,25.9259582673091)) ;
#106133=CARTESIAN_POINT('Ctrl Pts',(64.928263675975,252.713211813452,25.9117600448439)) ;
#106134=CARTESIAN_POINT('Ctrl Pts',(64.9206090302592,252.723407277665,25.8969584151117)) ;
#106135=CARTESIAN_POINT('Ctrl Pts',(64.9095180038063,252.732669644223,25.8835376386852)) ;
#106136=CARTESIAN_POINT('Ctrl Pts',(64.8956136387305,252.740468923451,25.8722475987305)) ;
#106137=CARTESIAN_POINT('Ctrl Pts',(64.8817129938792,252.74826611592,25.8609605795167)) ;
#106138=CARTESIAN_POINT('Ctrl Pts',(64.8652664191738,252.75445161604,25.8520189483948)) ;
#106139=CARTESIAN_POINT('Ctrl Pts',(64.8471986491033,252.758670615469,25.8459219612514)) ;
#106140=CARTESIAN_POINT('Ctrl Pts',(64.8291331055124,252.762889094994,25.8398257254358)) ;
#106141=CARTESIAN_POINT('Ctrl Pts',(64.8097925816883,252.765060688054,25.8366900749968)) ;
#106142=CARTESIAN_POINT('Ctrl Pts',(64.7902651077865,252.765060688054,25.8366900749968)) ;
#106143=CARTESIAN_POINT('Origin',(64.7902651077865,252.489858576849,26.2541392311682)) ;
#106144=CARTESIAN_POINT('Origin',(64.7902651077865,250.176786044017,24.1416086685709)) ;
#106145=CARTESIAN_POINT('',(64.9402651077865,252.240326810636,25.6408587937931)) ;
#106146=CARTESIAN_POINT('',(64.9402651077865,250.176786044017,24.1416086685709)) ;
#106147=CARTESIAN_POINT('',(64.7902651077865,252.440005081538,25.6005233528965)) ;
#106148=CARTESIAN_POINT('Ctrl Pts',(64.9402651077865,252.240326810636,25.6408587937931)) ;
#106149=CARTESIAN_POINT('Ctrl Pts',(64.9402651077865,252.241100988176,25.6407079681271)) ;
#106150=CARTESIAN_POINT('Ctrl Pts',(64.9402617776811,252.241875158935,25.6405570783181)) ;
#106151=CARTESIAN_POINT('Ctrl Pts',(64.9400834366342,252.262598818305,25.6365161805235)) ;
#106152=CARTESIAN_POINT('Ctrl Pts',(64.9376982652982,252.282615374491,25.6325687175188)) ;
#106153=CARTESIAN_POINT('Ctrl Pts',(64.9285249168178,252.320552472789,25.6250083928117)) ;
#106154=CARTESIAN_POINT('Ctrl Pts',(64.9218878905884,252.338694157341,25.6213548329578)) ;
#106155=CARTESIAN_POINT('Ctrl Pts',(64.9030518920066,252.374297247581,25.6141229718641)) ;
#106156=CARTESIAN_POINT('Ctrl Pts',(64.8902415596279,252.39162718984,25.6105637433868)) ;
#106157=CARTESIAN_POINT('Ctrl Pts',(64.8622234505159,252.416789454087,25.6053629780756)) ;
#106158=CARTESIAN_POINT('Ctrl Pts',(64.8483068832619,252.42578440312,25.6034910268201)) ;
#106159=CARTESIAN_POINT('Ctrl Pts',(64.8193104176513,252.437161315521,25.6011186979124)) ;
#106160=CARTESIAN_POINT('Ctrl Pts',(64.8049443310403,252.440005081538,25.6005233528966)) ;
#106161=CARTESIAN_POINT('Ctrl Pts',(64.7902651077865,252.440005081538,25.6005233528966)) ;
#106162=CARTESIAN_POINT('',(64.7902651077865,250.26495383186,24.0202561194147)) ;
#106163=CARTESIAN_POINT('Origin',(64.7902651077865,248.040265107786,23.0213203435596)) ;
#106164=CARTESIAN_POINT('',(64.9402651077865,252.628250559098,24.8795155697285)) ;
#106165=CARTESIAN_POINT('Origin',(64.9402651077865,248.040265107786,23.0213203435596)) ;
#106166=CARTESIAN_POINT('',(64.7902651077865,252.712986444776,25.0647672615988)) ;
#106167=CARTESIAN_POINT('Ctrl Pts',(64.9402651077865,252.628250559098,24.8795155697285)) ;
#106168=CARTESIAN_POINT('Ctrl Pts',(64.9402651077865,252.628583588709,24.8802305456133)) ;
#106169=CARTESIAN_POINT('Ctrl Pts',(64.940261777681,252.628916562446,24.8809455537216)) ;
#106170=CARTESIAN_POINT('Ctrl Pts',(64.9400834366345,252.637828468808,24.9000865264628)) ;
#106171=CARTESIAN_POINT('Ctrl Pts',(64.9376982652988,252.64640034068,24.9186005211264)) ;
#106172=CARTESIAN_POINT('Ctrl Pts',(64.9285249168184,252.662582776404,24.9537361257334)) ;
#106173=CARTESIAN_POINT('Ctrl Pts',(64.9218878905887,252.670290399024,24.9705605654437)) ;
#106174=CARTESIAN_POINT('Ctrl Pts',(64.9030518920066,252.685366671877,25.0036148517979)) ;
#106175=CARTESIAN_POINT('Ctrl Pts',(64.8902415596279,252.692673480035,25.0197271316054)) ;
#106176=CARTESIAN_POINT('Ctrl Pts',(64.8622234505159,252.703255980354,25.0431407641494)) ;
#106177=CARTESIAN_POINT('Ctrl Pts',(64.8483068832618,252.707028638362,25.051518136121)) ;
#106178=CARTESIAN_POINT('Ctrl Pts',(64.8193104176513,252.711796565285,25.0621166715429)) ;
#106179=CARTESIAN_POINT('Ctrl Pts',(64.8049443310403,252.712986444776,25.0647672615988)) ;
#106180=CARTESIAN_POINT('Ctrl Pts',(64.7902651077865,252.712986444776,25.0647672615988)) ;
#106181=CARTESIAN_POINT('Origin',(64.7902651077865,248.040265107786,23.0213203435596)) ;
#106182=CARTESIAN_POINT('Origin',(64.7902651077865,250.536866817902,24.1999837998328)) ;
#106183=CARTESIAN_POINT('',(64.9402651077865,253.144997361738,25.0474167838718)) ;
#106184=CARTESIAN_POINT('',(64.9402651077865,250.536866817902,24.1999837998328)) ;
#106185=CARTESIAN_POINT('',(64.7902651077865,253.095112228145,25.188927455054)) ;
#106186=CARTESIAN_POINT('Ctrl Pts',(64.9402651077865,253.144997361738,25.0474167838718)) ;
#106187=CARTESIAN_POINT('Ctrl Pts',(64.9402651077865,253.14450908292,25.0487912940387)) ;
#106188=CARTESIAN_POINT('Ctrl Pts',(64.940243846551,253.144020946746,25.0501657727844)) ;
#106189=CARTESIAN_POINT('Ctrl Pts',(64.9402013305491,253.143533106564,25.0515397810629)) ;
#106190=CARTESIAN_POINT('Ctrl Pts',(64.9396551395109,253.137265961864,25.0691912764082)) ;
#106191=CARTESIAN_POINT('Ctrl Pts',(64.9356062703198,253.131107267253,25.0865982562063)) ;
#106192=CARTESIAN_POINT('Ctrl Pts',(64.928263675975,253.12536910568,25.1028558131956)) ;
#106193=CARTESIAN_POINT('Ctrl Pts',(64.9206090302592,253.119387079187,25.1198042966758)) ;
#106194=CARTESIAN_POINT('Ctrl Pts',(64.9095180038063,253.113973725445,25.1351862430875)) ;
#106195=CARTESIAN_POINT('Ctrl Pts',(64.8956136387304,253.109424192563,25.1481321115103)) ;
#106196=CARTESIAN_POINT('Ctrl Pts',(64.8817129938791,253.104875876945,25.161074516162)) ;
#106197=CARTESIAN_POINT('Ctrl Pts',(64.8652664191736,253.101277691159,25.1713344497829)) ;
#106198=CARTESIAN_POINT('Ctrl Pts',(64.8471986491031,253.098824990589,25.1783314111465)) ;
#106199=CARTESIAN_POINT('Ctrl Pts',(64.8291331055122,253.096372592264,25.1853275102792)) ;
#106200=CARTESIAN_POINT('Ctrl Pts',(64.8097925816883,253.095112228145,25.1889274550539)) ;
#106201=CARTESIAN_POINT('Ctrl Pts',(64.7902651077865,253.095112228145,25.1889274550539)) ;
#106202=CARTESIAN_POINT('',(64.7902651077865,250.490514268746,24.3426422772771)) ;
#106203=CARTESIAN_POINT('Origin',(64.7902651077865,253.27107594741,24.7209138126218)) ;
#106204=CARTESIAN_POINT('',(64.9402651077865,253.360989860305,24.382660226879)) ;
#106205=CARTESIAN_POINT('Origin',(64.9402651077865,253.27107594741,24.7209138126218)) ;
#106206=CARTESIAN_POINT('',(64.7902651077865,253.403809825024,24.2388539431727)) ;
#106207=CARTESIAN_POINT('Ctrl Pts',(64.9402651077865,253.360989860307,24.3826602268732)) ;
#106208=CARTESIAN_POINT('Ctrl Pts',(64.9402651077864,253.36140275125,24.3812612217023)) ;
#106209=CARTESIAN_POINT('Ctrl Pts',(64.9402438465509,253.361815739121,24.3798623257963)) ;
#106210=CARTESIAN_POINT('Ctrl Pts',(64.9402013305491,253.362228689927,24.3784639844859)) ;
#106211=CARTESIAN_POINT('Ctrl Pts',(64.9396551395108,253.367533752025,24.3604998895503)) ;
#106212=CARTESIAN_POINT('Ctrl Pts',(64.9356062703196,253.372782829414,24.3427973572038)) ;
#106213=CARTESIAN_POINT('Ctrl Pts',(64.9282636759748,253.377696511422,24.3262719105652)) ;
#106214=CARTESIAN_POINT('Ctrl Pts',(64.9206090302591,253.382819018967,24.3090441524495)) ;
#106215=CARTESIAN_POINT('Ctrl Pts',(64.9095180038062,253.387480805045,24.2934180069007)) ;
#106216=CARTESIAN_POINT('Ctrl Pts',(64.8956136387303,253.391409546165,24.2802704310071)) ;
#106217=CARTESIAN_POINT('Ctrl Pts',(64.8817129938789,253.395337236118,24.2671263728531)) ;
#106218=CARTESIAN_POINT('Ctrl Pts',(64.8652664191735,253.39845688034,24.2567109516527)) ;
#106219=CARTESIAN_POINT('Ctrl Pts',(64.8471986491031,253.400585314597,24.2496086297771)) ;
#106220=CARTESIAN_POINT('Ctrl Pts',(64.8291331055124,253.402713486568,24.2425071831161)) ;
#106221=CARTESIAN_POINT('Ctrl Pts',(64.8097925816883,253.403809825025,24.238853943173)) ;
#106222=CARTESIAN_POINT('Ctrl Pts',(64.7902651077865,253.403809825025,24.238853943173)) ;
#106223=CARTESIAN_POINT('Origin',(64.7902651077865,253.27107594741,24.7209138126218)) ;
#106224=CARTESIAN_POINT('Origin',(64.7902651077865,250.418405397417,23.426556577058)) ;
#106225=CARTESIAN_POINT('',(64.9402651077865,252.844243057664,24.2147590127358)) ;
#106226=CARTESIAN_POINT('',(64.9402651077865,250.418405397417,23.426556577058)) ;
#106227=CARTESIAN_POINT('',(64.7902651077865,253.021684041655,24.1146937497175)) ;
#106228=CARTESIAN_POINT('Ctrl Pts',(64.9402651077865,252.844243057664,24.2147590127358)) ;
#106229=CARTESIAN_POINT('Ctrl Pts',(64.9402651077865,252.844932736563,24.2143763349877)) ;
#106230=CARTESIAN_POINT('Ctrl Pts',(64.9402617776811,252.845622389192,24.213993598331)) ;
#106231=CARTESIAN_POINT('Ctrl Pts',(64.9400834366345,252.864083054386,24.2037465132207)) ;
#106232=CARTESIAN_POINT('Ctrl Pts',(64.9376982652987,252.881900097428,24.1938067967769)) ;
#106233=CARTESIAN_POINT('Ctrl Pts',(64.9285249168183,252.915644153157,24.1748932926068)) ;
#106234=CARTESIAN_POINT('Ctrl Pts',(64.9218878905886,252.931768908382,24.1658124618668)) ;
#106235=CARTESIAN_POINT('Ctrl Pts',(64.9030518920066,252.963394691376,24.1479325933121)) ;
#106236=CARTESIAN_POINT('Ctrl Pts',(64.8902415596279,252.978776583803,24.1391923192062)) ;
#106237=CARTESIAN_POINT('Ctrl Pts',(64.8622234505159,253.001100194315,24.1264705301978)) ;
#106238=CARTESIAN_POINT('Ctrl Pts',(64.8483068832618,253.009076434455,24.1219106066435)) ;
#106239=CARTESIAN_POINT('Ctrl Pts',(64.8193104176514,253.019163431181,24.1161387285016)) ;
#106240=CARTESIAN_POINT('Ctrl Pts',(64.8049443310404,253.021684041655,24.1146937497175)) ;
#106241=CARTESIAN_POINT('Ctrl Pts',(64.7902651077865,253.021684041655,24.1146937497175)) ;
#106242=CARTESIAN_POINT('',(64.7902651077865,250.464757946574,23.2838980996137)) ;
#106243=CARTESIAN_POINT('Origin',(64.7902651077865,248.040265107786,23.0213203435596)) ;
#106244=CARTESIAN_POINT('',(64.9402651077865,252.977912471676,23.3708035475559)) ;
#106245=CARTESIAN_POINT('Origin',(64.9402651077865,248.040265107786,23.0213203435596)) ;
#106246=CARTESIAN_POINT('',(64.7902651077865,253.115747008939,23.5208035475559)) ;
#106247=CARTESIAN_POINT('Ctrl Pts',(64.9402651077865,252.977912471676,23.3708035475559)) ;
#106248=CARTESIAN_POINT('Ctrl Pts',(64.9402651077865,252.978450141357,23.3713806182205)) ;
#106249=CARTESIAN_POINT('Ctrl Pts',(64.940261777681,252.978987767856,23.3719577367977)) ;
#106250=CARTESIAN_POINT('Ctrl Pts',(64.9400834366345,252.99337838034,23.3874079531344)) ;
#106251=CARTESIAN_POINT('Ctrl Pts',(64.9376982652987,253.007251853926,23.4023669543188)) ;
#106252=CARTESIAN_POINT('Ctrl Pts',(64.9285249168183,253.033499763802,23.4307822523852)) ;
#106253=CARTESIAN_POINT('Ctrl Pts',(64.9218878905887,253.046029186311,23.4444014590288)) ;
#106254=CARTESIAN_POINT('Ctrl Pts',(64.9030518920067,253.070581910069,23.4711791289338)) ;
#106255=CARTESIAN_POINT('Ctrl Pts',(64.890241559628,253.08251006586,23.4842448897418)) ;
#106256=CARTESIAN_POINT('Ctrl Pts',(64.8622234505159,253.099809832103,23.5032424051016)) ;
#106257=CARTESIAN_POINT('Ctrl Pts',(64.8483068832618,253.105986593393,23.5100439438662)) ;
#106258=CARTESIAN_POINT('Ctrl Pts',(64.8193104176514,253.113796288923,23.5186503795949)) ;
#106259=CARTESIAN_POINT('Ctrl Pts',(64.8049443310404,253.115747008939,23.5208035475559)) ;
#106260=CARTESIAN_POINT('Ctrl Pts',(64.7902651077866,253.115747008939,23.5208035475559)) ;
#106261=CARTESIAN_POINT('Origin',(64.7902651077865,248.040265107786,23.0213203435596)) ;
#106262=CARTESIAN_POINT('Origin',(64.7902651077865,250.778901471423,23.3708035475559)) ;
#106263=CARTESIAN_POINT('',(64.9402651077865,253.521252214148,23.3708035475559)) ;
#106264=CARTESIAN_POINT('',(64.9402651077865,250.778901471423,23.3708035475559)) ;
#106265=CARTESIAN_POINT('',(64.7902651077865,253.517537835059,23.5208035475559)) ;
#106266=CARTESIAN_POINT('Ctrl Pts',(64.9402651077865,253.521252214148,23.3708035475559)) ;
#106267=CARTESIAN_POINT('Ctrl Pts',(64.9402651077865,253.521212580397,23.3722616708597)) ;
#106268=CARTESIAN_POINT('Ctrl Pts',(64.940243846551,253.521173072598,23.3737197202007)) ;
#106269=CARTESIAN_POINT('Ctrl Pts',(64.9402013305491,253.521133700923,23.3751772306343)) ;
#106270=CARTESIAN_POINT('Ctrl Pts',(64.9396551395109,253.52062790416,23.3939014545241)) ;
#106271=CARTESIAN_POINT('Ctrl Pts',(64.9356062703198,253.520149690092,23.4123596173871)) ;
#106272=CARTESIAN_POINT('Ctrl Pts',(64.928263675975,253.519716235533,23.4295946623432)) ;
#106273=CARTESIAN_POINT('Ctrl Pts',(64.9206090302592,253.51926435968,23.4475621758456)) ;
#106274=CARTESIAN_POINT('Ctrl Pts',(64.9095180038063,253.518869237177,23.4638640945167)) ;
#106275=CARTESIAN_POINT('Ctrl Pts',(64.8956136387304,253.518542867634,23.4775822300162)) ;
#106276=CARTESIAN_POINT('Ctrl Pts',(64.8817129938792,253.518216585413,23.4912966951183)) ;
#106277=CARTESIAN_POINT('Ctrl Pts',(64.8652664191737,253.517965001223,23.5021663724021)) ;
#106278=CARTESIAN_POINT('Ctrl Pts',(64.8471986491033,253.517794524334,23.5095788042594)) ;
#106279=CARTESIAN_POINT('Ctrl Pts',(64.8291331055124,253.517624068453,23.5169903226877)) ;
#106280=CARTESIAN_POINT('Ctrl Pts',(64.8097925816883,253.517537835059,23.5208035475559)) ;
#106281=CARTESIAN_POINT('Ctrl Pts',(64.7902651077866,253.517537835059,23.5208035475559)) ;
#106282=CARTESIAN_POINT('',(64.7902651077865,250.778901471423,23.5208035475559)) ;
#106283=CARTESIAN_POINT('Origin',(64.7902651077865,253.540265107786,23.0213203435596)) ;
#106284=CARTESIAN_POINT('',(64.9402651077865,253.521252214148,22.6718371395634)) ;
#106285=CARTESIAN_POINT('Origin',(64.9402651077865,253.540265107786,23.0213203435596)) ;
#106286=CARTESIAN_POINT('',(64.7902651077865,253.517537835059,22.5218371395634)) ;
#106287=CARTESIAN_POINT('Ctrl Pts',(64.9402651077865,253.521252214148,22.6718371395631)) ;
#106288=CARTESIAN_POINT('Ctrl Pts',(64.9402651077865,253.521212580397,22.6703790162594)) ;
#106289=CARTESIAN_POINT('Ctrl Pts',(64.940243846551,253.521173072598,22.6689209669185)) ;
#106290=CARTESIAN_POINT('Ctrl Pts',(64.9402013305491,253.521133700923,22.667463456485)) ;
#106291=CARTESIAN_POINT('Ctrl Pts',(64.9396551395109,253.52062790416,22.6487392325952)) ;
#106292=CARTESIAN_POINT('Ctrl Pts',(64.9356062703198,253.520149690091,22.6302810697322)) ;
#106293=CARTESIAN_POINT('Ctrl Pts',(64.928263675975,253.519716235533,22.6130460247761)) ;
#106294=CARTESIAN_POINT('Ctrl Pts',(64.9206090302592,253.51926435968,22.5950785112737)) ;
#106295=CARTESIAN_POINT('Ctrl Pts',(64.9095180038063,253.518869237177,22.5787765926026)) ;
#106296=CARTESIAN_POINT('Ctrl Pts',(64.8956136387304,253.518542867634,22.5650584571031)) ;
#106297=CARTESIAN_POINT('Ctrl Pts',(64.8817129938791,253.518216585413,22.5513439920009)) ;
#106298=CARTESIAN_POINT('Ctrl Pts',(64.8652664191736,253.517965001224,22.5404743147172)) ;
#106299=CARTESIAN_POINT('Ctrl Pts',(64.8471986491032,253.517794524335,22.5330618828598)) ;
#106300=CARTESIAN_POINT('Ctrl Pts',(64.8291331055124,253.517624068453,22.5256503644316)) ;
#106301=CARTESIAN_POINT('Ctrl Pts',(64.8097925816883,253.517537835059,22.5218371395634)) ;
#106302=CARTESIAN_POINT('Ctrl Pts',(64.7902651077865,253.517537835059,22.5218371395634)) ;
#106303=CARTESIAN_POINT('Origin',(64.7902651077865,253.540265107786,23.0213203435596)) ;
#106304=CARTESIAN_POINT('Origin',(64.7902651077865,250.427235809792,22.6718371395634)) ;
#106305=CARTESIAN_POINT('',(64.9402651077865,252.977912471676,22.6718371395634)) ;
#106306=CARTESIAN_POINT('',(64.9402651077865,250.427235809792,22.6718371395634)) ;
#106307=CARTESIAN_POINT('',(64.7902651077865,253.115747008939,22.5218371395634)) ;
#106308=CARTESIAN_POINT('Ctrl Pts',(64.9402651077865,252.977912471676,22.6718371395634)) ;
#106309=CARTESIAN_POINT('Ctrl Pts',(64.9402651077865,252.978450141357,22.6712600688988)) ;
#106310=CARTESIAN_POINT('Ctrl Pts',(64.940261777681,252.978987767856,22.6706829503216)) ;
#106311=CARTESIAN_POINT('Ctrl Pts',(64.9400834366345,252.99337838034,22.655232733985)) ;
#106312=CARTESIAN_POINT('Ctrl Pts',(64.9376982652987,253.007251853926,22.6402737328004)) ;
#106313=CARTESIAN_POINT('Ctrl Pts',(64.9285249168183,253.033499763802,22.611858434734)) ;
#106314=CARTESIAN_POINT('Ctrl Pts',(64.9218878905887,253.046029186311,22.5982392280904)) ;
#106315=CARTESIAN_POINT('Ctrl Pts',(64.9030518920067,253.07058191007,22.5714615581854)) ;
#106316=CARTESIAN_POINT('Ctrl Pts',(64.890241559628,253.08251006586,22.5583957973774)) ;
#106317=CARTESIAN_POINT('Ctrl Pts',(64.8622234505159,253.099809832103,22.5393982820177)) ;
#106318=CARTESIAN_POINT('Ctrl Pts',(64.8483068832618,253.105986593393,22.5325967432531)) ;
#106319=CARTESIAN_POINT('Ctrl Pts',(64.8193104176513,253.113796288923,22.5239903075244)) ;
#106320=CARTESIAN_POINT('Ctrl Pts',(64.8049443310403,253.115747008939,22.5218371395634)) ;
#106321=CARTESIAN_POINT('Ctrl Pts',(64.7902651077865,253.115747008939,22.5218371395634)) ;
#106322=CARTESIAN_POINT('',(64.7902651077865,250.427235809792,22.5218371395634)) ;
#106323=CARTESIAN_POINT('Origin',(64.7902651077865,248.040265107786,23.0213203435596)) ;
#106324=CARTESIAN_POINT('',(64.9402651077865,252.844243057664,21.8278816743835)) ;
#106325=CARTESIAN_POINT('Origin',(64.9402651077865,248.040265107786,23.0213203435596)) ;
#106326=CARTESIAN_POINT('',(64.7902651077865,253.021684041655,21.9279469374017)) ;
#106327=CARTESIAN_POINT('Ctrl Pts',(64.9402651077865,252.844243057664,21.8278816743835)) ;
#106328=CARTESIAN_POINT('Ctrl Pts',(64.9402651077865,252.844932736563,21.8282643521316)) ;
#106329=CARTESIAN_POINT('Ctrl Pts',(64.9402617776811,252.845622389192,21.8286470887883)) ;
#106330=CARTESIAN_POINT('Ctrl Pts',(64.9400834366345,252.864083054386,21.8388941738985)) ;
#106331=CARTESIAN_POINT('Ctrl Pts',(64.9376982652987,252.881900097428,21.8488338903424)) ;
#106332=CARTESIAN_POINT('Ctrl Pts',(64.9285249168182,252.915644153157,21.8677473945125)) ;
#106333=CARTESIAN_POINT('Ctrl Pts',(64.9218878905886,252.931768908382,21.8768282252525)) ;
#106334=CARTESIAN_POINT('Ctrl Pts',(64.9030518920066,252.963394691376,21.8947080938071)) ;
#106335=CARTESIAN_POINT('Ctrl Pts',(64.8902415596279,252.978776583803,21.903448367913)) ;
#106336=CARTESIAN_POINT('Ctrl Pts',(64.8622234505159,253.001100194315,21.9161701569215)) ;
#106337=CARTESIAN_POINT('Ctrl Pts',(64.8483068832618,253.009076434455,21.9207300804757)) ;
#106338=CARTESIAN_POINT('Ctrl Pts',(64.8193104176514,253.019163431181,21.9265019586177)) ;
#106339=CARTESIAN_POINT('Ctrl Pts',(64.8049443310404,253.021684041655,21.9279469374017)) ;
#106340=CARTESIAN_POINT('Ctrl Pts',(64.7902651077865,253.021684041655,21.9279469374017)) ;
#106341=CARTESIAN_POINT('Origin',(64.7902651077865,248.040265107786,23.0213203435596)) ;
#106342=CARTESIAN_POINT('Origin',(64.7902651077865,250.752859316469,22.5074134442792)) ;
#106343=CARTESIAN_POINT('',(64.9402651077865,253.360989860305,21.6599804602402)) ;
#106344=CARTESIAN_POINT('',(64.9402651077865,250.752859316469,22.5074134442792)) ;
#106345=CARTESIAN_POINT('',(64.7902651077865,253.403809825024,21.8037867439466)) ;
#106346=CARTESIAN_POINT('Ctrl Pts',(64.9402651077865,253.360989860305,21.6599804602402)) ;
#106347=CARTESIAN_POINT('Ctrl Pts',(64.9402651077865,253.361402751249,21.661379465413)) ;
#106348=CARTESIAN_POINT('Ctrl Pts',(64.940243846551,253.361815739121,21.662778361321)) ;
#106349=CARTESIAN_POINT('Ctrl Pts',(64.9402013305491,253.362228689928,21.6641767026333)) ;
#106350=CARTESIAN_POINT('Ctrl Pts',(64.9396551395108,253.367533752023,21.6821407975691)) ;
#106351=CARTESIAN_POINT('Ctrl Pts',(64.9356062703197,253.372782829414,21.6998433299152)) ;
#106352=CARTESIAN_POINT('Ctrl Pts',(64.928263675975,253.377696511422,21.716368776554)) ;
#106353=CARTESIAN_POINT('Ctrl Pts',(64.9206090302591,253.382819018967,21.73359653467)) ;
#106354=CARTESIAN_POINT('Ctrl Pts',(64.9095180038062,253.387480805045,21.7492226802187)) ;
#106355=CARTESIAN_POINT('Ctrl Pts',(64.8956136387304,253.391409546164,21.7623702561123)) ;
#106356=CARTESIAN_POINT('Ctrl Pts',(64.8817129938792,253.395337236117,21.7755143142665)) ;
#106357=CARTESIAN_POINT('Ctrl Pts',(64.8652664191735,253.39845688034,21.7859297354668)) ;
#106358=CARTESIAN_POINT('Ctrl Pts',(64.8471986491032,253.400585314597,21.7930320573423)) ;
#106359=CARTESIAN_POINT('Ctrl Pts',(64.8291331055125,253.402713486568,21.8001335040033)) ;
#106360=CARTESIAN_POINT('Ctrl Pts',(64.8097925816883,253.403809825025,21.8037867439465)) ;
#106361=CARTESIAN_POINT('Ctrl Pts',(64.7902651077865,253.403809825024,21.8037867439468)) ;
#106362=CARTESIAN_POINT('',(64.7902651077865,250.799211865625,22.6500719217234)) ;
#106363=CARTESIAN_POINT('Origin',(64.7902651077865,253.27107594741,21.3217268744974)) ;
#106364=CARTESIAN_POINT('',(64.9402651077865,253.144997361738,20.9952239032474)) ;
#106365=CARTESIAN_POINT('Origin',(64.9402651077865,253.27107594741,21.3217268744974)) ;
#106366=CARTESIAN_POINT('',(64.7902651077865,253.095112228145,20.8537132320653)) ;
#106367=CARTESIAN_POINT('Ctrl Pts',(64.9402651077865,253.144997361737,20.995223903243)) ;
#106368=CARTESIAN_POINT('Ctrl Pts',(64.9402651077865,253.144509082919,20.9938493930776)) ;
#106369=CARTESIAN_POINT('Ctrl Pts',(64.9402438465509,253.144020946745,20.9924749143332)) ;
#106370=CARTESIAN_POINT('Ctrl Pts',(64.9402013305491,253.143533106564,20.9911009060563)) ;
#106371=CARTESIAN_POINT('Ctrl Pts',(64.9396551395109,253.137265961862,20.9734494107126)) ;
#106372=CARTESIAN_POINT('Ctrl Pts',(64.9356062703199,253.131107267255,20.9560424309125)) ;
#106373=CARTESIAN_POINT('Ctrl Pts',(64.9282636759749,253.125369105682,20.9397848739233)) ;
#106374=CARTESIAN_POINT('Ctrl Pts',(64.9206090302591,253.119387079188,20.9228363904431)) ;
#106375=CARTESIAN_POINT('Ctrl Pts',(64.9095180038061,253.113973725445,20.9074544440316)) ;
#106376=CARTESIAN_POINT('Ctrl Pts',(64.8956136387303,253.109424192564,20.8945085756089)) ;
#106377=CARTESIAN_POINT('Ctrl Pts',(64.881712993879,253.104875876946,20.8815661709571)) ;
#106378=CARTESIAN_POINT('Ctrl Pts',(64.8652664191735,253.101277691159,20.8713062373366)) ;
#106379=CARTESIAN_POINT('Ctrl Pts',(64.8471986491031,253.098824990589,20.8643092759729)) ;
#106380=CARTESIAN_POINT('Ctrl Pts',(64.8291331055122,253.096372592264,20.8573131768402)) ;
#106381=CARTESIAN_POINT('Ctrl Pts',(64.8097925816883,253.095112228145,20.8537132320655)) ;
#106382=CARTESIAN_POINT('Ctrl Pts',(64.7902651077865,253.095112228145,20.8537132320655)) ;
#106383=CARTESIAN_POINT('Origin',(64.7902651077865,253.27107594741,21.3217268744974)) ;
#106384=CARTESIAN_POINT('Origin',(64.7902651077865,250.202412898851,21.9513275530686)) ;
#106385=CARTESIAN_POINT('',(64.9402651077865,252.628250559098,21.1631251173908)) ;
#106386=CARTESIAN_POINT('',(64.9402651077865,250.202412898851,21.9513275530686)) ;
#106387=CARTESIAN_POINT('',(64.7902651077865,252.712986444776,20.9778734255204)) ;
#106388=CARTESIAN_POINT('Ctrl Pts',(64.9402651077865,252.628250559098,21.1631251173908)) ;
#106389=CARTESIAN_POINT('Ctrl Pts',(64.9402651077865,252.628583588709,21.162410141506)) ;
#106390=CARTESIAN_POINT('Ctrl Pts',(64.940261777681,252.628916562446,21.1616951333976)) ;
#106391=CARTESIAN_POINT('Ctrl Pts',(64.9400834366345,252.637828468808,21.1425541606572)) ;
#106392=CARTESIAN_POINT('Ctrl Pts',(64.9376982652988,252.64640034068,21.1240401659929)) ;
#106393=CARTESIAN_POINT('Ctrl Pts',(64.9285249168183,252.662582776404,21.0889045613858)) ;
#106394=CARTESIAN_POINT('Ctrl Pts',(64.9218878905887,252.670290399024,21.0720801216756)) ;
#106395=CARTESIAN_POINT('Ctrl Pts',(64.9030518920067,252.685366671877,21.0390258353215)) ;
#106396=CARTESIAN_POINT('Ctrl Pts',(64.890241559628,252.692673480035,21.0229135555138)) ;
#106397=CARTESIAN_POINT('Ctrl Pts',(64.8622234505159,252.703255980354,20.9994999229698)) ;
#106398=CARTESIAN_POINT('Ctrl Pts',(64.8483068832618,252.707028638362,20.9911225509982)) ;
#106399=CARTESIAN_POINT('Ctrl Pts',(64.8193104176512,252.711796565285,20.9805240155764)) ;
#106400=CARTESIAN_POINT('Ctrl Pts',(64.8049443310403,252.712986444776,20.9778734255205)) ;
#106401=CARTESIAN_POINT('Ctrl Pts',(64.7902651077865,252.712986444776,20.9778734255204)) ;
#106402=CARTESIAN_POINT('',(64.7902651077865,250.156060349694,21.8086690756243)) ;
#106403=CARTESIAN_POINT('Origin',(64.7902651077865,248.040265107786,23.0213203435596)) ;
#106404=CARTESIAN_POINT('',(64.9402651077865,252.240326810636,20.4017818933262)) ;
#106405=CARTESIAN_POINT('Origin',(64.9402651077865,248.040265107786,23.0213203435596)) ;
#106406=CARTESIAN_POINT('',(64.7902651077865,252.440005081538,20.4421173342227)) ;
#106407=CARTESIAN_POINT('Ctrl Pts',(64.9402651077865,252.240326810636,20.4017818933262)) ;
#106408=CARTESIAN_POINT('Ctrl Pts',(64.9402651077865,252.241100988172,20.4019327189915)) ;
#106409=CARTESIAN_POINT('Ctrl Pts',(64.940261777681,252.241875158935,20.402083608801)) ;
#106410=CARTESIAN_POINT('Ctrl Pts',(64.9400834366345,252.262598818301,20.4061245065945)) ;
#106411=CARTESIAN_POINT('Ctrl Pts',(64.9376982652987,252.282615374489,20.4100719695998)) ;
#106412=CARTESIAN_POINT('Ctrl Pts',(64.9285249168184,252.320552472788,20.4176322943072)) ;
#106413=CARTESIAN_POINT('Ctrl Pts',(64.9218878905887,252.33869415734,20.4212858541613)) ;
#106414=CARTESIAN_POINT('Ctrl Pts',(64.9030518920066,252.374297247581,20.4285177152552)) ;
#106415=CARTESIAN_POINT('Ctrl Pts',(64.8902415596279,252.39162718984,20.4320769437325)) ;
#106416=CARTESIAN_POINT('Ctrl Pts',(64.8622234505159,252.416789454087,20.4372777090437)) ;
#106417=CARTESIAN_POINT('Ctrl Pts',(64.8483068832618,252.42578440312,20.4391496602992)) ;
#106418=CARTESIAN_POINT('Ctrl Pts',(64.8193104176514,252.437161315521,20.4415219892068)) ;
#106419=CARTESIAN_POINT('Ctrl Pts',(64.8049443310403,252.440005081538,20.4421173342227)) ;
#106420=CARTESIAN_POINT('Ctrl Pts',(64.7902651077865,252.440005081538,20.4421173342227)) ;
#106421=CARTESIAN_POINT('Origin',(64.7902651077865,248.040265107786,23.0213203435596)) ;
#106422=CARTESIAN_POINT('Origin',(64.7902651077865,250.461289540614,21.6943281289039)) ;
#106423=CARTESIAN_POINT('',(64.9402651077865,252.679897896016,20.0824148057166)) ;
#106424=CARTESIAN_POINT('',(64.9402651077865,250.461289540614,21.6943281289039)) ;
#106425=CARTESIAN_POINT('',(64.7902651077865,252.765060688053,20.2059506121228)) ;
#106426=CARTESIAN_POINT('Ctrl Pts',(64.9402651077865,252.679897896016,20.0824148057166)) ;
#106427=CARTESIAN_POINT('Ctrl Pts',(64.9402651077865,252.680722895012,20.0836177483836)) ;
#106428=CARTESIAN_POINT('Ctrl Pts',(64.940243846551,252.681547952431,20.0848205571807)) ;
#106429=CARTESIAN_POINT('Ctrl Pts',(64.9402013305491,252.682372803215,20.086022849981)) ;
#106430=CARTESIAN_POINT('Ctrl Pts',(64.9396551395108,252.692969427699,20.1014683651929)) ;
#106431=CARTESIAN_POINT('Ctrl Pts',(64.9356062703198,252.703431980308,20.1166824198099)) ;
#106432=CARTESIAN_POINT('Ctrl Pts',(64.9282636759749,252.713211813451,20.1308806422754)) ;
#106433=CARTESIAN_POINT('Ctrl Pts',(64.9206090302592,252.723407277664,20.1456822720077)) ;
#106434=CARTESIAN_POINT('Ctrl Pts',(64.9095180038062,252.732669644223,20.1591030484337)) ;
#106435=CARTESIAN_POINT('Ctrl Pts',(64.8956136387303,252.740468923451,20.1703930883885)) ;
#106436=CARTESIAN_POINT('Ctrl Pts',(64.881712993879,252.74826611592,20.1816801076024)) ;
#106437=CARTESIAN_POINT('Ctrl Pts',(64.8652664191735,252.75445161604,20.1906217387244)) ;
#106438=CARTESIAN_POINT('Ctrl Pts',(64.8471986491032,252.758670615469,20.1967187258679)) ;
#106439=CARTESIAN_POINT('Ctrl Pts',(64.8291331055124,252.762889094993,20.2028149616837)) ;
#106440=CARTESIAN_POINT('Ctrl Pts',(64.8097925816883,252.765060688053,20.2059506121227)) ;
#106441=CARTESIAN_POINT('Ctrl Pts',(64.7902651077865,252.765060688053,20.2059506121227)) ;
#106442=CARTESIAN_POINT('',(64.7902651077865,250.549457328458,21.8156806780601)) ;
#106443=CARTESIAN_POINT('Origin',(64.7902651077865,252.489858576849,19.788501455951)) ;
#106444=CARTESIAN_POINT('',(64.9402651077865,252.26905574955,19.5169391031533)) ;
#106445=CARTESIAN_POINT('Origin',(64.9402651077865,252.489858576849,19.788501455951)) ;
#106446=CARTESIAN_POINT('',(64.7902651077865,252.1778829659,19.3977698112471)) ;
#106447=CARTESIAN_POINT('Ctrl Pts',(64.9402651077865,252.269055749548,19.5169391031502)) ;
#106448=CARTESIAN_POINT('Ctrl Pts',(64.9402651077865,252.268166621797,19.5157827527532)) ;
#106449=CARTESIAN_POINT('Ctrl Pts',(64.9402438465509,252.267277639417,19.5146263881596)) ;
#106450=CARTESIAN_POINT('Ctrl Pts',(64.9402013305491,252.266389083925,19.5134703795409)) ;
#106451=CARTESIAN_POINT('Ctrl Pts',(64.9396551395109,252.25497406308,19.498619464092)) ;
#106452=CARTESIAN_POINT('Ctrl Pts',(64.9356062703198,252.243737743863,19.4839675838203)) ;
#106453=CARTESIAN_POINT('Ctrl Pts',(64.9282636759749,252.233256566511,19.4702789177493)) ;
#106454=CARTESIAN_POINT('Ctrl Pts',(64.9206090302592,252.222329951809,19.4560084999417)) ;
#106455=CARTESIAN_POINT('Ctrl Pts',(64.9095180038061,252.212428263609,19.4430522178766)) ;
#106456=CARTESIAN_POINT('Ctrl Pts',(64.8956136387303,252.204100907367,19.4321458483308)) ;
#106457=CARTESIAN_POINT('Ctrl Pts',(64.881712993879,252.195775779175,19.4212423968718)) ;
#106458=CARTESIAN_POINT('Ctrl Pts',(64.8652664191735,252.189183207286,19.4125965207019)) ;
#106459=CARTESIAN_POINT('Ctrl Pts',(64.8471986491031,252.184688370457,19.4066999411606)) ;
#106460=CARTESIAN_POINT('Ctrl Pts',(64.8291331055122,252.180194087523,19.4008040882511)) ;
#106461=CARTESIAN_POINT('Ctrl Pts',(64.8097925816882,252.177882965899,19.3977698112477)) ;
#106462=CARTESIAN_POINT('Ctrl Pts',(64.7902651077865,252.177882965899,19.3977698112476)) ;
#106463=CARTESIAN_POINT('Origin',(64.7902651077865,252.489858576849,19.788501455951)) ;
#106464=CARTESIAN_POINT('Origin',(64.7902651077865,249.765943897551,21.3355563159851)) ;
#106465=CARTESIAN_POINT('',(64.9402651077865,251.829484664171,19.836306190763)) ;
#106466=CARTESIAN_POINT('',(64.9402651077865,249.765943897551,21.3355563159851)) ;
#106467=CARTESIAN_POINT('',(64.7902651077865,251.852827359384,19.6339365333471)) ;
#106468=CARTESIAN_POINT('Ctrl Pts',(64.9402651077865,251.829484664171,19.836306190763)) ;
#106469=CARTESIAN_POINT('Ctrl Pts',(64.9402651077865,251.829580454454,19.8355232964791)) ;
#106470=CARTESIAN_POINT('Ctrl Pts',(64.940261777681,251.82967618164,19.8347403888152)) ;
#106471=CARTESIAN_POINT('Ctrl Pts',(64.9400834366345,251.832237022392,19.8137823114442)) ;
#106472=CARTESIAN_POINT('Ctrl Pts',(64.9376982652988,251.834668218008,19.7935256020938)) ;
#106473=CARTESIAN_POINT('Ctrl Pts',(64.9285249168184,251.839201130021,19.7551090087292)) ;
#106474=CARTESIAN_POINT('Ctrl Pts',(64.9218878905887,251.841332476948,19.7367262293339)) ;
#106475=CARTESIAN_POINT('Ctrl Pts',(64.9030518920067,251.845456528266,19.7006309103819)) ;
#106476=CARTESIAN_POINT('Ctrl Pts',(64.890241559628,251.847426747499,19.683049293783)) ;
#106477=CARTESIAN_POINT('Ctrl Pts',(64.8622234505158,251.85025609303,19.6575114335403)) ;
#106478=CARTESIAN_POINT('Ctrl Pts',(64.8483068832618,251.851255353705,19.648378263899)) ;
#106479=CARTESIAN_POINT('Ctrl Pts',(64.8193104176512,251.852514794114,19.6368250872756)) ;
#106480=CARTESIAN_POINT('Ctrl Pts',(64.8049443310403,251.852827359384,19.6339365333471)) ;
#106481=CARTESIAN_POINT('Ctrl Pts',(64.7902651077865,251.852827359384,19.6339365333471)) ;
#106482=CARTESIAN_POINT('',(64.7902651077865,249.677776109707,21.2142037668289)) ;
#106483=CARTESIAN_POINT('Origin',(64.7902651077865,248.040265107786,23.0213203435596)) ;
#106484=CARTESIAN_POINT('',(64.9402651077865,251.225279260583,19.2321007871753)) ;
#106485=CARTESIAN_POINT('Origin',(64.9402651077865,248.040265107786,23.0213203435596)) ;
#106486=CARTESIAN_POINT('',(64.7902651077865,251.427648917999,19.2087580919617)) ;
#106487=CARTESIAN_POINT('Ctrl Pts',(64.9402651077865,251.225279260583,19.2321007871753)) ;
#106488=CARTESIAN_POINT('Ctrl Pts',(64.9402651077865,251.226062154865,19.2320049968921)) ;
#106489=CARTESIAN_POINT('Ctrl Pts',(64.940261777681,251.226845062528,19.2319092697067)) ;
#106490=CARTESIAN_POINT('Ctrl Pts',(64.9400834366348,251.247803139899,19.2293484289549)) ;
#106491=CARTESIAN_POINT('Ctrl Pts',(64.9376982652993,251.268059849249,19.2269172333384)) ;
#106492=CARTESIAN_POINT('Ctrl Pts',(64.9285249168188,251.306476442616,19.2223843213247)) ;
#106493=CARTESIAN_POINT('Ctrl Pts',(64.921887890589,251.324859222011,19.2202529743981)) ;
#106494=CARTESIAN_POINT('Ctrl Pts',(64.9030518920067,251.360954540964,19.2161289230798)) ;
#106495=CARTESIAN_POINT('Ctrl Pts',(64.890241559628,251.378536157563,19.2141587038466)) ;
#106496=CARTESIAN_POINT('Ctrl Pts',(64.8622234505159,251.404074017806,19.211329358316)) ;
#106497=CARTESIAN_POINT('Ctrl Pts',(64.8483068832618,251.413207187447,19.2103300976412)) ;
#106498=CARTESIAN_POINT('Ctrl Pts',(64.8193104176513,251.42476036407,19.2090706572321)) ;
#106499=CARTESIAN_POINT('Ctrl Pts',(64.8049443310403,251.427648917999,19.2087580919617)) ;
#106500=CARTESIAN_POINT('Ctrl Pts',(64.7902651077865,251.427648917999,19.2087580919617)) ;
#106501=CARTESIAN_POINT('Origin',(64.7902651077865,248.040265107786,23.0213203435596)) ;
#106502=CARTESIAN_POINT('Origin',(64.7902651077865,249.932733025005,21.0111380571975)) ;
#106503=CARTESIAN_POINT('',(64.9402651077865,251.544646348193,18.792529701796)) ;
#106504=CARTESIAN_POINT('',(64.9402651077865,249.932733025005,21.0111380571975)) ;
#106505=CARTESIAN_POINT('',(64.7902651077865,251.663815640099,18.8837024854464)) ;
#106506=CARTESIAN_POINT('Ctrl Pts',(64.9402651077865,251.544646348193,18.792529701796)) ;
#106507=CARTESIAN_POINT('Ctrl Pts',(64.9402651077865,251.545802698591,18.7934188295481)) ;
#106508=CARTESIAN_POINT('Ctrl Pts',(64.940243846551,251.546959063185,18.7943078119284)) ;
#106509=CARTESIAN_POINT('Ctrl Pts',(64.9402013305491,251.548115071805,18.7951963674209)) ;
#106510=CARTESIAN_POINT('Ctrl Pts',(64.9396551395109,251.562965987255,18.8066113882653)) ;
#106511=CARTESIAN_POINT('Ctrl Pts',(64.93560627032,251.577617867525,18.817847707483)) ;
#106512=CARTESIAN_POINT('Ctrl Pts',(64.928263675975,251.591306533596,18.8283288848357)) ;
#106513=CARTESIAN_POINT('Ctrl Pts',(64.9206090302591,251.605576951404,18.8392554995375)) ;
#106514=CARTESIAN_POINT('Ctrl Pts',(64.9095180038063,251.618533233469,18.8491571877368)) ;
#106515=CARTESIAN_POINT('Ctrl Pts',(64.8956136387304,251.629439603015,18.8574845439795)) ;
#106516=CARTESIAN_POINT('Ctrl Pts',(64.881712993879,251.640343054474,18.8658096721712)) ;
#106517=CARTESIAN_POINT('Ctrl Pts',(64.8652664191734,251.648988930644,18.8724022440602)) ;
#106518=CARTESIAN_POINT('Ctrl Pts',(64.8471986491031,251.654885510185,18.8768970808899)) ;
#106519=CARTESIAN_POINT('Ctrl Pts',(64.8291331055123,251.660781363094,18.8813913638239)) ;
#106520=CARTESIAN_POINT('Ctrl Pts',(64.8097925816882,251.663815640099,18.8837024854465)) ;
#106521=CARTESIAN_POINT('Ctrl Pts',(64.7902651077865,251.663815640099,18.8837024854463)) ;
#106522=CARTESIAN_POINT('',(64.7902651077865,250.054085574161,21.0993058450414)) ;
#106523=CARTESIAN_POINT('Origin',(64.7902651077865,251.273083995395,18.5717268744974)) ;
#106524=CARTESIAN_POINT('',(64.9402651077865,250.979170645629,18.38168755533)) ;
#106525=CARTESIAN_POINT('Origin',(64.9402651077865,251.273083995395,18.5717268744974)) ;
#106526=CARTESIAN_POINT('',(64.7902651077865,250.855634839223,18.2965247632928)) ;
#106527=CARTESIAN_POINT('Ctrl Pts',(64.9402651077865,250.979170645627,18.381687555328)) ;
#106528=CARTESIAN_POINT('Ctrl Pts',(64.9402651077865,250.97796770296,18.3808625563329)) ;
#106529=CARTESIAN_POINT('Ctrl Pts',(64.9402438465509,250.976764894164,18.3800374989153)) ;
#106530=CARTESIAN_POINT('Ctrl Pts',(64.9402013305491,250.975562601365,18.3792126481319)) ;
#106531=CARTESIAN_POINT('Ctrl Pts',(64.9396551395108,250.960117086155,18.3686160236418)) ;
#106532=CARTESIAN_POINT('Ctrl Pts',(64.9356062703197,250.944903031536,18.3581534710383)) ;
#106533=CARTESIAN_POINT('Ctrl Pts',(64.9282636759749,250.930704809071,18.3483736378949)) ;
#106534=CARTESIAN_POINT('Ctrl Pts',(64.920609030259,250.915903179338,18.3381781736819)) ;
#106535=CARTESIAN_POINT('Ctrl Pts',(64.9095180038059,250.902482402912,18.3289158071228)) ;
#106536=CARTESIAN_POINT('Ctrl Pts',(64.8956136387303,250.891192362958,18.3211165278944)) ;
#106537=CARTESIAN_POINT('Ctrl Pts',(64.8817129938791,250.879905343744,18.3133193354259)) ;
#106538=CARTESIAN_POINT('Ctrl Pts',(64.8652664191733,250.870963712621,18.3071338353064)) ;
#106539=CARTESIAN_POINT('Ctrl Pts',(64.847198649103,250.864866725478,18.3029148358775)) ;
#106540=CARTESIAN_POINT('Ctrl Pts',(64.8291331055123,250.858770489662,18.2986963563531)) ;
#106541=CARTESIAN_POINT('Ctrl Pts',(64.8097925816882,250.855634839223,18.2965247632931)) ;
#106542=CARTESIAN_POINT('Ctrl Pts',(64.7902651077865,250.855634839223,18.2965247632931)) ;
#106543=CARTESIAN_POINT('Origin',(64.7902651077865,251.273083995395,18.5717268744974)) ;
#106544=CARTESIAN_POINT('Origin',(64.7902651077865,249.160553432798,20.8847994073294)) ;
#106545=CARTESIAN_POINT('',(64.9402651077865,250.65980355802,18.8212586407095)) ;
#106546=CARTESIAN_POINT('',(64.9402651077865,249.160553432798,20.8847994073294)) ;
#106547=CARTESIAN_POINT('',(64.7902651077865,250.619468117123,18.6215803698081)) ;
#106548=CARTESIAN_POINT('Ctrl Pts',(64.9402651077865,250.65980355802,18.8212586407095)) ;
#106549=CARTESIAN_POINT('Ctrl Pts',(64.9402651077865,250.659652732354,18.8204844631737)) ;
#106550=CARTESIAN_POINT('Ctrl Pts',(64.940261777681,250.659501842545,18.8197102924112)) ;
#106551=CARTESIAN_POINT('Ctrl Pts',(64.9400834366345,250.655460944751,18.7989866330446)) ;
#106552=CARTESIAN_POINT('Ctrl Pts',(64.9376982652987,250.651513481746,18.7789700768574)) ;
#106553=CARTESIAN_POINT('Ctrl Pts',(64.9285249168183,250.643953157039,18.7410329785579)) ;
#106554=CARTESIAN_POINT('Ctrl Pts',(64.9218878905886,250.640299597185,18.7228912940054)) ;
#106555=CARTESIAN_POINT('Ctrl Pts',(64.9030518920067,250.633067736091,18.6872882037656)) ;
#106556=CARTESIAN_POINT('Ctrl Pts',(64.890241559628,250.629508507613,18.6699582615064)) ;
#106557=CARTESIAN_POINT('Ctrl Pts',(64.8622234505159,250.624307742302,18.6447959972585)) ;
#106558=CARTESIAN_POINT('Ctrl Pts',(64.8483068832618,250.622435791047,18.6358010482263)) ;
#106559=CARTESIAN_POINT('Ctrl Pts',(64.8193104176513,250.620063462139,18.6244241358249)) ;
#106560=CARTESIAN_POINT('Ctrl Pts',(64.8049443310403,250.619468117123,18.6215803698081)) ;
#106561=CARTESIAN_POINT('Ctrl Pts',(64.7902651077865,250.619468117123,18.6215803698081)) ;
#106562=CARTESIAN_POINT('',(64.7902651077865,249.039200883641,20.7966316194855)) ;
#106563=CARTESIAN_POINT('Origin',(64.7902651077865,248.040265107786,23.0213203435596)) ;
#106564=CARTESIAN_POINT('',(64.9402651077865,249.898460333955,18.4333348922484)) ;
#106565=CARTESIAN_POINT('Origin',(64.9402651077865,248.040265107786,23.0213203435596)) ;
#106566=CARTESIAN_POINT('',(64.7902651077865,250.083712025826,18.3485990065702)) ;
#106567=CARTESIAN_POINT('Ctrl Pts',(64.9402651077865,249.898460333955,18.4333348922483)) ;
#106568=CARTESIAN_POINT('Ctrl Pts',(64.9402651077865,249.899175309839,18.4330018626366)) ;
#106569=CARTESIAN_POINT('Ctrl Pts',(64.940261777681,249.899890317948,18.4326688888998)) ;
#106570=CARTESIAN_POINT('Ctrl Pts',(64.9400834366345,249.91903129069,18.4237569825383)) ;
#106571=CARTESIAN_POINT('Ctrl Pts',(64.9376982652987,249.937545285353,18.4151851106656)) ;
#106572=CARTESIAN_POINT('Ctrl Pts',(64.9285249168183,249.97268088996,18.3990026749418)) ;
#106573=CARTESIAN_POINT('Ctrl Pts',(64.9218878905886,249.98950532967,18.3912950523219)) ;
#106574=CARTESIAN_POINT('Ctrl Pts',(64.9030518920067,250.022559616024,18.3762187794687)) ;
#106575=CARTESIAN_POINT('Ctrl Pts',(64.890241559628,250.038671895832,18.3689119713107)) ;
#106576=CARTESIAN_POINT('Ctrl Pts',(64.8622234505159,250.062085528376,18.3583294709921)) ;
#106577=CARTESIAN_POINT('Ctrl Pts',(64.8483068832618,250.070462900348,18.3545568129842)) ;
#106578=CARTESIAN_POINT('Ctrl Pts',(64.8193104176513,250.08106143577,18.3497888860605)) ;
#106579=CARTESIAN_POINT('Ctrl Pts',(64.8049443310403,250.083712025826,18.3485990065702)) ;
#106580=CARTESIAN_POINT('Ctrl Pts',(64.7902651077865,250.083712025826,18.3485990065702)) ;
#106581=CARTESIAN_POINT('Origin',(64.7902651077865,248.040265107786,23.0213203435596)) ;
#106582=CARTESIAN_POINT('Origin',(64.7902651077865,249.21892856406,20.5247186334439)) ;
#106583=CARTESIAN_POINT('',(64.7902651077865,250.207872219281,17.9664732232009)) ;
#106584=CARTESIAN_POINT('',(64.7902651077865,249.361587041504,20.5710711826001)) ;
#106585=CARTESIAN_POINT('',(64.9402651077865,250.066361548099,17.9165880896075)) ;
#106586=CARTESIAN_POINT('',(64.9402651077865,249.21892856406,20.5247186334439)) ;
#106587=CARTESIAN_POINT('Ctrl Pts',(64.9402651077865,250.066361548099,17.9165880896075)) ;
#106588=CARTESIAN_POINT('Ctrl Pts',(64.9402651077865,250.067736058266,17.9170763684256)) ;
#106589=CARTESIAN_POINT('Ctrl Pts',(64.940243846551,250.069110537011,17.9175645046006)) ;
#106590=CARTESIAN_POINT('Ctrl Pts',(64.9402013305492,250.07048454529,17.9180523447822)) ;
#106591=CARTESIAN_POINT('Ctrl Pts',(64.939655139511,250.088136040637,17.9243194894782)) ;
#106592=CARTESIAN_POINT('Ctrl Pts',(64.9356062703199,250.105543020433,17.9304781840933)) ;
#106593=CARTESIAN_POINT('Ctrl Pts',(64.9282636759752,250.121800577422,17.9362163456661)) ;
#106594=CARTESIAN_POINT('Ctrl Pts',(64.9206090302596,250.138749060902,17.9421983721593)) ;
#106595=CARTESIAN_POINT('Ctrl Pts',(64.9095180038067,250.154131007314,17.9476117259011)) ;
#106596=CARTESIAN_POINT('Ctrl Pts',(64.8956136387307,250.167076875737,17.9521612587827)) ;
#106597=CARTESIAN_POINT('Ctrl Pts',(64.8817129938793,250.180019280389,17.9567095744003)) ;
#106598=CARTESIAN_POINT('Ctrl Pts',(64.8652664191736,250.19027921401,17.9603077601869)) ;
#106599=CARTESIAN_POINT('Ctrl Pts',(64.8471986491033,250.197276175374,17.9627604607567)) ;
#106600=CARTESIAN_POINT('Ctrl Pts',(64.8291331055124,250.204272274506,17.9652128590818)) ;
#106601=CARTESIAN_POINT('Ctrl Pts',(64.8097925816883,250.207872219281,17.9664732232008)) ;
#106602=CARTESIAN_POINT('Ctrl Pts',(64.7902651077865,250.207872219281,17.9664732232008)) ;
#106603=CARTESIAN_POINT('Origin',(64.7902651077865,249.739858576849,17.7905095039363)) ;
#106604=CARTESIAN_POINT('',(64.7902651077865,249.257798707399,17.6577756263215)) ;
#106605=CARTESIAN_POINT('Origin',(64.7902651077865,249.739858576849,17.7905095039363)) ;
#106606=CARTESIAN_POINT('',(64.9402651077865,249.401604991106,17.7005955910415)) ;
#106607=CARTESIAN_POINT('Origin',(64.9402651077865,249.739858576849,17.7905095039363)) ;
#106608=CARTESIAN_POINT('Ctrl Pts',(64.9402651077865,249.401604991096,17.7005955910383)) ;
#106609=CARTESIAN_POINT('Ctrl Pts',(64.9402651077864,249.400205985927,17.7001827000958)) ;
#106610=CARTESIAN_POINT('Ctrl Pts',(64.9402438465509,249.398807090022,17.699769712222)) ;
#106611=CARTESIAN_POINT('Ctrl Pts',(64.9402013305491,249.397408748713,17.6993567614174)) ;
#106612=CARTESIAN_POINT('Ctrl Pts',(64.9396551395108,249.379444653775,17.694051699333)) ;
#106613=CARTESIAN_POINT('Ctrl Pts',(64.9356062703196,249.361742121431,17.6888026219303)) ;
#106614=CARTESIAN_POINT('Ctrl Pts',(64.9282636759748,249.345216674792,17.683888939923)) ;
#106615=CARTESIAN_POINT('Ctrl Pts',(64.9206090302589,249.327988916676,17.6787664323787)) ;
#106616=CARTESIAN_POINT('Ctrl Pts',(64.9095180038059,249.312362771127,17.6741046463012)) ;
#106617=CARTESIAN_POINT('Ctrl Pts',(64.8956136387303,249.299215195234,17.6701759051819)) ;
#106618=CARTESIAN_POINT('Ctrl Pts',(64.8817129938792,249.28607113708,17.6662482152289)) ;
#106619=CARTESIAN_POINT('Ctrl Pts',(64.8652664191736,249.275655715879,17.663128571007)) ;
#106620=CARTESIAN_POINT('Ctrl Pts',(64.8471986491032,249.268553394004,17.6610001367496)) ;
#106621=CARTESIAN_POINT('Ctrl Pts',(64.8291331055123,249.261451947343,17.6588719647777)) ;
#106622=CARTESIAN_POINT('Ctrl Pts',(64.8097925816883,249.257798707399,17.6577756263226)) ;
#106623=CARTESIAN_POINT('Ctrl Pts',(64.7902651077865,249.257798707399,17.6577756263226)) ;
#106624=CARTESIAN_POINT('Origin',(64.7902651077865,248.445501341285,20.6431800539285)) ;
#106625=CARTESIAN_POINT('',(64.7902651077865,249.133638513944,18.0399014096908)) ;
#106626=CARTESIAN_POINT('',(64.7902651077865,248.30284286384,20.5968275047722)) ;
#106627=CARTESIAN_POINT('',(64.9402651077865,249.233703776962,18.2173423936815)) ;
#106628=CARTESIAN_POINT('',(64.9402651077865,248.445501341285,20.6431800539285)) ;
#106629=CARTESIAN_POINT('Ctrl Pts',(64.9402651077865,249.233703776962,18.2173423936815)) ;
#106630=CARTESIAN_POINT('Ctrl Pts',(64.9402651077865,249.233321099215,18.2166527147851)) ;
#106631=CARTESIAN_POINT('Ctrl Pts',(64.940261777681,249.232938362557,18.2159630621521)) ;
#106632=CARTESIAN_POINT('Ctrl Pts',(64.9400834366345,249.222691277449,18.197502396961)) ;
#106633=CARTESIAN_POINT('Ctrl Pts',(64.9376982652987,249.212751561004,18.1796853539185)) ;
#106634=CARTESIAN_POINT('Ctrl Pts',(64.9285249168183,249.193838056834,18.1459412981892)) ;
#106635=CARTESIAN_POINT('Ctrl Pts',(64.9218878905887,249.184757226094,18.1298165429637)) ;
#106636=CARTESIAN_POINT('Ctrl Pts',(64.9030518920067,249.166877357539,18.0981907599697)) ;
#106637=CARTESIAN_POINT('Ctrl Pts',(64.890241559628,249.158137083433,18.0828088675435)) ;
#106638=CARTESIAN_POINT('Ctrl Pts',(64.8622234505158,249.145415294424,18.0604852570307)) ;
#106639=CARTESIAN_POINT('Ctrl Pts',(64.8483068832618,249.14085537087,18.0525090168905)) ;
#106640=CARTESIAN_POINT('Ctrl Pts',(64.8193104176514,249.135083492728,18.0424220201646)) ;
#106641=CARTESIAN_POINT('Ctrl Pts',(64.8049443310403,249.133638513944,18.0399014096908)) ;
#106642=CARTESIAN_POINT('Ctrl Pts',(64.7902651077865,249.133638513944,18.0399014096908)) ;
#106643=CARTESIAN_POINT('Origin',(64.7902651077865,248.040265107786,23.0213203435596)) ;
#106644=CARTESIAN_POINT('',(64.7902651077865,248.539748311783,17.9458384424072)) ;
#106645=CARTESIAN_POINT('Origin',(64.7902651077865,248.040265107786,23.0213203435596)) ;
#106646=CARTESIAN_POINT('',(64.9402651077865,248.389748311783,18.0836729796702)) ;
#106647=CARTESIAN_POINT('Origin',(64.9402651077865,248.040265107786,23.0213203435596)) ;
#106648=CARTESIAN_POINT('Ctrl Pts',(64.9402651077865,248.389748311783,18.0836729796702)) ;
#106649=CARTESIAN_POINT('Ctrl Pts',(64.9402651077865,248.390325382448,18.0831353099878)) ;
#106650=CARTESIAN_POINT('Ctrl Pts',(64.940261777681,248.390902501026,18.0825976834882)) ;
#106651=CARTESIAN_POINT('Ctrl Pts',(64.9400834366341,248.406352717363,18.0682070710039)) ;
#106652=CARTESIAN_POINT('Ctrl Pts',(64.9376982652983,248.421311718547,18.0543335974184)) ;
#106653=CARTESIAN_POINT('Ctrl Pts',(64.9285249168178,248.449727016613,18.0280856875433)) ;
#106654=CARTESIAN_POINT('Ctrl Pts',(64.9218878905883,248.463346223256,18.0155562650348)) ;
#106655=CARTESIAN_POINT('Ctrl Pts',(64.9030518920067,248.490123893161,17.9910035412764)) ;
#106656=CARTESIAN_POINT('Ctrl Pts',(64.890241559628,248.503189653969,17.9790753854858)) ;
#106657=CARTESIAN_POINT('Ctrl Pts',(64.8622234505158,248.522187169328,17.9617756192428)) ;
#106658=CARTESIAN_POINT('Ctrl Pts',(64.8483068832618,248.528988708093,17.9555988579533)) ;
#106659=CARTESIAN_POINT('Ctrl Pts',(64.8193104176513,248.537595143822,17.9477891624225)) ;
#106660=CARTESIAN_POINT('Ctrl Pts',(64.8049443310403,248.539748311783,17.9458384424072)) ;
#106661=CARTESIAN_POINT('Ctrl Pts',(64.7902651077865,248.539748311783,17.9458384424072)) ;
#106662=CARTESIAN_POINT('Origin',(64.7902651077865,248.389748311783,20.2826839799233)) ;
#106663=CARTESIAN_POINT('',(64.7902651077865,248.539748311783,17.5440476162869)) ;
#106664=CARTESIAN_POINT('',(64.7902651077865,248.539748311783,20.2826839799233)) ;
#106665=CARTESIAN_POINT('',(64.9402651077865,248.389748311783,17.5403332371978)) ;
#106666=CARTESIAN_POINT('',(64.9402651077865,248.389748311783,20.2826839799233)) ;
#106667=CARTESIAN_POINT('Ctrl Pts',(64.9402651077865,248.389748311783,17.5403332371978)) ;
#106668=CARTESIAN_POINT('Ctrl Pts',(64.9402651077865,248.391206435086,17.5403728709491)) ;
#106669=CARTESIAN_POINT('Ctrl Pts',(64.940243846551,248.392664484427,17.5404123787478)) ;
#106670=CARTESIAN_POINT('Ctrl Pts',(64.9402013305492,248.394121994861,17.5404517504229)) ;
#106671=CARTESIAN_POINT('Ctrl Pts',(64.939655139511,248.412846218751,17.5409575471863)) ;
#106672=CARTESIAN_POINT('Ctrl Pts',(64.9356062703198,248.431304381614,17.5414357612545)) ;
#106673=CARTESIAN_POINT('Ctrl Pts',(64.9282636759751,248.44853942657,17.5418692158132)) ;
#106674=CARTESIAN_POINT('Ctrl Pts',(64.9206090302595,248.466506940072,17.5423210916659)) ;
#106675=CARTESIAN_POINT('Ctrl Pts',(64.9095180038066,248.482808858743,17.5427162141691)) ;
#106676=CARTESIAN_POINT('Ctrl Pts',(64.8956136387307,248.496526994243,17.5430425837127)) ;
#106677=CARTESIAN_POINT('Ctrl Pts',(64.8817129938794,248.510241459345,17.5433688659336)) ;
#106678=CARTESIAN_POINT('Ctrl Pts',(64.8652664191738,248.521111136629,17.5436204501224)) ;
#106679=CARTESIAN_POINT('Ctrl Pts',(64.8471986491034,248.528523568487,17.5437909270114)) ;
#106680=CARTESIAN_POINT('Ctrl Pts',(64.8291331055125,248.535935086915,17.5439613828926)) ;
#106681=CARTESIAN_POINT('Ctrl Pts',(64.8097925816883,248.539748311783,17.5440476162861)) ;
#106682=CARTESIAN_POINT('Ctrl Pts',(64.7902651077865,248.539748311783,17.5440476162861)) ;
#106683=CARTESIAN_POINT('Origin',(64.7902651077865,248.040265107786,17.5213203435596)) ;
#106684=CARTESIAN_POINT('',(64.7902651077865,247.54078190379,17.5440476162869)) ;
#106685=CARTESIAN_POINT('Origin',(64.7902651077865,248.040265107786,17.5213203435596)) ;
#106686=CARTESIAN_POINT('',(64.9402651077865,247.69078190379,17.5403332371979)) ;
#106687=CARTESIAN_POINT('Origin',(64.9402651077865,248.040265107786,17.5213203435596)) ;
#106688=CARTESIAN_POINT('Ctrl Pts',(64.9402651077865,247.69078190379,17.5403332371979)) ;
#106689=CARTESIAN_POINT('Ctrl Pts',(64.9402651077865,247.689323780486,17.5403728709491)) ;
#106690=CARTESIAN_POINT('Ctrl Pts',(64.940243846551,247.687865731145,17.5404123787479)) ;
#106691=CARTESIAN_POINT('Ctrl Pts',(64.9402013305491,247.686408220711,17.540451750423)) ;
#106692=CARTESIAN_POINT('Ctrl Pts',(64.9396551395109,247.667683996822,17.5409575471857)) ;
#106693=CARTESIAN_POINT('Ctrl Pts',(64.9356062703199,247.649225833959,17.5414357612546)) ;
#106694=CARTESIAN_POINT('Ctrl Pts',(64.928263675975,247.631990789003,17.5418692158132)) ;
#106695=CARTESIAN_POINT('Ctrl Pts',(64.9206090302591,247.6140232755,17.5423210916658)) ;
#106696=CARTESIAN_POINT('Ctrl Pts',(64.9095180038062,247.597721356829,17.5427162141691)) ;
#106697=CARTESIAN_POINT('Ctrl Pts',(64.8956136387305,247.58400322133,17.5430425837128)) ;
#106698=CARTESIAN_POINT('Ctrl Pts',(64.8817129938794,247.570288756228,17.5433688659337)) ;
#106699=CARTESIAN_POINT('Ctrl Pts',(64.8652664191737,247.559419078944,17.5436204501225)) ;
#106700=CARTESIAN_POINT('Ctrl Pts',(64.8471986491032,247.552006647086,17.5437909270115)) ;
#106701=CARTESIAN_POINT('Ctrl Pts',(64.8291331055122,247.544595128658,17.5439613828928)) ;
#106702=CARTESIAN_POINT('Ctrl Pts',(64.8097925816883,247.54078190379,17.5440476162862)) ;
#106703=CARTESIAN_POINT('Ctrl Pts',(64.7902651077865,247.54078190379,17.5440476162862)) ;
#106704=CARTESIAN_POINT('Origin',(64.7902651077865,247.69078190379,20.6343496415544)) ;
#106705=CARTESIAN_POINT('',(64.7902651077865,247.54078190379,17.9458384424072)) ;
#106706=CARTESIAN_POINT('',(64.7902651077865,247.54078190379,20.6343496415544)) ;
#106707=CARTESIAN_POINT('',(64.9402651077865,247.69078190379,18.0836729796702)) ;
#106708=CARTESIAN_POINT('',(64.9402651077865,247.69078190379,20.6343496415544)) ;
#106709=CARTESIAN_POINT('Ctrl Pts',(64.9402651077865,247.69078190379,18.0836729796702)) ;
#106710=CARTESIAN_POINT('Ctrl Pts',(64.9402651077865,247.690204833124,18.0831353099878)) ;
#106711=CARTESIAN_POINT('Ctrl Pts',(64.940261777681,247.689627714546,18.0825976834882)) ;
#106712=CARTESIAN_POINT('Ctrl Pts',(64.9400834366341,247.674177498209,18.0682070710039)) ;
#106713=CARTESIAN_POINT('Ctrl Pts',(64.9376982652983,247.659218497025,18.0543335974184)) ;
#106714=CARTESIAN_POINT('Ctrl Pts',(64.9285249168178,247.63080319896,18.0280856875433)) ;
#106715=CARTESIAN_POINT('Ctrl Pts',(64.9218878905883,247.617183992317,18.0155562650348)) ;
#106716=CARTESIAN_POINT('Ctrl Pts',(64.9030518920067,247.590406322412,17.9910035412764)) ;
#106717=CARTESIAN_POINT('Ctrl Pts',(64.890241559628,247.577340561604,17.9790753854858)) ;
#106718=CARTESIAN_POINT('Ctrl Pts',(64.8622234505159,247.558343046244,17.9617756192428)) ;
#106719=CARTESIAN_POINT('Ctrl Pts',(64.8483068832618,247.55154150748,17.9555988579533)) ;
#106720=CARTESIAN_POINT('Ctrl Pts',(64.8193104176513,247.542935071751,17.9477891624225)) ;
#106721=CARTESIAN_POINT('Ctrl Pts',(64.8049443310403,247.54078190379,17.9458384424072)) ;
#106722=CARTESIAN_POINT('Ctrl Pts',(64.7902651077865,247.54078190379,17.9458384424072)) ;
#106723=CARTESIAN_POINT('Origin',(64.7902651077865,248.040265107786,23.0213203435596)) ;
#106724=CARTESIAN_POINT('',(64.7902651077865,246.946891701628,18.0399014096908)) ;
#106725=CARTESIAN_POINT('Origin',(64.7902651077865,248.040265107786,23.0213203435596)) ;
#106726=CARTESIAN_POINT('',(64.9402651077865,246.84682643861,18.2173423936815)) ;
#106727=CARTESIAN_POINT('Origin',(64.9402651077865,248.040265107786,23.0213203435596)) ;
#106728=CARTESIAN_POINT('Ctrl Pts',(64.9402651077865,246.84682643861,18.2173423936815)) ;
#106729=CARTESIAN_POINT('Ctrl Pts',(64.9402651077865,246.847209116358,18.2166527147839)) ;
#106730=CARTESIAN_POINT('Ctrl Pts',(64.940261777681,246.847591853017,18.2159630621497)) ;
#106731=CARTESIAN_POINT('Ctrl Pts',(64.9400834366341,246.857838938126,18.197502396958)) ;
#106732=CARTESIAN_POINT('Ctrl Pts',(64.9376982652983,246.86777865457,18.1796853539161)) ;
#106733=CARTESIAN_POINT('Ctrl Pts',(64.9285249168178,246.88669215874,18.1459412981879)) ;
#106734=CARTESIAN_POINT('Ctrl Pts',(64.9218878905883,246.895772989479,18.1298165429631)) ;
#106735=CARTESIAN_POINT('Ctrl Pts',(64.9030518920067,246.913652858034,18.0981907599697)) ;
#106736=CARTESIAN_POINT('Ctrl Pts',(64.890241559628,246.92239313214,18.0828088675435)) ;
#106737=CARTESIAN_POINT('Ctrl Pts',(64.8622234505159,246.935114921148,18.0604852570307)) ;
#106738=CARTESIAN_POINT('Ctrl Pts',(64.8483068832618,246.939674844702,18.0525090168905)) ;
#106739=CARTESIAN_POINT('Ctrl Pts',(64.8193104176513,246.945446722844,18.0424220201645)) ;
#106740=CARTESIAN_POINT('Ctrl Pts',(64.8049443310403,246.946891701628,18.0399014096908)) ;
#106741=CARTESIAN_POINT('Ctrl Pts',(64.7902651077865,246.946891701628,18.0399014096908)) ;
#106742=CARTESIAN_POINT('Origin',(64.7902651077865,247.526358208506,20.3087261348769)) ;
#106743=CARTESIAN_POINT('',(64.7902651077865,246.822731508173,17.6577756263215)) ;
#106744=CARTESIAN_POINT('',(64.7902651077865,247.66901668595,20.2623735857207)) ;
#106745=CARTESIAN_POINT('',(64.9402651077865,246.678925224467,17.7005955910409)) ;
#106746=CARTESIAN_POINT('',(64.9402651077865,247.526358208506,20.3087261348769)) ;
#106747=CARTESIAN_POINT('Ctrl Pts',(64.9402651077865,246.678925224467,17.7005955910409)) ;
#106748=CARTESIAN_POINT('Ctrl Pts',(64.9402651077865,246.680324229639,17.7001827000975)) ;
#106749=CARTESIAN_POINT('Ctrl Pts',(64.940243846551,246.681723125547,17.6997697122226)) ;
#106750=CARTESIAN_POINT('Ctrl Pts',(64.9402013305492,246.683121466859,17.6993567614171)) ;
#106751=CARTESIAN_POINT('Ctrl Pts',(64.9396551395109,246.701085561798,17.6940516993336)) ;
#106752=CARTESIAN_POINT('Ctrl Pts',(64.93560627032,246.718788094141,17.6888026219308)) ;
#106753=CARTESIAN_POINT('Ctrl Pts',(64.928263675975,246.73531354078,17.6838889399233)) ;
#106754=CARTESIAN_POINT('Ctrl Pts',(64.9206090302591,246.752541298897,17.6787664323789)) ;
#106755=CARTESIAN_POINT('Ctrl Pts',(64.9095180038064,246.768167444445,17.6741046463009)) ;
#106756=CARTESIAN_POINT('Ctrl Pts',(64.8956136387306,246.781315020339,17.6701759051816)) ;
#106757=CARTESIAN_POINT('Ctrl Pts',(64.8817129938792,246.794459078493,17.6662482152284)) ;
#106758=CARTESIAN_POINT('Ctrl Pts',(64.8652664191735,246.804874499694,17.6631285710069)) ;
#106759=CARTESIAN_POINT('Ctrl Pts',(64.8471986491032,246.811976821569,17.6610001367494)) ;
#106760=CARTESIAN_POINT('Ctrl Pts',(64.8291331055123,246.81907826823,17.6588719647776)) ;
#106761=CARTESIAN_POINT('Ctrl Pts',(64.8097925816884,246.822731508174,17.6577756263219)) ;
#106762=CARTESIAN_POINT('Ctrl Pts',(64.7902651077865,246.822731508174,17.6577756263219)) ;
#106763=CARTESIAN_POINT('Origin',(64.7902651077865,246.340671638724,17.7905095039363)) ;
#106764=CARTESIAN_POINT('',(64.7902651077865,245.872657996292,17.9664732232009)) ;
#106765=CARTESIAN_POINT('Origin',(64.7902651077865,246.340671638724,17.7905095039363)) ;
#106766=CARTESIAN_POINT('',(64.9402651077865,246.014168667474,17.9165880896082)) ;
#106767=CARTESIAN_POINT('Origin',(64.9402651077865,246.340671638724,17.7905095039363)) ;
#106768=CARTESIAN_POINT('Ctrl Pts',(64.9402651077865,246.014168667472,17.9165880896088)) ;
#106769=CARTESIAN_POINT('Ctrl Pts',(64.9402651077865,246.012794157306,17.9170763684267)) ;
#106770=CARTESIAN_POINT('Ctrl Pts',(64.9402438465509,246.011419678561,17.917564504601)) ;
#106771=CARTESIAN_POINT('Ctrl Pts',(64.9402013305491,246.010045670283,17.9180523447824)) ;
#106772=CARTESIAN_POINT('Ctrl Pts',(64.9396551395109,245.992394174936,17.9243194894788)) ;
#106773=CARTESIAN_POINT('Ctrl Pts',(64.9356062703199,245.97498719514,17.9304781840937)) ;
#106774=CARTESIAN_POINT('Ctrl Pts',(64.928263675975,245.958729638151,17.9362163456665)) ;
#106775=CARTESIAN_POINT('Ctrl Pts',(64.9206090302592,245.94178115467,17.9421983721597)) ;
#106776=CARTESIAN_POINT('Ctrl Pts',(64.9095180038062,245.926399208258,17.9476117259015)) ;
#106777=CARTESIAN_POINT('Ctrl Pts',(64.8956136387304,245.913453339835,17.9521612587831)) ;
#106778=CARTESIAN_POINT('Ctrl Pts',(64.8817129938793,245.900510935184,17.9567095744006)) ;
#106779=CARTESIAN_POINT('Ctrl Pts',(64.8652664191737,245.890251001563,17.960307760187)) ;
#106780=CARTESIAN_POINT('Ctrl Pts',(64.8471986491033,245.883254040199,17.9627604607568)) ;
#106781=CARTESIAN_POINT('Ctrl Pts',(64.8291331055124,245.876257941067,17.9652128590819)) ;
#106782=CARTESIAN_POINT('Ctrl Pts',(64.8097925816883,245.872657996292,17.9664732232011)) ;
#106783=CARTESIAN_POINT('Ctrl Pts',(64.7902651077865,245.872657996292,17.9664732232011)) ;
#106784=CARTESIAN_POINT('Origin',(64.7902651077865,246.970272317295,20.8591725524954)) ;
#106785=CARTESIAN_POINT('',(64.7902651077865,245.996818189747,18.3485990065702)) ;
#106786=CARTESIAN_POINT('',(64.7902651077865,246.827613839851,20.9055251016516)) ;
#106787=CARTESIAN_POINT('',(64.9402651077865,246.182069881617,18.4333348922484)) ;
#106788=CARTESIAN_POINT('',(64.9402651077865,246.970272317295,20.8591725524954)) ;
#106789=CARTESIAN_POINT('Ctrl Pts',(64.9402651077865,246.182069881617,18.4333348922484)) ;
#106790=CARTESIAN_POINT('Ctrl Pts',(64.9402651077865,246.181354905731,18.4330018626361)) ;
#106791=CARTESIAN_POINT('Ctrl Pts',(64.940261777681,246.180639897622,18.4326688888987)) ;
#106792=CARTESIAN_POINT('Ctrl Pts',(64.9400834366341,246.16149892488,18.4237569825369)) ;
#106793=CARTESIAN_POINT('Ctrl Pts',(64.9376982652983,246.142984930217,18.4151851106646)) ;
#106794=CARTESIAN_POINT('Ctrl Pts',(64.9285249168178,246.107849325611,18.3990026749412)) ;
#106795=CARTESIAN_POINT('Ctrl Pts',(64.9218878905884,246.091024885902,18.3912950523217)) ;
#106796=CARTESIAN_POINT('Ctrl Pts',(64.9030518920067,246.057970599548,18.3762187794687)) ;
#106797=CARTESIAN_POINT('Ctrl Pts',(64.890241559628,246.041858319741,18.3689119713107)) ;
#106798=CARTESIAN_POINT('Ctrl Pts',(64.862223450516,246.018444687197,18.3583294709921)) ;
#106799=CARTESIAN_POINT('Ctrl Pts',(64.8483068832619,246.010067315225,18.3545568129842)) ;
#106800=CARTESIAN_POINT('Ctrl Pts',(64.8193104176514,245.999468779803,18.3497888860605)) ;
#106801=CARTESIAN_POINT('Ctrl Pts',(64.8049443310404,245.996818189747,18.3485990065702)) ;
#106802=CARTESIAN_POINT('Ctrl Pts',(64.7902651077866,245.996818189747,18.3485990065702)) ;
#106803=CARTESIAN_POINT('Origin',(64.7902651077865,248.040265107786,23.0213203435596)) ;
#106804=CARTESIAN_POINT('',(64.7902651077865,245.461062098449,18.6215803698081)) ;
#106805=CARTESIAN_POINT('Origin',(64.7902651077865,248.040265107786,23.0213203435596)) ;
#106806=CARTESIAN_POINT('',(64.9402651077865,245.420726657553,18.8212586407095)) ;
#106807=CARTESIAN_POINT('Origin',(64.9402651077865,248.040265107786,23.0213203435596)) ;
#106808=CARTESIAN_POINT('Ctrl Pts',(64.9402651077865,245.420726657553,18.8212586407095)) ;
#106809=CARTESIAN_POINT('Ctrl Pts',(64.9402651077865,245.420877483218,18.8204844631751)) ;
#106810=CARTESIAN_POINT('Ctrl Pts',(64.940261777681,245.421028373027,18.8197102924139)) ;
#106811=CARTESIAN_POINT('Ctrl Pts',(64.9400834366348,245.42506927082,18.7989866330484)) ;
#106812=CARTESIAN_POINT('Ctrl Pts',(64.9376982652992,245.429016733826,18.7789700768601)) ;
#106813=CARTESIAN_POINT('Ctrl Pts',(64.9285249168188,245.436577058534,18.7410329785595)) ;
#106814=CARTESIAN_POINT('Ctrl Pts',(64.921887890589,245.440230618388,18.7228912940061)) ;
#106815=CARTESIAN_POINT('Ctrl Pts',(64.9030518920066,245.447462479482,18.6872882037654)) ;
#106816=CARTESIAN_POINT('Ctrl Pts',(64.8902415596279,245.451021707959,18.6699582615064)) ;
#106817=CARTESIAN_POINT('Ctrl Pts',(64.8622234505159,245.45622247327,18.6447959972585)) ;
#106818=CARTESIAN_POINT('Ctrl Pts',(64.8483068832618,245.458094424526,18.6358010482263)) ;
#106819=CARTESIAN_POINT('Ctrl Pts',(64.8193104176514,245.460466753434,18.6244241358249)) ;
#106820=CARTESIAN_POINT('Ctrl Pts',(64.8049443310403,245.461062098449,18.6215803698081)) ;
#106821=CARTESIAN_POINT('Ctrl Pts',(64.7902651077865,245.461062098449,18.6215803698081)) ;
#106822=CARTESIAN_POINT('Origin',(64.7902651077865,246.713272893131,20.6002959107317)) ;
#106823=CARTESIAN_POINT('',(64.7902651077865,245.224895376349,18.2965247632928)) ;
#106824=CARTESIAN_POINT('',(64.7902651077865,246.834625442287,20.5121281228878)) ;
#106825=CARTESIAN_POINT('',(64.9402651077865,245.101359569943,18.3816875553298)) ;
#106826=CARTESIAN_POINT('',(64.9402651077865,246.713272893131,20.6002959107317)) ;
#106827=CARTESIAN_POINT('Ctrl Pts',(64.9402651077865,245.101359569943,18.3816875553298)) ;
#106828=CARTESIAN_POINT('Ctrl Pts',(64.9402651077865,245.10256251261,18.3808625563341)) ;
#106829=CARTESIAN_POINT('Ctrl Pts',(64.940243846551,245.103765321407,18.3800374989151)) ;
#106830=CARTESIAN_POINT('Ctrl Pts',(64.9402013305492,245.104967614207,18.3792126481315)) ;
#106831=CARTESIAN_POINT('Ctrl Pts',(64.939655139511,245.120413129419,18.3686160236467)) ;
#106832=CARTESIAN_POINT('Ctrl Pts',(64.93560627032,245.135627184036,18.3581534710379)) ;
#106833=CARTESIAN_POINT('Ctrl Pts',(64.9282636759752,245.149825406502,18.3483736378944)) ;
#106834=CARTESIAN_POINT('Ctrl Pts',(64.9206090302594,245.164627036234,18.3381781736815)) ;
#106835=CARTESIAN_POINT('Ctrl Pts',(64.9095180038065,245.17804781266,18.3289158071225)) ;
#106836=CARTESIAN_POINT('Ctrl Pts',(64.8956136387306,245.189337852615,18.3211165278942)) ;
#106837=CARTESIAN_POINT('Ctrl Pts',(64.8817129938792,245.200624871829,18.3133193354257)) ;
#106838=CARTESIAN_POINT('Ctrl Pts',(64.8652664191738,245.209566502951,18.3071338353058)) ;
#106839=CARTESIAN_POINT('Ctrl Pts',(64.8471986491033,245.215663490095,18.3029148358767)) ;
#106840=CARTESIAN_POINT('Ctrl Pts',(64.8291331055125,245.22175972591,18.2986963563522)) ;
#106841=CARTESIAN_POINT('Ctrl Pts',(64.8097925816884,245.22489537635,18.2965247632923)) ;
#106842=CARTESIAN_POINT('Ctrl Pts',(64.7902651077865,245.224895376349,18.2965247632922)) ;
#106843=CARTESIAN_POINT('Origin',(64.7902651077865,244.807446220178,18.5717268744974)) ;
#106844=CARTESIAN_POINT('',(64.7902651077865,244.416714575474,18.8837024854464)) ;
#106845=CARTESIAN_POINT('Origin',(64.7902651077865,244.807446220178,18.5717268744974)) ;
#106846=CARTESIAN_POINT('',(64.9402651077865,244.53588386738,18.7925297017961)) ;
#106847=CARTESIAN_POINT('Origin',(64.9402651077865,244.807446220178,18.5717268744974)) ;
#106848=CARTESIAN_POINT('Ctrl Pts',(64.9402651077865,244.535883867376,18.7925297017989)) ;
#106849=CARTESIAN_POINT('Ctrl Pts',(64.9402651077864,244.534727516979,18.7934188295502)) ;
#106850=CARTESIAN_POINT('Ctrl Pts',(64.9402438465509,244.533571152387,18.7943078119297)) ;
#106851=CARTESIAN_POINT('Ctrl Pts',(64.9402013305491,244.532415143768,18.795196367421)) ;
#106852=CARTESIAN_POINT('Ctrl Pts',(64.9396551395109,244.517564228314,18.8066113882631)) ;
#106853=CARTESIAN_POINT('Ctrl Pts',(64.9356062703197,244.502912348047,18.8178477074834)) ;
#106854=CARTESIAN_POINT('Ctrl Pts',(64.9282636759748,244.489223681976,18.8283288848357)) ;
#106855=CARTESIAN_POINT('Ctrl Pts',(64.920609030259,244.474953264168,18.8392554995373)) ;
#106856=CARTESIAN_POINT('Ctrl Pts',(64.9095180038061,244.461996982103,18.8491571877365)) ;
#106857=CARTESIAN_POINT('Ctrl Pts',(64.8956136387302,244.451090612557,18.8574845439792)) ;
#106858=CARTESIAN_POINT('Ctrl Pts',(64.8817129938788,244.440187161098,18.8658096721709)) ;
#106859=CARTESIAN_POINT('Ctrl Pts',(64.8652664191737,244.431541284929,18.8724022440602)) ;
#106860=CARTESIAN_POINT('Ctrl Pts',(64.8471986491032,244.425644705388,18.8768970808898)) ;
#106861=CARTESIAN_POINT('Ctrl Pts',(64.8291331055122,244.419748852478,18.8813913638236)) ;
#106862=CARTESIAN_POINT('Ctrl Pts',(64.8097925816883,244.416714575474,18.8837024854465)) ;
#106863=CARTESIAN_POINT('Ctrl Pts',(64.7902651077865,244.416714575474,18.8837024854465)) ;
#106864=CARTESIAN_POINT('Origin',(64.7902651077865,246.354501080212,21.2956415537952)) ;
#106865=CARTESIAN_POINT('',(64.7902651077865,244.652881297574,19.2087580919617)) ;
#106866=CARTESIAN_POINT('',(64.7902651077865,246.233148531056,21.3838093416391)) ;
#106867=CARTESIAN_POINT('',(64.9402651077865,244.85525095499,19.2321007871753)) ;
#106868=CARTESIAN_POINT('',(64.9402651077865,246.354501080212,21.2956415537952)) ;
#106869=CARTESIAN_POINT('Ctrl Pts',(64.9402651077865,244.85525095499,19.2321007871753)) ;
#106870=CARTESIAN_POINT('Ctrl Pts',(64.9402651077865,244.854468060706,19.2320049968919)) ;
#106871=CARTESIAN_POINT('Ctrl Pts',(64.940261777681,244.853685153042,19.2319092697064)) ;
#106872=CARTESIAN_POINT('Ctrl Pts',(64.9400834366345,244.83272707567,19.2293484289546)) ;
#106873=CARTESIAN_POINT('Ctrl Pts',(64.9376982652987,244.81247036632,19.226917233338)) ;
#106874=CARTESIAN_POINT('Ctrl Pts',(64.9285249168183,244.774053772956,19.2223843213245)) ;
#106875=CARTESIAN_POINT('Ctrl Pts',(64.9218878905887,244.755670993561,19.220252974398)) ;
#106876=CARTESIAN_POINT('Ctrl Pts',(64.9030518920067,244.719575674609,19.2161289230799)) ;
#106877=CARTESIAN_POINT('Ctrl Pts',(64.890241559628,244.70199405801,19.2141587038466)) ;
#106878=CARTESIAN_POINT('Ctrl Pts',(64.862223450516,244.676456197767,19.211329358316)) ;
#106879=CARTESIAN_POINT('Ctrl Pts',(64.8483068832619,244.667323028126,19.2103300976413)) ;
#106880=CARTESIAN_POINT('Ctrl Pts',(64.8193104176513,244.655769851502,19.2090706572321)) ;
#106881=CARTESIAN_POINT('Ctrl Pts',(64.8049443310403,244.652881297574,19.2087580919617)) ;
#106882=CARTESIAN_POINT('Ctrl Pts',(64.7902651077866,244.652881297574,19.2087580919617)) ;
#106883=CARTESIAN_POINT('Origin',(64.7902651077865,248.040265107786,23.0213203435596)) ;
#106884=CARTESIAN_POINT('',(64.7902651077865,244.227702856188,19.633936533347)) ;
#106885=CARTESIAN_POINT('Origin',(64.7902651077865,248.040265107786,23.0213203435596)) ;
#106886=CARTESIAN_POINT('',(64.9402651077865,244.251045551402,19.836306190763)) ;
#106887=CARTESIAN_POINT('Origin',(64.9402651077865,248.040265107786,23.0213203435596)) ;
#106888=CARTESIAN_POINT('Ctrl Pts',(64.9402651077865,244.251045551402,19.836306190763)) ;
#106889=CARTESIAN_POINT('Ctrl Pts',(64.9402651077865,244.250949761118,19.835523296477)) ;
#106890=CARTESIAN_POINT('Ctrl Pts',(64.9402617776811,244.250854033933,19.8347403888173)) ;
#106891=CARTESIAN_POINT('Ctrl Pts',(64.9400834366345,244.248293193182,19.8137823114414)) ;
#106892=CARTESIAN_POINT('Ctrl Pts',(64.9376982652987,244.245861997565,19.7935256020932)) ;
#106893=CARTESIAN_POINT('Ctrl Pts',(64.9285249168183,244.241329085551,19.7551090087289)) ;
#106894=CARTESIAN_POINT('Ctrl Pts',(64.9218878905886,244.239197738625,19.7367262293338)) ;
#106895=CARTESIAN_POINT('Ctrl Pts',(64.9030518920067,244.235073687307,19.7006309103819)) ;
#106896=CARTESIAN_POINT('Ctrl Pts',(64.890241559628,244.233103468073,19.683049293783)) ;
#106897=CARTESIAN_POINT('Ctrl Pts',(64.8622234505159,244.230274122543,19.6575114335404)) ;
#106898=CARTESIAN_POINT('Ctrl Pts',(64.8483068832618,244.229274861868,19.648378263899)) ;
#106899=CARTESIAN_POINT('Ctrl Pts',(64.8193104176514,244.228015421459,19.6368250872756)) ;
#106900=CARTESIAN_POINT('Ctrl Pts',(64.8049443310404,244.227702856188,19.6339365333471)) ;
#106901=CARTESIAN_POINT('Ctrl Pts',(64.7902651077866,244.227702856188,19.6339365333471)) ;
#106902=CARTESIAN_POINT('Origin',(64.7902651077865,246.030082821424,21.1288524263407)) ;
#106903=CARTESIAN_POINT('',(64.7902651077865,243.902647249673,19.3977698112471)) ;
#106904=CARTESIAN_POINT('',(64.7902651077865,246.118250609268,21.0074998771845)) ;
#106905=CARTESIAN_POINT('',(64.9402651077865,243.811474466023,19.5169391031534)) ;
#106906=CARTESIAN_POINT('',(64.9402651077865,246.030082821424,21.1288524263407)) ;
#106907=CARTESIAN_POINT('Ctrl Pts',(64.9402651077865,243.811474466023,19.5169391031534)) ;
#106908=CARTESIAN_POINT('Ctrl Pts',(64.9402651077865,243.812363593775,19.5157827527548)) ;
#106909=CARTESIAN_POINT('Ctrl Pts',(64.940243846551,243.813252576157,19.5146263881627)) ;
#106910=CARTESIAN_POINT('Ctrl Pts',(64.9402013305491,243.814141131649,19.5134703795416)) ;
#106911=CARTESIAN_POINT('Ctrl Pts',(64.9396551395108,243.825556152481,19.4986194640777)) ;
#106912=CARTESIAN_POINT('Ctrl Pts',(64.9356062703196,243.836792471712,19.4839675838214)) ;
#106913=CARTESIAN_POINT('Ctrl Pts',(64.928263675975,243.847273649063,19.4702789177503)) ;
#106914=CARTESIAN_POINT('Ctrl Pts',(64.9206090302592,243.858200263764,19.456008499942)) ;
#106915=CARTESIAN_POINT('Ctrl Pts',(64.9095180038061,243.868101951963,19.4430522178762)) ;
#106916=CARTESIAN_POINT('Ctrl Pts',(64.8956136387302,243.876429308206,19.4321458483306)) ;
#106917=CARTESIAN_POINT('Ctrl Pts',(64.8817129938788,243.884754436398,19.4212423968717)) ;
#106918=CARTESIAN_POINT('Ctrl Pts',(64.8652664191734,243.891347008287,19.412596520702)) ;
#106919=CARTESIAN_POINT('Ctrl Pts',(64.847198649103,243.895841845117,19.4066999411611)) ;
#106920=CARTESIAN_POINT('Ctrl Pts',(64.8291331055123,243.900336128051,19.4008040882519)) ;
#106921=CARTESIAN_POINT('Ctrl Pts',(64.8097925816883,243.902647249673,19.3977698112471)) ;
#106922=CARTESIAN_POINT('Ctrl Pts',(64.7902651077865,243.902647249673,19.3977698112472)) ;
#106923=CARTESIAN_POINT('Origin',(64.7902651077865,243.590671638724,19.788501455951)) ;
#106924=CARTESIAN_POINT('',(64.7902651077865,243.315469527519,20.2059506121228)) ;
#106925=CARTESIAN_POINT('Origin',(64.7902651077865,243.590671638724,19.788501455951)) ;
#106926=CARTESIAN_POINT('',(64.9402651077865,243.400632319557,20.0824148057165)) ;
#106927=CARTESIAN_POINT('Origin',(64.9402651077865,243.590671638724,19.788501455951)) ;
#106928=CARTESIAN_POINT('Ctrl Pts',(64.9402651077865,243.400632319555,20.0824148057187)) ;
#106929=CARTESIAN_POINT('Ctrl Pts',(64.9402651077865,243.39980732056,20.0836177483853)) ;
#106930=CARTESIAN_POINT('Ctrl Pts',(64.9402438465509,243.398982263143,20.084820557182)) ;
#106931=CARTESIAN_POINT('Ctrl Pts',(64.9402013305491,243.398157412359,20.0860228499814)) ;
#106932=CARTESIAN_POINT('Ctrl Pts',(64.9396551395109,243.387560787866,20.1014683651894)) ;
#106933=CARTESIAN_POINT('Ctrl Pts',(64.9356062703196,243.377098235265,20.1166824198106)) ;
#106934=CARTESIAN_POINT('Ctrl Pts',(64.9282636759749,243.367318402122,20.1308806422758)) ;
#106935=CARTESIAN_POINT('Ctrl Pts',(64.9206090302592,243.357122937909,20.1456822720079)) ;
#106936=CARTESIAN_POINT('Ctrl Pts',(64.9095180038063,243.34786057135,20.1591030484339)) ;
#106937=CARTESIAN_POINT('Ctrl Pts',(64.8956136387305,243.340061292122,20.1703930883887)) ;
#106938=CARTESIAN_POINT('Ctrl Pts',(64.8817129938791,243.332264099653,20.1816801076026)) ;
#106939=CARTESIAN_POINT('Ctrl Pts',(64.8652664191737,243.326078599533,20.1906217387245)) ;
#106940=CARTESIAN_POINT('Ctrl Pts',(64.8471986491031,243.321859600104,20.1967187258679)) ;
#106941=CARTESIAN_POINT('Ctrl Pts',(64.8291331055123,243.317641120579,20.2028149616835)) ;
#106942=CARTESIAN_POINT('Ctrl Pts',(64.8097925816883,243.315469527519,20.2059506121225)) ;
#106943=CARTESIAN_POINT('Ctrl Pts',(64.7902651077865,243.315469527519,20.2059506121226)) ;
#106944=CARTESIAN_POINT('Origin',(64.7902651077865,245.903744171556,21.9010320185483)) ;
#106945=CARTESIAN_POINT('',(64.7902651077865,243.640525134035,20.4421173342227)) ;
#106946=CARTESIAN_POINT('',(64.7902651077865,245.815576383712,22.0223845677046)) ;
#106947=CARTESIAN_POINT('',(64.9402651077865,243.840203404936,20.4017818933262)) ;
#106948=CARTESIAN_POINT('',(64.9402651077865,245.903744171556,21.9010320185483)) ;
#106949=CARTESIAN_POINT('Ctrl Pts',(64.9402651077865,243.840203404936,20.4017818933262)) ;
#106950=CARTESIAN_POINT('Ctrl Pts',(64.9402651077865,243.839429227398,20.4019327189919)) ;
#106951=CARTESIAN_POINT('Ctrl Pts',(64.9402617776811,243.83865505664,20.4020836088006)) ;
#106952=CARTESIAN_POINT('Ctrl Pts',(64.9400834366345,243.817931397271,20.4061245065949)) ;
#106953=CARTESIAN_POINT('Ctrl Pts',(64.9376982652987,243.797914841084,20.4100719696)) ;
#106954=CARTESIAN_POINT('Ctrl Pts',(64.9285249168183,243.759977742784,20.4176322943074)) ;
#106955=CARTESIAN_POINT('Ctrl Pts',(64.9218878905886,243.741836058232,20.4212858541613)) ;
#106956=CARTESIAN_POINT('Ctrl Pts',(64.9030518920066,243.706232967992,20.4285177152552)) ;
#106957=CARTESIAN_POINT('Ctrl Pts',(64.8902415596279,243.688903025733,20.4320769437325)) ;
#106958=CARTESIAN_POINT('Ctrl Pts',(64.862223450516,243.663740761485,20.4372777090437)) ;
#106959=CARTESIAN_POINT('Ctrl Pts',(64.8483068832619,243.654745812453,20.4391496602992)) ;
#106960=CARTESIAN_POINT('Ctrl Pts',(64.8193104176513,243.643368900052,20.4415219892068)) ;
#106961=CARTESIAN_POINT('Ctrl Pts',(64.8049443310403,243.640525134035,20.4421173342227)) ;
#106962=CARTESIAN_POINT('Ctrl Pts',(64.7902651077865,243.640525134035,20.4421173342227)) ;
#106963=CARTESIAN_POINT('Origin',(64.7902651077865,248.040265107786,23.0213203435596)) ;
#106964=CARTESIAN_POINT('',(64.7902651077865,243.367543770797,20.9778734255204)) ;
#106965=CARTESIAN_POINT('Origin',(64.7902651077865,248.040265107786,23.0213203435596)) ;
#106966=CARTESIAN_POINT('',(64.9402651077865,243.452279656475,21.1631251173908)) ;
#106967=CARTESIAN_POINT('Origin',(64.9402651077865,248.040265107786,23.0213203435596)) ;
#106968=CARTESIAN_POINT('Ctrl Pts',(64.9402651077865,243.452279656475,21.1631251173908)) ;
#106969=CARTESIAN_POINT('Ctrl Pts',(64.9402651077865,243.451946626863,21.162410141506)) ;
#106970=CARTESIAN_POINT('Ctrl Pts',(64.940261777681,243.451613653127,21.1616951333977)) ;
#106971=CARTESIAN_POINT('Ctrl Pts',(64.9400834366345,243.442701746765,21.1425541606558)) ;
#106972=CARTESIAN_POINT('Ctrl Pts',(64.9376982652987,243.434129874892,21.1240401659928)) ;
#106973=CARTESIAN_POINT('Ctrl Pts',(64.9285249168183,243.417947439168,21.0889045613856)) ;
#106974=CARTESIAN_POINT('Ctrl Pts',(64.9218878905886,243.410239816549,21.0720801216755)) ;
#106975=CARTESIAN_POINT('Ctrl Pts',(64.9030518920067,243.395163543695,21.0390258353216)) ;
#106976=CARTESIAN_POINT('Ctrl Pts',(64.890241559628,243.387856735537,21.0229135555139)) ;
#106977=CARTESIAN_POINT('Ctrl Pts',(64.8622234505159,243.377274235219,20.9994999229698)) ;
#106978=CARTESIAN_POINT('Ctrl Pts',(64.8483068832618,243.373501577211,20.9911225509982)) ;
#106979=CARTESIAN_POINT('Ctrl Pts',(64.8193104176513,243.368733650287,20.9805240155764)) ;
#106980=CARTESIAN_POINT('Ctrl Pts',(64.8049443310403,243.367543770797,20.9778734255204)) ;
#106981=CARTESIAN_POINT('Ctrl Pts',(64.7902651077865,243.367543770797,20.9778734255204)) ;
#106982=CARTESIAN_POINT('Origin',(64.7902651077865,245.543663397671,21.8426568872864)) ;
#106983=CARTESIAN_POINT('',(64.7902651077865,242.985417987428,20.8537132320653)) ;
#106984=CARTESIAN_POINT('',(64.7902651077865,245.590015946827,21.6999984098422)) ;
#106985=CARTESIAN_POINT('',(64.9402651077865,242.935532853835,20.9952239032475)) ;
#106986=CARTESIAN_POINT('',(64.9402651077865,245.543663397671,21.8426568872864)) ;
#106987=CARTESIAN_POINT('Ctrl Pts',(64.9402651077865,242.935532853835,20.9952239032475)) ;
#106988=CARTESIAN_POINT('Ctrl Pts',(64.9402651077865,242.936021132653,20.9938493930805)) ;
#106989=CARTESIAN_POINT('Ctrl Pts',(64.940243846551,242.936509268827,20.9924749143349)) ;
#106990=CARTESIAN_POINT('Ctrl Pts',(64.9402013305491,242.936997109009,20.9911009060562)) ;
#106991=CARTESIAN_POINT('Ctrl Pts',(64.9396551395109,242.943264253705,20.9734494107095)) ;
#106992=CARTESIAN_POINT('Ctrl Pts',(64.9356062703199,242.94942294832,20.9560424309132)) ;
#106993=CARTESIAN_POINT('Ctrl Pts',(64.928263675975,242.955161109893,20.9397848739239)) ;
#106994=CARTESIAN_POINT('Ctrl Pts',(64.9206090302593,242.961143136386,20.9228363904435)) ;
#106995=CARTESIAN_POINT('Ctrl Pts',(64.9095180038063,242.966556490128,20.9074544440317)) ;
#106996=CARTESIAN_POINT('Ctrl Pts',(64.8956136387305,242.97110602301,20.8945085756088)) ;
#106997=CARTESIAN_POINT('Ctrl Pts',(64.8817129938792,242.975654338627,20.881566170957)) ;
#106998=CARTESIAN_POINT('Ctrl Pts',(64.8652664191736,242.979252524414,20.8713062373364)) ;
#106999=CARTESIAN_POINT('Ctrl Pts',(64.8471986491032,242.981705224983,20.8643092759726)) ;
#107000=CARTESIAN_POINT('Ctrl Pts',(64.8291331055124,242.984157623308,20.8573131768398)) ;
#107001=CARTESIAN_POINT('Ctrl Pts',(64.8097925816883,242.985417987427,20.853713232065)) ;
#107002=CARTESIAN_POINT('Ctrl Pts',(64.7902651077865,242.985417987427,20.853713232065)) ;
#107003=CARTESIAN_POINT('Origin',(64.7902651077865,242.809454268163,21.3217268744974)) ;
#107004=CARTESIAN_POINT('',(64.7902651077865,242.676720390548,21.8037867439466)) ;
#107005=CARTESIAN_POINT('Origin',(64.7902651077865,242.809454268163,21.3217268744974)) ;
#107006=CARTESIAN_POINT('',(64.9402651077865,242.719540355268,21.6599804602403)) ;
#107007=CARTESIAN_POINT('Origin',(64.9402651077865,242.809454268163,21.3217268744974)) ;
#107008=CARTESIAN_POINT('Ctrl Pts',(64.9402651077865,242.719540355266,21.6599804602464)) ;
#107009=CARTESIAN_POINT('Ctrl Pts',(64.9402651077864,242.719127464323,21.6613794654168)) ;
#107010=CARTESIAN_POINT('Ctrl Pts',(64.9402438465509,242.718714476449,21.6627783613227)) ;
#107011=CARTESIAN_POINT('Ctrl Pts',(64.9402013305491,242.718301525644,21.6641767026329)) ;
#107012=CARTESIAN_POINT('Ctrl Pts',(64.9396551395109,242.71299646356,21.6821407975713)) ;
#107013=CARTESIAN_POINT('Ctrl Pts',(64.9356062703198,242.707747386158,21.6998433299147)) ;
#107014=CARTESIAN_POINT('Ctrl Pts',(64.928263675975,242.70283370415,21.7163687765538)) ;
#107015=CARTESIAN_POINT('Ctrl Pts',(64.9206090302592,242.697711196606,21.7335965346699)) ;
#107016=CARTESIAN_POINT('Ctrl Pts',(64.9095180038063,242.693049410528,21.7492226802188)) ;
#107017=CARTESIAN_POINT('Ctrl Pts',(64.8956136387304,242.689120669408,21.7623702561123)) ;
#107018=CARTESIAN_POINT('Ctrl Pts',(64.8817129938791,242.685192979455,21.7755143142664)) ;
#107019=CARTESIAN_POINT('Ctrl Pts',(64.8652664191737,242.682073335234,21.7859297354671)) ;
#107020=CARTESIAN_POINT('Ctrl Pts',(64.8471986491032,242.679944900976,21.7930320573425)) ;
#107021=CARTESIAN_POINT('Ctrl Pts',(64.8291331055123,242.677816729004,21.8001335040033)) ;
#107022=CARTESIAN_POINT('Ctrl Pts',(64.8097925816883,242.676720390548,21.8037867439466)) ;
#107023=CARTESIAN_POINT('Ctrl Pts',(64.7902651077865,242.676720390548,21.8037867439466)) ;
#107024=CARTESIAN_POINT('Origin',(64.7902651077865,245.662124818155,22.6160841100613)) ;
#107025=CARTESIAN_POINT('',(64.7902651077865,243.058846173918,21.9279469374017)) ;
#107026=CARTESIAN_POINT('',(64.7902651077865,245.615772268999,22.7587425875056)) ;
#107027=CARTESIAN_POINT('',(64.9402651077865,243.236287157908,21.8278816743835)) ;
#107028=CARTESIAN_POINT('',(64.9402651077865,245.662124818155,22.6160841100613)) ;
#107029=CARTESIAN_POINT('Ctrl Pts',(64.9402651077865,243.236287157908,21.8278816743835)) ;
#107030=CARTESIAN_POINT('Ctrl Pts',(64.9402651077865,243.235597479012,21.8282643521305)) ;
#107031=CARTESIAN_POINT('Ctrl Pts',(64.940261777681,243.234907826379,21.8286470887893)) ;
#107032=CARTESIAN_POINT('Ctrl Pts',(64.9400834366345,243.216447161187,21.8388941738976)) ;
#107033=CARTESIAN_POINT('Ctrl Pts',(64.9376982652987,243.198630118145,21.8488338903421)) ;
#107034=CARTESIAN_POINT('Ctrl Pts',(64.9285249168183,243.164886062416,21.8677473945122)) ;
#107035=CARTESIAN_POINT('Ctrl Pts',(64.9218878905887,243.14876130719,21.8768282252524)) ;
#107036=CARTESIAN_POINT('Ctrl Pts',(64.9030518920067,243.117135524196,21.8947080938071)) ;
#107037=CARTESIAN_POINT('Ctrl Pts',(64.890241559628,243.10175363177,21.903448367913)) ;
#107038=CARTESIAN_POINT('Ctrl Pts',(64.8622234505159,243.079430021257,21.9161701569215)) ;
#107039=CARTESIAN_POINT('Ctrl Pts',(64.8483068832618,243.071453781117,21.9207300804757)) ;
#107040=CARTESIAN_POINT('Ctrl Pts',(64.8193104176513,243.061366784391,21.9265019586177)) ;
#107041=CARTESIAN_POINT('Ctrl Pts',(64.8049443310403,243.058846173917,21.9279469374017)) ;
#107042=CARTESIAN_POINT('Ctrl Pts',(64.7902651077865,243.058846173917,21.9279469374017)) ;
#107043=CARTESIAN_POINT('Origin',(64.7902651077865,248.040265107786,23.0213203435596)) ;
#107044=CARTESIAN_POINT('',(64.7902651077865,242.964783206634,22.5218371395634)) ;
#107045=CARTESIAN_POINT('Origin',(64.7902651077865,248.040265107786,23.0213203435596)) ;
#107046=CARTESIAN_POINT('',(64.9402651077865,243.102617743897,22.6718371395634)) ;
#107047=CARTESIAN_POINT('Origin',(64.9402651077865,248.040265107786,23.0213203435596)) ;
#107048=CARTESIAN_POINT('Ctrl Pts',(64.9402651077865,243.102617743897,22.6718371395634)) ;
#107049=CARTESIAN_POINT('Ctrl Pts',(64.9402651077865,243.102080074215,22.6712600688988)) ;
#107050=CARTESIAN_POINT('Ctrl Pts',(64.940261777681,243.101542447717,22.6706829503216)) ;
#107051=CARTESIAN_POINT('Ctrl Pts',(64.9400834366345,243.087151835233,22.655232733985)) ;
#107052=CARTESIAN_POINT('Ctrl Pts',(64.9376982652987,243.073278361647,22.6402737328005)) ;
#107053=CARTESIAN_POINT('Ctrl Pts',(64.9285249168183,243.047030451771,22.6118584347341)) ;
#107054=CARTESIAN_POINT('Ctrl Pts',(64.9218878905887,243.034501029262,22.5982392280904)) ;
#107055=CARTESIAN_POINT('Ctrl Pts',(64.9030518920067,243.009948305503,22.5714615581854)) ;
#107056=CARTESIAN_POINT('Ctrl Pts',(64.890241559628,242.998020149712,22.5583957973774)) ;
#107057=CARTESIAN_POINT('Ctrl Pts',(64.8622234505159,242.98072038347,22.5393982820177)) ;
#107058=CARTESIAN_POINT('Ctrl Pts',(64.8483068832618,242.97454362218,22.5325967432531)) ;
#107059=CARTESIAN_POINT('Ctrl Pts',(64.8193104176514,242.966733926649,22.5239903075244)) ;
#107060=CARTESIAN_POINT('Ctrl Pts',(64.8049443310404,242.964783206634,22.5218371395634)) ;
#107061=CARTESIAN_POINT('Ctrl Pts',(64.7902651077866,242.964783206634,22.5218371395634)) ;
#107062=CARTESIAN_POINT('Origin',(64.7902651077865,245.30162874415,22.6718371395634)) ;
#107063=CARTESIAN_POINT('',(64.7902651077865,242.562992380514,22.5218371395634)) ;
#107064=CARTESIAN_POINT('',(64.7902651077865,245.30162874415,22.5218371395634)) ;
#107065=CARTESIAN_POINT('',(64.9402651077865,242.559278001424,22.6718371395634)) ;
#107066=CARTESIAN_POINT('',(64.9402651077865,245.30162874415,22.6718371395634)) ;
#107067=CARTESIAN_POINT('Ctrl Pts',(64.9402651077865,242.559278001424,22.6718371395634)) ;
#107068=CARTESIAN_POINT('Ctrl Pts',(64.9402651077865,242.559317635176,22.6703790162596)) ;
#107069=CARTESIAN_POINT('Ctrl Pts',(64.940243846551,242.559357142974,22.6689209669185)) ;
#107070=CARTESIAN_POINT('Ctrl Pts',(64.9402013305491,242.559396514649,22.6674634564849)) ;
#107071=CARTESIAN_POINT('Ctrl Pts',(64.9396551395109,242.559902311412,22.6487392325954)) ;
#107072=CARTESIAN_POINT('Ctrl Pts',(64.9356062703199,242.560380525481,22.6302810697323)) ;
#107073=CARTESIAN_POINT('Ctrl Pts',(64.928263675975,242.56081398004,22.6130460247761)) ;
#107074=CARTESIAN_POINT('Ctrl Pts',(64.9206090302592,242.561265855892,22.5950785112737)) ;
#107075=CARTESIAN_POINT('Ctrl Pts',(64.9095180038063,242.561660978396,22.5787765926026)) ;
#107076=CARTESIAN_POINT('Ctrl Pts',(64.8956136387304,242.561987347939,22.5650584571031)) ;
#107077=CARTESIAN_POINT('Ctrl Pts',(64.881712993879,242.56231363016,22.5513439920008)) ;
#107078=CARTESIAN_POINT('Ctrl Pts',(64.8652664191735,242.562565214349,22.5404743147171)) ;
#107079=CARTESIAN_POINT('Ctrl Pts',(64.8471986491031,242.562735691238,22.5330618828598)) ;
#107080=CARTESIAN_POINT('Ctrl Pts',(64.8291331055124,242.562906147119,22.5256503644317)) ;
#107081=CARTESIAN_POINT('Ctrl Pts',(64.8097925816883,242.562992380514,22.5218371395634)) ;
#107082=CARTESIAN_POINT('Ctrl Pts',(64.7902651077865,242.562992380514,22.5218371395634)) ;
#107083=CARTESIAN_POINT('Origin',(64.7902651077865,242.540265107786,23.0213203435596)) ;
#107084=CARTESIAN_POINT('',(64.7902651077865,242.562992380514,23.5208035475559)) ;
#107085=CARTESIAN_POINT('Origin',(64.7902651077865,242.540265107786,23.0213203435596)) ;
#107086=CARTESIAN_POINT('',(64.9402651077865,242.559278001425,23.3708035475559)) ;
#107087=CARTESIAN_POINT('Origin',(64.9402651077865,242.540265107786,23.0213203435596)) ;
#107088=CARTESIAN_POINT('Ctrl Pts',(64.9402651077865,242.559278001425,23.3708035475559)) ;
#107089=CARTESIAN_POINT('Ctrl Pts',(64.9402651077865,242.559317635176,23.3722616708596)) ;
#107090=CARTESIAN_POINT('Ctrl Pts',(64.940243846551,242.559357142975,23.3737197202007)) ;
#107091=CARTESIAN_POINT('Ctrl Pts',(64.9402013305491,242.55939651465,23.3751772306343)) ;
#107092=CARTESIAN_POINT('Ctrl Pts',(64.9396551395109,242.559902311413,23.3939014545241)) ;
#107093=CARTESIAN_POINT('Ctrl Pts',(64.9356062703199,242.560380525481,23.412359617387)) ;
#107094=CARTESIAN_POINT('Ctrl Pts',(64.928263675975,242.56081398004,23.4295946623431)) ;
#107095=CARTESIAN_POINT('Ctrl Pts',(64.9206090302592,242.561265855892,23.4475621758458)) ;
#107096=CARTESIAN_POINT('Ctrl Pts',(64.9095180038062,242.561660978395,23.4638640945167)) ;
#107097=CARTESIAN_POINT('Ctrl Pts',(64.8956136387304,242.561987347939,23.4775822300162)) ;
#107098=CARTESIAN_POINT('Ctrl Pts',(64.8817129938791,242.56231363016,23.4912966951184)) ;
#107099=CARTESIAN_POINT('Ctrl Pts',(64.8652664191737,242.562565214349,23.5021663724021)) ;
#107100=CARTESIAN_POINT('Ctrl Pts',(64.8471986491032,242.562735691238,23.5095788042594)) ;
#107101=CARTESIAN_POINT('Ctrl Pts',(64.8291331055124,242.56290614712,23.5169903226877)) ;
#107102=CARTESIAN_POINT('Ctrl Pts',(64.8097925816884,242.562992380514,23.5208035475559)) ;
#107103=CARTESIAN_POINT('Ctrl Pts',(64.7902651077866,242.562992380514,23.5208035475559)) ;
#107104=CARTESIAN_POINT('Origin',(64.7902651077865,245.653294405781,23.3708035475559)) ;
#107105=CARTESIAN_POINT('',(64.7902651077865,242.964783206634,23.5208035475559)) ;
#107106=CARTESIAN_POINT('',(64.7902651077865,245.653294405781,23.5208035475559)) ;
#107107=CARTESIAN_POINT('',(64.9402651077865,243.102617743897,23.3708035475559)) ;
#107108=CARTESIAN_POINT('',(64.9402651077865,245.653294405781,23.3708035475559)) ;
#107109=CARTESIAN_POINT('Ctrl Pts',(64.9402651077865,243.102617743897,23.3708035475559)) ;
#107110=CARTESIAN_POINT('Ctrl Pts',(64.9402651077865,243.102080074215,23.3713806182205)) ;
#107111=CARTESIAN_POINT('Ctrl Pts',(64.940261777681,243.101542447717,23.3719577367977)) ;
#107112=CARTESIAN_POINT('Ctrl Pts',(64.9400834366345,243.087151835233,23.3874079531342)) ;
#107113=CARTESIAN_POINT('Ctrl Pts',(64.9376982652987,243.073278361647,23.4023669543188)) ;
#107114=CARTESIAN_POINT('Ctrl Pts',(64.9285249168183,243.047030451771,23.4307822523853)) ;
#107115=CARTESIAN_POINT('Ctrl Pts',(64.9218878905887,243.034501029262,23.4444014590289)) ;
#107116=CARTESIAN_POINT('Ctrl Pts',(64.9030518920067,243.009948305503,23.4711791289339)) ;
#107117=CARTESIAN_POINT('Ctrl Pts',(64.890241559628,242.998020149712,23.4842448897419)) ;
#107118=CARTESIAN_POINT('Ctrl Pts',(64.8622234505159,242.98072038347,23.5032424051016)) ;
#107119=CARTESIAN_POINT('Ctrl Pts',(64.8483068832618,242.97454362218,23.5100439438662)) ;
#107120=CARTESIAN_POINT('Ctrl Pts',(64.8193104176513,242.966733926649,23.5186503795949)) ;
#107121=CARTESIAN_POINT('Ctrl Pts',(64.8049443310403,242.964783206634,23.5208035475559)) ;
#107122=CARTESIAN_POINT('Ctrl Pts',(64.7902651077865,242.964783206634,23.5208035475559)) ;
#107123=CARTESIAN_POINT('Origin',(64.7902651077865,248.040265107786,23.0213203435596)) ;
#107124=CARTESIAN_POINT('',(64.7902651077865,243.058846173918,24.1146937497175)) ;
#107125=CARTESIAN_POINT('Origin',(64.7902651077865,248.040265107786,23.0213203435596)) ;
#107126=CARTESIAN_POINT('',(64.9402651077865,243.236287157908,24.2147590127358)) ;
#107127=CARTESIAN_POINT('Origin',(64.9402651077865,248.040265107786,23.0213203435596)) ;
#107128=CARTESIAN_POINT('Ctrl Pts',(64.9402651077865,243.236287157908,24.2147590127358)) ;
#107129=CARTESIAN_POINT('Ctrl Pts',(64.9402651077865,243.235597479013,24.2143763349894)) ;
#107130=CARTESIAN_POINT('Ctrl Pts',(64.940261777681,243.234907826381,24.2139935983313)) ;
#107131=CARTESIAN_POINT('Ctrl Pts',(64.9400834366348,243.216447161191,24.2037465132234)) ;
#107132=CARTESIAN_POINT('Ctrl Pts',(64.9376982652992,243.198630118147,24.1938067967784)) ;
#107133=CARTESIAN_POINT('Ctrl Pts',(64.9285249168188,243.164886062417,24.1748932926076)) ;
#107134=CARTESIAN_POINT('Ctrl Pts',(64.921887890589,243.148761307191,24.1658124618672)) ;
#107135=CARTESIAN_POINT('Ctrl Pts',(64.9030518920067,243.117135524196,24.1479325933122)) ;
#107136=CARTESIAN_POINT('Ctrl Pts',(64.890241559628,243.10175363177,24.1391923192062)) ;
#107137=CARTESIAN_POINT('Ctrl Pts',(64.8622234505159,243.079430021257,24.1264705301977)) ;
#107138=CARTESIAN_POINT('Ctrl Pts',(64.8483068832618,243.071453781117,24.1219106066435)) ;
#107139=CARTESIAN_POINT('Ctrl Pts',(64.8193104176513,243.061366784391,24.1161387285016)) ;
#107140=CARTESIAN_POINT('Ctrl Pts',(64.8049443310403,243.058846173917,24.1146937497176)) ;
#107141=CARTESIAN_POINT('Ctrl Pts',(64.7902651077865,243.058846173917,24.1146937497176)) ;
#107142=CARTESIAN_POINT('Origin',(64.7902651077865,245.327670899104,23.5352272428401)) ;
#107143=CARTESIAN_POINT('',(64.7902651077865,242.676720390548,24.2388539431727)) ;
#107144=CARTESIAN_POINT('',(64.7902651077865,245.281318349947,23.3925687653958)) ;
#107145=CARTESIAN_POINT('',(64.9402651077865,242.719540355268,24.3826602268791)) ;
#107146=CARTESIAN_POINT('',(64.9402651077865,245.327670899104,23.5352272428401)) ;
#107147=CARTESIAN_POINT('Ctrl Pts',(64.9402651077865,242.719540355268,24.3826602268791)) ;
#107148=CARTESIAN_POINT('Ctrl Pts',(64.9402651077865,242.719127464324,24.3812612217067)) ;
#107149=CARTESIAN_POINT('Ctrl Pts',(64.940243846551,242.718714476449,24.3798623257986)) ;
#107150=CARTESIAN_POINT('Ctrl Pts',(64.9402013305491,242.718301525644,24.3784639844864)) ;
#107151=CARTESIAN_POINT('Ctrl Pts',(64.9396551395108,242.71299646356,24.360499889548)) ;
#107152=CARTESIAN_POINT('Ctrl Pts',(64.9356062703197,242.707747386158,24.3427973572043)) ;
#107153=CARTESIAN_POINT('Ctrl Pts',(64.9282636759749,242.702833704151,24.3262719105654)) ;
#107154=CARTESIAN_POINT('Ctrl Pts',(64.9206090302591,242.697711196606,24.3090441524494)) ;
#107155=CARTESIAN_POINT('Ctrl Pts',(64.9095180038062,242.693049410527,24.2934180069009)) ;
#107156=CARTESIAN_POINT('Ctrl Pts',(64.8956136387304,242.689120669408,24.2802704310072)) ;
#107157=CARTESIAN_POINT('Ctrl Pts',(64.8817129938791,242.685192979455,24.2671263728531)) ;
#107158=CARTESIAN_POINT('Ctrl Pts',(64.8652664191735,242.682073335233,24.2567109516525)) ;
#107159=CARTESIAN_POINT('Ctrl Pts',(64.8471986491031,242.679944900976,24.2496086297771)) ;
#107160=CARTESIAN_POINT('Ctrl Pts',(64.8291331055123,242.677816729004,24.2425071831162)) ;
#107161=CARTESIAN_POINT('Ctrl Pts',(64.8097925816884,242.676720390548,24.2388539431728)) ;
#107162=CARTESIAN_POINT('Ctrl Pts',(64.7902651077866,242.676720390548,24.2388539431728)) ;
#107163=CARTESIAN_POINT('Origin',(64.7902651077865,242.809454268163,24.7209138126218)) ;
#107164=CARTESIAN_POINT('',(64.7902651077865,242.985417987428,25.188927455054)) ;
#107165=CARTESIAN_POINT('Origin',(64.7902651077865,242.809454268163,24.7209138126218)) ;
#107166=CARTESIAN_POINT('',(64.9402651077865,242.935532853835,25.0474167838717)) ;
#107167=CARTESIAN_POINT('Origin',(64.9402651077865,242.809454268163,24.7209138126218)) ;
#107168=CARTESIAN_POINT('Ctrl Pts',(64.9402651077865,242.935532853835,25.0474167838725)) ;
#107169=CARTESIAN_POINT('Ctrl Pts',(64.9402651077865,242.936021132653,25.0487912940392)) ;
#107170=CARTESIAN_POINT('Ctrl Pts',(64.940243846551,242.936509268827,25.0501657727845)) ;
#107171=CARTESIAN_POINT('Ctrl Pts',(64.9402013305491,242.936997109009,25.051539781063)) ;
#107172=CARTESIAN_POINT('Ctrl Pts',(64.9396551395109,242.943264253705,25.0691912764101)) ;
#107173=CARTESIAN_POINT('Ctrl Pts',(64.9356062703198,242.949422948318,25.0865982562069)) ;
#107174=CARTESIAN_POINT('Ctrl Pts',(64.9282636759749,242.955161109891,25.102855813196)) ;
#107175=CARTESIAN_POINT('Ctrl Pts',(64.9206090302591,242.961143136385,25.1198042966763)) ;
#107176=CARTESIAN_POINT('Ctrl Pts',(64.9095180038061,242.966556490128,25.1351862430876)) ;
#107177=CARTESIAN_POINT('Ctrl Pts',(64.8956136387304,242.97110602301,25.1481321115104)) ;
#107178=CARTESIAN_POINT('Ctrl Pts',(64.8817129938791,242.975654338627,25.1610745161621)) ;
#107179=CARTESIAN_POINT('Ctrl Pts',(64.8652664191736,242.979252524414,25.1713344497827)) ;
#107180=CARTESIAN_POINT('Ctrl Pts',(64.8471986491031,242.981705224984,25.1783314111464)) ;
#107181=CARTESIAN_POINT('Ctrl Pts',(64.8291331055122,242.984157623309,25.1853275102791)) ;
#107182=CARTESIAN_POINT('Ctrl Pts',(64.8097925816883,242.985417987428,25.1889274550538)) ;
#107183=CARTESIAN_POINT('Ctrl Pts',(64.7902651077865,242.985417987428,25.1889274550538)) ;
#107184=CARTESIAN_POINT('Origin',(64.7902651077865,245.878117316722,24.0913131340507)) ;
#107185=CARTESIAN_POINT('',(64.7902651077865,243.367543770797,25.0647672615988)) ;
#107186=CARTESIAN_POINT('',(64.7902651077865,245.924469865878,24.233971611495)) ;
#107187=CARTESIAN_POINT('',(64.9402651077865,243.452279656475,24.8795155697285)) ;
#107188=CARTESIAN_POINT('',(64.9402651077865,245.878117316722,24.0913131340507)) ;
#107189=CARTESIAN_POINT('Ctrl Pts',(64.9402651077865,243.452279656475,24.8795155697285)) ;
#107190=CARTESIAN_POINT('Ctrl Pts',(64.9402651077865,243.451946626863,24.8802305456133)) ;
#107191=CARTESIAN_POINT('Ctrl Pts',(64.940261777681,243.451613653127,24.8809455537216)) ;
#107192=CARTESIAN_POINT('Ctrl Pts',(64.9400834366345,243.442701746765,24.9000865264632)) ;
#107193=CARTESIAN_POINT('Ctrl Pts',(64.9376982652988,243.434129874892,24.9186005211265)) ;
#107194=CARTESIAN_POINT('Ctrl Pts',(64.9285249168183,243.417947439168,24.9537361257337)) ;
#107195=CARTESIAN_POINT('Ctrl Pts',(64.9218878905886,243.410239816549,24.9705605654438)) ;
#107196=CARTESIAN_POINT('Ctrl Pts',(64.9030518920066,243.395163543695,25.0036148517979)) ;
#107197=CARTESIAN_POINT('Ctrl Pts',(64.8902415596279,243.387856735537,25.0197271316055)) ;
#107198=CARTESIAN_POINT('Ctrl Pts',(64.8622234505159,243.377274235219,25.0431407641495)) ;
#107199=CARTESIAN_POINT('Ctrl Pts',(64.8483068832618,243.373501577211,25.0515181361211)) ;
#107200=CARTESIAN_POINT('Ctrl Pts',(64.8193104176513,243.368733650287,25.0621166715429)) ;
#107201=CARTESIAN_POINT('Ctrl Pts',(64.8049443310403,243.367543770797,25.0647672615988)) ;
#107202=CARTESIAN_POINT('Ctrl Pts',(64.7902651077865,243.367543770797,25.0647672615988)) ;
#107203=CARTESIAN_POINT('Origin',(64.7902651077865,248.040265107786,23.0213203435596)) ;
#107204=CARTESIAN_POINT('',(64.7902651077865,243.640525134035,25.6005233528965)) ;
#107205=CARTESIAN_POINT('Origin',(64.7902651077865,248.040265107786,23.0213203435596)) ;
#107206=CARTESIAN_POINT('',(64.9402651077865,243.840203404936,25.6408587937931)) ;
#107207=CARTESIAN_POINT('Origin',(64.9402651077865,248.040265107786,23.0213203435596)) ;
#107208=CARTESIAN_POINT('Ctrl Pts',(64.9402651077865,243.840203404936,25.6408587937931)) ;
#107209=CARTESIAN_POINT('Ctrl Pts',(64.9402651077865,243.839429227398,25.6407079681274)) ;
#107210=CARTESIAN_POINT('Ctrl Pts',(64.9402617776811,243.83865505664,25.6405570783186)) ;
#107211=CARTESIAN_POINT('Ctrl Pts',(64.9400834366345,243.817931397271,25.6365161805243)) ;
#107212=CARTESIAN_POINT('Ctrl Pts',(64.9376982652987,243.797914841084,25.6325687175194)) ;
#107213=CARTESIAN_POINT('Ctrl Pts',(64.9285249168183,243.759977742785,25.6250083928119)) ;
#107214=CARTESIAN_POINT('Ctrl Pts',(64.9218878905886,243.741836058232,25.621354832958)) ;
#107215=CARTESIAN_POINT('Ctrl Pts',(64.9030518920066,243.706232967992,25.6141229718641)) ;
#107216=CARTESIAN_POINT('Ctrl Pts',(64.8902415596279,243.688903025733,25.6105637433868)) ;
#107217=CARTESIAN_POINT('Ctrl Pts',(64.862223450516,243.663740761485,25.6053629780756)) ;
#107218=CARTESIAN_POINT('Ctrl Pts',(64.8483068832619,243.654745812453,25.6034910268201)) ;
#107219=CARTESIAN_POINT('Ctrl Pts',(64.8193104176514,243.643368900052,25.6011186979124)) ;
#107220=CARTESIAN_POINT('Ctrl Pts',(64.8049443310403,243.640525134035,25.6005233528966)) ;
#107221=CARTESIAN_POINT('Ctrl Pts',(64.7902651077865,243.640525134035,25.6005233528966)) ;
#107222=CARTESIAN_POINT('Origin',(64.7902651077865,245.619240674958,24.3483125582154)) ;
#107223=CARTESIAN_POINT('',(64.7902651077865,243.315469527519,25.8366900749965)) ;
#107224=CARTESIAN_POINT('',(64.7902651077865,245.531072887114,24.2269600090591)) ;
#107225=CARTESIAN_POINT('',(64.9402651077865,243.400632319557,25.9602258814026)) ;
#107226=CARTESIAN_POINT('',(64.9402651077865,245.619240674958,24.3483125582154)) ;
#107227=CARTESIAN_POINT('Ctrl Pts',(64.9402651077865,243.400632319557,25.9602258814026)) ;
#107228=CARTESIAN_POINT('Ctrl Pts',(64.9402651077865,243.399807320561,25.9590229387353)) ;
#107229=CARTESIAN_POINT('Ctrl Pts',(64.940243846551,243.398982263143,25.957820129938)) ;
#107230=CARTESIAN_POINT('Ctrl Pts',(64.9402013305491,243.398157412359,25.9566178371379)) ;
#107231=CARTESIAN_POINT('Ctrl Pts',(64.9396551395109,243.387560787867,25.9411723219294)) ;
#107232=CARTESIAN_POINT('Ctrl Pts',(64.9356062703199,243.377098235264,25.9259582673101)) ;
#107233=CARTESIAN_POINT('Ctrl Pts',(64.928263675975,243.36731840212,25.9117600448446)) ;
#107234=CARTESIAN_POINT('Ctrl Pts',(64.9206090302591,243.357122937907,25.8969584151121)) ;
#107235=CARTESIAN_POINT('Ctrl Pts',(64.9095180038062,243.347860571349,25.8835376386856)) ;
#107236=CARTESIAN_POINT('Ctrl Pts',(64.8956136387305,243.340061292121,25.8722475987307)) ;
#107237=CARTESIAN_POINT('Ctrl Pts',(64.8817129938793,243.332264099653,25.8609605795167)) ;
#107238=CARTESIAN_POINT('Ctrl Pts',(64.8652664191737,243.326078599533,25.8520189483946)) ;
#107239=CARTESIAN_POINT('Ctrl Pts',(64.8471986491033,243.321859600104,25.845921961251)) ;
#107240=CARTESIAN_POINT('Ctrl Pts',(64.8291331055125,243.31764112058,25.8398257254351)) ;
#107241=CARTESIAN_POINT('Ctrl Pts',(64.8097925816885,243.315469527519,25.8366900749965)) ;
#107242=CARTESIAN_POINT('Ctrl Pts',(64.7902651077865,243.31546952752,25.836690074996)) ;
#107243=CARTESIAN_POINT('Origin',(64.7902651077865,243.590671638724,26.2541392311682)) ;
#107244=CARTESIAN_POINT('',(64.7902651077865,243.902647249673,26.6448708758722)) ;
#107245=CARTESIAN_POINT('Origin',(64.7902651077865,243.590671638724,26.2541392311682)) ;
#107246=CARTESIAN_POINT('',(64.9402651077865,243.811474466023,26.5257015839659)) ;
#107247=CARTESIAN_POINT('Origin',(64.9402651077865,243.590671638724,26.2541392311682)) ;
#107248=CARTESIAN_POINT('Ctrl Pts',(64.9402651077865,243.811474466023,26.5257015839661)) ;
#107249=CARTESIAN_POINT('Ctrl Pts',(64.9402651077865,243.812363593775,26.5268579343641)) ;
#107250=CARTESIAN_POINT('Ctrl Pts',(64.940243846551,243.813252576156,26.5280142989584)) ;
#107251=CARTESIAN_POINT('Ctrl Pts',(64.9402013305491,243.814141131648,26.5291703075783)) ;
#107252=CARTESIAN_POINT('Ctrl Pts',(64.9396551395109,243.82555615249,26.5440212230313)) ;
#107253=CARTESIAN_POINT('Ctrl Pts',(64.9356062703199,243.836792471709,26.5586731032994)) ;
#107254=CARTESIAN_POINT('Ctrl Pts',(64.928263675975,243.847273649061,26.5723617693703)) ;
#107255=CARTESIAN_POINT('Ctrl Pts',(64.9206090302593,243.858200263763,26.586632187178)) ;
#107256=CARTESIAN_POINT('Ctrl Pts',(64.9095180038064,243.868101951963,26.5995884692429)) ;
#107257=CARTESIAN_POINT('Ctrl Pts',(64.8956136387305,243.876429308206,26.6104948387885)) ;
#107258=CARTESIAN_POINT('Ctrl Pts',(64.8817129938791,243.884754436398,26.6213982902475)) ;
#107259=CARTESIAN_POINT('Ctrl Pts',(64.8652664191736,243.891347008287,26.6300441664173)) ;
#107260=CARTESIAN_POINT('Ctrl Pts',(64.8471986491033,243.895841845116,26.6359407459585)) ;
#107261=CARTESIAN_POINT('Ctrl Pts',(64.8291331055124,243.90033612805,26.6418365988681)) ;
#107262=CARTESIAN_POINT('Ctrl Pts',(64.8097925816883,243.902647249673,26.6448708758722)) ;
#107263=CARTESIAN_POINT('Ctrl Pts',(64.7902651077866,243.902647249673,26.6448708758723)) ;
#107264=CARTESIAN_POINT('Origin',(64.7902651077865,246.314586318022,24.7070843711341)) ;
#107265=CARTESIAN_POINT('',(64.7902651077865,244.227702856188,26.4087041537722)) ;
#107266=CARTESIAN_POINT('',(64.7902651077865,246.402754105866,24.8284369202904)) ;
#107267=CARTESIAN_POINT('',(64.9402651077865,244.251045551402,26.2063344963562)) ;
#107268=CARTESIAN_POINT('',(64.9402651077865,246.314586318022,24.7070843711341)) ;
#107269=CARTESIAN_POINT('Ctrl Pts',(64.9402651077865,244.251045551402,26.2063344963562)) ;
#107270=CARTESIAN_POINT('Ctrl Pts',(64.9402651077865,244.250949761119,26.2071173906402)) ;
#107271=CARTESIAN_POINT('Ctrl Pts',(64.940261777681,244.250854033933,26.2079002983041)) ;
#107272=CARTESIAN_POINT('Ctrl Pts',(64.9400834366345,244.248293193181,26.228858375676)) ;
#107273=CARTESIAN_POINT('Ctrl Pts',(64.9376982652988,244.245861997565,26.2491150850256)) ;
#107274=CARTESIAN_POINT('Ctrl Pts',(64.9285249168183,244.241329085551,26.2875316783901)) ;
#107275=CARTESIAN_POINT('Ctrl Pts',(64.9218878905887,244.239197738625,26.3059144577853)) ;
#107276=CARTESIAN_POINT('Ctrl Pts',(64.9030518920066,244.235073687307,26.3420097767375)) ;
#107277=CARTESIAN_POINT('Ctrl Pts',(64.8902415596279,244.233103468073,26.3595913933363)) ;
#107278=CARTESIAN_POINT('Ctrl Pts',(64.862223450516,244.230274122543,26.3851292535788)) ;
#107279=CARTESIAN_POINT('Ctrl Pts',(64.8483068832619,244.229274861868,26.3942624232202)) ;
#107280=CARTESIAN_POINT('Ctrl Pts',(64.8193104176513,244.228015421459,26.4058155998437)) ;
#107281=CARTESIAN_POINT('Ctrl Pts',(64.8049443310403,244.227702856188,26.4087041537722)) ;
#107282=CARTESIAN_POINT('Ctrl Pts',(64.7902651077865,244.227702856188,26.4087041537722)) ;
#107283=CARTESIAN_POINT('Origin',(64.7902651077865,248.040265107786,23.0213203435596)) ;
#107284=CARTESIAN_POINT('',(64.7902651077865,244.652881297574,26.8338825951576)) ;
#107285=CARTESIAN_POINT('Origin',(64.7902651077865,248.040265107786,23.0213203435596)) ;
#107286=CARTESIAN_POINT('',(64.9402651077865,244.85525095499,26.8105398999439)) ;
#107287=CARTESIAN_POINT('Origin',(64.9402651077865,248.040265107786,23.0213203435596)) ;
#107288=CARTESIAN_POINT('Ctrl Pts',(64.9402651077865,244.85525095499,26.8105398999439)) ;
#107289=CARTESIAN_POINT('Ctrl Pts',(64.9402651077865,244.854468060706,26.8106356902274)) ;
#107290=CARTESIAN_POINT('Ctrl Pts',(64.940261777681,244.853685153042,26.8107314174129)) ;
#107291=CARTESIAN_POINT('Ctrl Pts',(64.9400834366345,244.832727075669,26.8132922581644)) ;
#107292=CARTESIAN_POINT('Ctrl Pts',(64.9376982652987,244.81247036632,26.8157234537813)) ;
#107293=CARTESIAN_POINT('Ctrl Pts',(64.9285249168183,244.774053772956,26.8202563657947)) ;
#107294=CARTESIAN_POINT('Ctrl Pts',(64.9218878905887,244.755670993561,26.8223877127213)) ;
#107295=CARTESIAN_POINT('Ctrl Pts',(64.9030518920066,244.719575674608,26.8265117640394)) ;
#107296=CARTESIAN_POINT('Ctrl Pts',(64.890241559628,244.70199405801,26.8284819832727)) ;
#107297=CARTESIAN_POINT('Ctrl Pts',(64.862223450516,244.676456197767,26.8313113288033)) ;
#107298=CARTESIAN_POINT('Ctrl Pts',(64.8483068832619,244.667323028126,26.832310589478)) ;
#107299=CARTESIAN_POINT('Ctrl Pts',(64.8193104176514,244.655769851502,26.8335700298872)) ;
#107300=CARTESIAN_POINT('Ctrl Pts',(64.8049443310404,244.652881297574,26.8338825951576)) ;
#107301=CARTESIAN_POINT('Ctrl Pts',(64.7902651077866,244.652881297574,26.8338825951576)) ;
#107302=CARTESIAN_POINT('Origin',(64.7902651077865,246.147797190567,25.0315026299217)) ;
#107303=CARTESIAN_POINT('',(64.7902651077865,244.416714575474,27.1589382016729)) ;
#107304=CARTESIAN_POINT('',(64.7902651077865,246.026444641411,24.9433348420779)) ;
#107305=CARTESIAN_POINT('',(64.9402651077865,244.53588386738,27.2501109853235)) ;
#107306=CARTESIAN_POINT('',(64.9402651077865,246.147797190567,25.0315026299217)) ;
#107307=CARTESIAN_POINT('Ctrl Pts',(64.9402651077865,244.53588386738,27.2501109853235)) ;
#107308=CARTESIAN_POINT('Ctrl Pts',(64.9402651077865,244.534727516982,27.2492218575712)) ;
#107309=CARTESIAN_POINT('Ctrl Pts',(64.940243846551,244.533571152388,27.2483328751903)) ;
#107310=CARTESIAN_POINT('Ctrl Pts',(64.9402013305491,244.532415143768,27.2474443196982)) ;
#107311=CARTESIAN_POINT('Ctrl Pts',(64.9396551395109,244.51756422831,27.2360292988605)) ;
#107312=CARTESIAN_POINT('Ctrl Pts',(64.9356062703199,244.502912348047,27.2247929796359)) ;
#107313=CARTESIAN_POINT('Ctrl Pts',(64.9282636759751,244.489223681976,27.2143118022837)) ;
#107314=CARTESIAN_POINT('Ctrl Pts',(64.9206090302593,244.474953264168,27.2033851875822)) ;
#107315=CARTESIAN_POINT('Ctrl Pts',(64.9095180038062,244.461996982103,27.1934834993823)) ;
#107316=CARTESIAN_POINT('Ctrl Pts',(64.8956136387306,244.451090612558,27.1851561431395)) ;
#107317=CARTESIAN_POINT('Ctrl Pts',(64.8817129938794,244.440187161099,27.1768310149477)) ;
#107318=CARTESIAN_POINT('Ctrl Pts',(64.8652664191739,244.431541284929,27.1702384430589)) ;
#107319=CARTESIAN_POINT('Ctrl Pts',(64.8471986491033,244.425644705387,27.1657436062292)) ;
#107320=CARTESIAN_POINT('Ctrl Pts',(64.8291331055124,244.419748852478,27.1612493232953)) ;
#107321=CARTESIAN_POINT('Ctrl Pts',(64.8097925816884,244.416714575474,27.1589382016726)) ;
#107322=CARTESIAN_POINT('Ctrl Pts',(64.7902651077865,244.416714575474,27.1589382016725)) ;
#107323=CARTESIAN_POINT('Origin',(64.7902651077865,244.807446220178,27.4709138126218)) ;
#107324=CARTESIAN_POINT('',(64.7902651077865,245.224895376349,27.7461159238265)) ;
#107325=CARTESIAN_POINT('Origin',(64.7902651077865,244.807446220178,27.4709138126218)) ;
#107326=CARTESIAN_POINT('',(64.9402651077865,245.101359569943,27.6609531317891)) ;
#107327=CARTESIAN_POINT('Origin',(64.9402651077865,244.807446220178,27.4709138126218)) ;
#107328=CARTESIAN_POINT('Ctrl Pts',(64.9402651077865,245.101359569948,27.6609531317925)) ;
#107329=CARTESIAN_POINT('Ctrl Pts',(64.9402651077864,245.102562512614,27.6617781307873)) ;
#107330=CARTESIAN_POINT('Ctrl Pts',(64.9402438465509,245.10376532141,27.6626031882038)) ;
#107331=CARTESIAN_POINT('Ctrl Pts',(64.9402013305491,245.104967614209,27.663428038987)) ;
#107332=CARTESIAN_POINT('Ctrl Pts',(64.9396551395108,245.120413129416,27.6740246634796)) ;
#107333=CARTESIAN_POINT('Ctrl Pts',(64.9356062703197,245.135627184036,27.6844872160823)) ;
#107334=CARTESIAN_POINT('Ctrl Pts',(64.9282636759749,245.149825406501,27.6942670492256)) ;
#107335=CARTESIAN_POINT('Ctrl Pts',(64.9206090302591,245.164627036234,27.7044625134384)) ;
#107336=CARTESIAN_POINT('Ctrl Pts',(64.9095180038063,245.17804781266,27.7137248799967)) ;
#107337=CARTESIAN_POINT('Ctrl Pts',(64.8956136387305,245.189337852615,27.7215241592249)) ;
#107338=CARTESIAN_POINT('Ctrl Pts',(64.8817129938791,245.200624871829,27.7293213516933)) ;
#107339=CARTESIAN_POINT('Ctrl Pts',(64.8652664191736,245.209566502951,27.7355068518133)) ;
#107340=CARTESIAN_POINT('Ctrl Pts',(64.8471986491032,245.215663490095,27.7397258512423)) ;
#107341=CARTESIAN_POINT('Ctrl Pts',(64.8291331055125,245.22175972591,27.7439443307667)) ;
#107342=CARTESIAN_POINT('Ctrl Pts',(64.8097925816882,245.224895376349,27.7461159238267)) ;
#107343=CARTESIAN_POINT('Ctrl Pts',(64.7902651077865,245.22489537635,27.7461159238262)) ;
#107344=CARTESIAN_POINT('Origin',(64.7902651077865,246.919976782775,25.1578412797899)) ;
#107345=CARTESIAN_POINT('',(64.7902651077865,247.041329331931,25.2460090676338)) ;
#107346=CARTESIAN_POINT('',(64.9402651077865,246.919976782775,25.1578412797899)) ;
#107347=CARTESIAN_POINT('Origin',(60.4402651077865,250.207872219281,17.9664732232009)) ;
#107348=CARTESIAN_POINT('',(60.5902651077865,250.207872219281,17.9664732232009)) ;
#107349=CARTESIAN_POINT('',(60.4402651077865,250.207872219281,17.9664732232009)) ;
#107350=CARTESIAN_POINT('',(60.5902651077865,250.083712025826,18.3485990065702)) ;
#107351=CARTESIAN_POINT('',(60.5902651077865,249.361587041504,20.5710711826001)) ;
#107352=CARTESIAN_POINT('',(60.4402651077865,250.083712025826,18.3485990065702)) ;
#107353=CARTESIAN_POINT('Origin',(60.4402651077865,249.739858576849,17.7905095039363)) ;
#107354=CARTESIAN_POINT('',(60.5902651077865,249.257798707399,17.6577756263215)) ;
#107355=CARTESIAN_POINT('',(60.4402651077865,249.257798707399,17.6577756263215)) ;
#107356=CARTESIAN_POINT('Origin',(60.5902651077865,249.739858576849,17.7905095039363)) ;
#107357=CARTESIAN_POINT('Origin',(60.4402651077865,249.040457375835,18.3266834644245)) ;
#107358=CARTESIAN_POINT('',(60.5902651077865,249.133638513944,18.0399014096908)) ;
#107359=CARTESIAN_POINT('',(60.4402651077865,249.133638513944,18.0399014096908)) ;
#107360=CARTESIAN_POINT('',(60.5902651077865,248.30284286384,20.5968275047722)) ;
#107361=CARTESIAN_POINT('Origin',(60.4402651077865,248.040265107786,23.0213203435596)) ;
#107362=CARTESIAN_POINT('',(60.5902651077865,248.539748311783,17.9458384424072)) ;
#107363=CARTESIAN_POINT('',(60.4402651077865,248.539748311783,17.9458384424072)) ;
#107364=CARTESIAN_POINT('Origin',(60.5902651077865,248.040265107786,23.0213203435596)) ;
#107365=CARTESIAN_POINT('Origin',(60.4402651077865,248.539748311783,17.5440476162869)) ;
#107366=CARTESIAN_POINT('',(60.5902651077865,248.539748311783,17.5440476162869)) ;
#107367=CARTESIAN_POINT('',(60.4402651077865,248.539748311783,17.5440476162869)) ;
#107368=CARTESIAN_POINT('',(60.5902651077865,248.539748311783,20.2826839799233)) ;
#107369=CARTESIAN_POINT('Origin',(60.4402651077865,248.040265107786,17.5213203435596)) ;
#107370=CARTESIAN_POINT('',(60.5902651077865,247.54078190379,17.5440476162869)) ;
#107371=CARTESIAN_POINT('',(60.4402651077865,247.54078190379,17.5440476162869)) ;
#107372=CARTESIAN_POINT('Origin',(60.5902651077865,248.040265107786,17.5213203435596)) ;
#107373=CARTESIAN_POINT('Origin',(60.4402651077865,247.54078190379,18.2473789395491)) ;
#107374=CARTESIAN_POINT('',(60.5902651077865,247.54078190379,17.9458384424072)) ;
#107375=CARTESIAN_POINT('',(60.4402651077865,247.54078190379,17.9458384424072)) ;
#107376=CARTESIAN_POINT('',(60.5902651077865,247.54078190379,20.6343496415544)) ;
#107377=CARTESIAN_POINT('Origin',(60.4402651077865,248.040265107786,23.0213203435596)) ;
#107378=CARTESIAN_POINT('',(60.5902651077865,246.946891701628,18.0399014096908)) ;
#107379=CARTESIAN_POINT('',(60.4402651077865,246.946891701628,18.0399014096908)) ;
#107380=CARTESIAN_POINT('Origin',(60.5902651077865,248.040265107786,23.0213203435596)) ;
#107381=CARTESIAN_POINT('Origin',(60.4402651077865,246.822731508173,17.6577756263215)) ;
#107382=CARTESIAN_POINT('',(60.5902651077865,246.822731508173,17.6577756263215)) ;
#107383=CARTESIAN_POINT('',(60.4402651077865,246.822731508173,17.6577756263215)) ;
#107384=CARTESIAN_POINT('',(60.5902651077865,247.66901668595,20.2623735857207)) ;
#107385=CARTESIAN_POINT('Origin',(60.4402651077865,246.340671638724,17.7905095039363)) ;
#107386=CARTESIAN_POINT('',(60.5902651077865,245.872657996292,17.9664732232009)) ;
#107387=CARTESIAN_POINT('',(60.4402651077865,245.872657996292,17.9664732232009)) ;
#107388=CARTESIAN_POINT('Origin',(60.5902651077865,246.340671638724,17.7905095039363)) ;
#107389=CARTESIAN_POINT('Origin',(60.4402651077865,246.089999327856,18.6353810613039)) ;
#107390=CARTESIAN_POINT('',(60.5902651077865,245.996818189747,18.3485990065702)) ;
#107391=CARTESIAN_POINT('',(60.4402651077865,245.996818189747,18.3485990065702)) ;
#107392=CARTESIAN_POINT('',(60.5902651077865,246.827613839851,20.9055251016516)) ;
#107393=CARTESIAN_POINT('Origin',(60.4402651077865,248.040265107786,23.0213203435596)) ;
#107394=CARTESIAN_POINT('',(60.5902651077865,245.461062098449,18.6215803698081)) ;
#107395=CARTESIAN_POINT('',(60.4402651077865,245.461062098449,18.6215803698081)) ;
#107396=CARTESIAN_POINT('Origin',(60.5902651077865,248.040265107786,23.0213203435596)) ;
#107397=CARTESIAN_POINT('Origin',(60.4402651077865,245.224895376349,18.2965247632928)) ;
#107398=CARTESIAN_POINT('',(60.5902651077865,245.224895376349,18.2965247632928)) ;
#107399=CARTESIAN_POINT('',(60.4402651077865,245.224895376349,18.2965247632928)) ;
#107400=CARTESIAN_POINT('',(60.5902651077865,246.834625442287,20.5121281228878)) ;
#107401=CARTESIAN_POINT('Origin',(60.4402651077865,244.807446220178,18.5717268744974)) ;
#107402=CARTESIAN_POINT('',(60.5902651077865,244.416714575474,18.8837024854464)) ;
#107403=CARTESIAN_POINT('',(60.4402651077865,244.416714575474,18.8837024854464)) ;
#107404=CARTESIAN_POINT('Origin',(60.5902651077865,244.807446220178,18.5717268744974)) ;
#107405=CARTESIAN_POINT('Origin',(60.4402651077865,244.830122354763,19.4527094786418)) ;
#107406=CARTESIAN_POINT('',(60.5902651077865,244.652881297574,19.2087580919617)) ;
#107407=CARTESIAN_POINT('',(60.4402651077865,244.652881297574,19.2087580919617)) ;
#107408=CARTESIAN_POINT('',(60.5902651077865,246.233148531056,21.3838093416391)) ;
#107409=CARTESIAN_POINT('Origin',(60.4402651077865,248.040265107786,23.0213203435596)) ;
#107410=CARTESIAN_POINT('',(60.5902651077865,244.227702856188,19.633936533347)) ;
#107411=CARTESIAN_POINT('',(60.4402651077865,244.227702856188,19.633936533347)) ;
#107412=CARTESIAN_POINT('Origin',(60.5902651077865,248.040265107786,23.0213203435596)) ;
#107413=CARTESIAN_POINT('Origin',(60.4402651077865,243.902647249673,19.3977698112471)) ;
#107414=CARTESIAN_POINT('',(60.5902651077865,243.902647249673,19.3977698112471)) ;
#107415=CARTESIAN_POINT('',(60.4402651077865,243.902647249673,19.3977698112471)) ;
#107416=CARTESIAN_POINT('',(60.5902651077865,246.118250609268,21.0074998771845)) ;
#107417=CARTESIAN_POINT('Origin',(60.4402651077865,243.590671638724,19.788501455951)) ;
#107418=CARTESIAN_POINT('',(60.5902651077865,243.315469527519,20.2059506121228)) ;
#107419=CARTESIAN_POINT('',(60.4402651077865,243.315469527519,20.2059506121228)) ;
#107420=CARTESIAN_POINT('Origin',(60.5902651077865,243.590671638724,19.788501455951)) ;
#107421=CARTESIAN_POINT('Origin',(60.4402651077865,243.884476520715,20.6193583914117)) ;
#107422=CARTESIAN_POINT('',(60.5902651077865,243.640525134035,20.4421173342227)) ;
#107423=CARTESIAN_POINT('',(60.4402651077865,243.640525134035,20.4421173342227)) ;
#107424=CARTESIAN_POINT('',(60.5902651077865,245.815576383712,22.0223845677046)) ;
#107425=CARTESIAN_POINT('Origin',(60.4402651077865,248.040265107786,23.0213203435596)) ;
#107426=CARTESIAN_POINT('',(60.5902651077865,243.367543770797,20.9778734255204)) ;
#107427=CARTESIAN_POINT('',(60.4402651077865,243.367543770797,20.9778734255204)) ;
#107428=CARTESIAN_POINT('Origin',(60.5902651077865,248.040265107786,23.0213203435596)) ;
#107429=CARTESIAN_POINT('Origin',(60.4402651077865,242.985417987428,20.8537132320653)) ;
#107430=CARTESIAN_POINT('',(60.5902651077865,242.985417987428,20.8537132320653)) ;
#107431=CARTESIAN_POINT('',(60.4402651077865,242.985417987428,20.8537132320653)) ;
#107432=CARTESIAN_POINT('',(60.5902651077865,245.590015946827,21.6999984098422)) ;
#107433=CARTESIAN_POINT('Origin',(60.4402651077865,242.809454268163,21.3217268744974)) ;
#107434=CARTESIAN_POINT('',(60.5902651077865,242.676720390548,21.8037867439466)) ;
#107435=CARTESIAN_POINT('',(60.4402651077865,242.676720390548,21.8037867439466)) ;
#107436=CARTESIAN_POINT('Origin',(60.5902651077865,242.809454268163,21.3217268744974)) ;
#107437=CARTESIAN_POINT('Origin',(60.4402651077865,243.345628228651,22.0211280755108)) ;
#107438=CARTESIAN_POINT('',(60.5902651077865,243.058846173918,21.9279469374017)) ;
#107439=CARTESIAN_POINT('',(60.4402651077865,243.058846173918,21.9279469374017)) ;
#107440=CARTESIAN_POINT('',(60.5902651077865,245.615772268999,22.7587425875056)) ;
#107441=CARTESIAN_POINT('Origin',(60.4402651077865,248.040265107786,23.0213203435596)) ;
#107442=CARTESIAN_POINT('',(60.5902651077865,242.964783206634,22.5218371395634)) ;
#107443=CARTESIAN_POINT('',(60.4402651077865,242.964783206634,22.5218371395634)) ;
#107444=CARTESIAN_POINT('Origin',(60.5902651077865,248.040265107786,23.0213203435596)) ;
#107445=CARTESIAN_POINT('Origin',(60.4402651077865,242.562992380514,22.5218371395634)) ;
#107446=CARTESIAN_POINT('',(60.5902651077865,242.562992380514,22.5218371395634)) ;
#107447=CARTESIAN_POINT('',(60.4402651077865,242.562992380514,22.5218371395634)) ;
#107448=CARTESIAN_POINT('',(60.5902651077865,245.30162874415,22.5218371395634)) ;
#107449=CARTESIAN_POINT('Origin',(60.4402651077865,242.540265107786,23.0213203435596)) ;
#107450=CARTESIAN_POINT('',(60.5902651077865,242.562992380514,23.5208035475559)) ;
#107451=CARTESIAN_POINT('',(60.4402651077865,242.562992380514,23.5208035475559)) ;
#107452=CARTESIAN_POINT('Origin',(60.5902651077865,242.540265107786,23.0213203435596)) ;
#107453=CARTESIAN_POINT('Origin',(60.4402651077865,243.266323703776,23.5208035475559)) ;
#107454=CARTESIAN_POINT('',(60.5902651077865,242.964783206634,23.5208035475559)) ;
#107455=CARTESIAN_POINT('',(60.4402651077865,242.964783206634,23.5208035475559)) ;
#107456=CARTESIAN_POINT('',(60.5902651077865,245.653294405781,23.5208035475559)) ;
#107457=CARTESIAN_POINT('Origin',(60.4402651077865,248.040265107786,23.0213203435596)) ;
#107458=CARTESIAN_POINT('',(60.5902651077865,243.058846173918,24.1146937497175)) ;
#107459=CARTESIAN_POINT('',(60.4402651077865,243.058846173918,24.1146937497175)) ;
#107460=CARTESIAN_POINT('Origin',(60.5902651077865,248.040265107786,23.0213203435596)) ;
#107461=CARTESIAN_POINT('Origin',(60.4402651077865,242.676720390548,24.2388539431727)) ;
#107462=CARTESIAN_POINT('',(60.5902651077865,242.676720390548,24.2388539431727)) ;
#107463=CARTESIAN_POINT('',(60.4402651077865,242.676720390548,24.2388539431727)) ;
#107464=CARTESIAN_POINT('',(60.5902651077865,245.281318349947,23.3925687653958)) ;
#107465=CARTESIAN_POINT('Origin',(60.4402651077865,242.809454268163,24.7209138126218)) ;
#107466=CARTESIAN_POINT('',(60.5902651077865,242.985417987428,25.188927455054)) ;
#107467=CARTESIAN_POINT('',(60.4402651077865,242.985417987428,25.188927455054)) ;
#107468=CARTESIAN_POINT('Origin',(60.5902651077865,242.809454268163,24.7209138126218)) ;
#107469=CARTESIAN_POINT('Origin',(60.4402651077865,243.654325825531,24.9715861234897)) ;
#107470=CARTESIAN_POINT('',(60.5902651077865,243.367543770797,25.0647672615988)) ;
#107471=CARTESIAN_POINT('',(60.4402651077865,243.367543770797,25.0647672615988)) ;
#107472=CARTESIAN_POINT('',(60.5902651077865,245.924469865878,24.233971611495)) ;
#107473=CARTESIAN_POINT('Origin',(60.4402651077865,248.040265107786,23.0213203435596)) ;
#107474=CARTESIAN_POINT('',(60.5902651077865,243.640525134035,25.6005233528965)) ;
#107475=CARTESIAN_POINT('',(60.4402651077865,243.640525134035,25.6005233528965)) ;
#107476=CARTESIAN_POINT('Origin',(60.5902651077865,248.040265107786,23.0213203435596)) ;
#107477=CARTESIAN_POINT('Origin',(60.4402651077865,243.315469527519,25.8366900749965)) ;
#107478=CARTESIAN_POINT('',(60.5902651077865,243.315469527519,25.8366900749965)) ;
#107479=CARTESIAN_POINT('',(60.4402651077865,243.315469527519,25.8366900749965)) ;
#107480=CARTESIAN_POINT('',(60.5902651077865,245.531072887114,24.2269600090591)) ;
#107481=CARTESIAN_POINT('Origin',(60.4402651077865,243.590671638724,26.2541392311682)) ;
#107482=CARTESIAN_POINT('',(60.5902651077865,243.902647249673,26.6448708758722)) ;
#107483=CARTESIAN_POINT('',(60.4402651077865,243.902647249673,26.6448708758722)) ;
#107484=CARTESIAN_POINT('Origin',(60.5902651077865,243.590671638724,26.2541392311682)) ;
#107485=CARTESIAN_POINT('Origin',(60.4402651077865,244.471654242868,26.2314630965833)) ;
#107486=CARTESIAN_POINT('',(60.5902651077865,244.227702856188,26.4087041537722)) ;
#107487=CARTESIAN_POINT('',(60.4402651077865,244.227702856188,26.4087041537722)) ;
#107488=CARTESIAN_POINT('',(60.5902651077865,246.402754105866,24.8284369202904)) ;
#107489=CARTESIAN_POINT('Origin',(60.4402651077865,248.040265107786,23.0213203435596)) ;
#107490=CARTESIAN_POINT('',(60.5902651077865,244.652881297574,26.8338825951576)) ;
#107491=CARTESIAN_POINT('',(60.4402651077865,244.652881297574,26.8338825951576)) ;
#107492=CARTESIAN_POINT('Origin',(60.5902651077865,248.040265107786,23.0213203435596)) ;
#107493=CARTESIAN_POINT('Origin',(60.4402651077865,244.416714575474,27.1589382016729)) ;
#107494=CARTESIAN_POINT('',(60.5902651077865,244.416714575474,27.1589382016729)) ;
#107495=CARTESIAN_POINT('',(60.4402651077865,244.416714575474,27.1589382016729)) ;
#107496=CARTESIAN_POINT('',(60.5902651077865,246.026444641411,24.9433348420779)) ;
#107497=CARTESIAN_POINT('Origin',(60.4402651077865,244.807446220178,27.4709138126218)) ;
#107498=CARTESIAN_POINT('',(60.5902651077865,245.224895376349,27.7461159238265)) ;
#107499=CARTESIAN_POINT('',(60.4402651077865,245.224895376349,27.7461159238265)) ;
#107500=CARTESIAN_POINT('Origin',(60.5902651077865,244.807446220178,27.4709138126218)) ;
#107501=CARTESIAN_POINT('Origin',(60.4402651077865,245.638303155638,27.1771089306311)) ;
#107502=CARTESIAN_POINT('',(60.5902651077865,245.461062098449,27.4210603173112)) ;
#107503=CARTESIAN_POINT('',(60.4402651077865,245.461062098449,27.4210603173112)) ;
#107504=CARTESIAN_POINT('',(60.5902651077865,247.041329331931,25.2460090676338)) ;
#107505=CARTESIAN_POINT('Origin',(60.4402651077865,248.040265107786,23.0213203435596)) ;
#107506=CARTESIAN_POINT('',(60.5902651077865,245.996818189747,27.694041680549)) ;
#107507=CARTESIAN_POINT('',(60.4402651077865,245.996818189747,27.694041680549)) ;
#107508=CARTESIAN_POINT('Origin',(60.5902651077865,248.040265107786,23.0213203435596)) ;
#107509=CARTESIAN_POINT('Origin',(64.9402651077865,248.040265107786,23.0213203435596)) ;
#107510=CARTESIAN_POINT('Origin',(64.9402651077865,248.040265107786,23.0213203435596)) ;
#107511=CARTESIAN_POINT('Origin',(64.9402651077865,248.040265107786,23.0213203435596)) ;
#107512=CARTESIAN_POINT('Origin',(64.9402651077865,248.040265107786,23.0213203435596)) ;
#107513=CARTESIAN_POINT('Origin',(64.9402651077865,248.040265107786,23.0213203435596)) ;
#107514=CARTESIAN_POINT('Origin',(64.9402651077865,248.040265107786,23.0213203435596)) ;
#107515=CARTESIAN_POINT('Origin',(64.9402651077865,248.040265107786,23.0213203435596)) ;
#107516=CARTESIAN_POINT('Origin',(64.9402651077865,248.040265107786,23.0213203435596)) ;
#107517=CARTESIAN_POINT('Origin',(64.9402651077865,248.040265107786,23.0213203435596)) ;
#107518=CARTESIAN_POINT('Origin',(64.9402651077865,248.040265107786,23.0213203435596)) ;
#107519=CARTESIAN_POINT('Origin',(64.9402651077865,248.040265107786,23.0213203435596)) ;
#107520=CARTESIAN_POINT('Origin',(64.9402651077865,248.040265107786,23.0213203435596)) ;
#107521=CARTESIAN_POINT('Origin',(64.9402651077865,248.040265107786,23.0213203435596)) ;
#107522=CARTESIAN_POINT('Origin',(64.9402651077865,248.040265107786,23.0213203435596)) ;
#107523=CARTESIAN_POINT('Origin',(64.9402651077865,248.040265107786,23.0213203435596)) ;
#107524=CARTESIAN_POINT('Origin',(64.9402651077865,248.040265107786,23.0213203435596)) ;
#107525=CARTESIAN_POINT('Origin',(64.9402651077865,248.040265107786,23.0213203435596)) ;
#107526=CARTESIAN_POINT('Origin',(64.9402651077865,248.040265107786,23.0213203435596)) ;
#107527=CARTESIAN_POINT('Origin',(64.9402651077865,248.040265107786,23.0213203435596)) ;
#107528=CARTESIAN_POINT('Origin',(64.9402651077865,248.040265107786,23.0213203435596)) ;
#107529=CARTESIAN_POINT('Origin',(64.9402651077865,248.040265107786,23.0213203435596)) ;
#107530=CARTESIAN_POINT('Origin',(64.9402651077865,248.040265107786,23.0213203435596)) ;
#107531=CARTESIAN_POINT('Origin',(64.9402651077865,248.040265107786,23.0213203435596)) ;
#107532=CARTESIAN_POINT('Origin',(64.9402651077865,248.040265107786,23.0213203435596)) ;
#107533=CARTESIAN_POINT('Origin',(64.9402651077865,248.040265107786,23.0213203435596)) ;
#107534=CARTESIAN_POINT('Origin',(64.9402651077865,248.040265107786,23.0213203435596)) ;
#107535=CARTESIAN_POINT('Origin',(64.9402651077865,248.040265107786,23.0213203435596)) ;
#107536=CARTESIAN_POINT('Origin',(64.9402651077865,248.040265107786,23.0213203435596)) ;
#107537=CARTESIAN_POINT('Origin',(64.9402651077865,248.040265107786,23.0213203435596)) ;
#107538=CARTESIAN_POINT('Origin',(64.9402651077865,248.040265107786,23.0213203435596)) ;
#107539=CARTESIAN_POINT('Origin',(64.9402651077865,248.040265107786,23.0213203435596)) ;
#107540=CARTESIAN_POINT('Origin',(64.9402651077865,248.040265107786,23.0213203435596)) ;
#107541=CARTESIAN_POINT('Origin',(64.9402651077865,248.040265107786,23.0213203435596)) ;
#107542=CARTESIAN_POINT('Origin',(64.9402651077865,248.040265107786,23.0213203435596)) ;
#107543=CARTESIAN_POINT('Origin',(64.9402651077865,248.040265107786,23.0213203435596)) ;
#107544=CARTESIAN_POINT('Origin',(64.9402651077865,248.040265107786,23.0213203435596)) ;
#107545=CARTESIAN_POINT('Origin',(64.9402651077865,248.040265107786,23.0213203435596)) ;
#107546=CARTESIAN_POINT('',(64.9402651077865,248.040265107786,27.9713203435596)) ;
#107547=CARTESIAN_POINT('Origin',(64.9402651077865,248.040265107786,23.0213203435596)) ;
#107548=CARTESIAN_POINT('Origin',(64.9402651077865,248.040265107786,23.0213203435596)) ;
#107549=CARTESIAN_POINT('Origin',(65.0902651077865,248.040265107786,23.0213203435596)) ;
#107550=CARTESIAN_POINT('Origin',(65.0902651077865,248.040265107786,27.9713203435596)) ;
#107551=CARTESIAN_POINT('Origin',(64.9402651077865,248.040265107786,23.0213203435596)) ;
#107552=CARTESIAN_POINT('Origin',(64.9402651077865,248.040265107786,23.0213203435596)) ;
#107553=CARTESIAN_POINT('Origin',(60.2902651077865,248.040265107786,23.0213203435596)) ;
#107554=CARTESIAN_POINT('',(60.4402651077865,248.040265107786,18.0713203435596)) ;
#107555=CARTESIAN_POINT('Origin',(60.2902651077865,248.040265107786,18.0713203435596)) ;
#107556=CARTESIAN_POINT('',(60.4402651077865,247.69078190379,18.0836729796702)) ;
#107557=CARTESIAN_POINT('Origin',(60.4402651077865,248.040265107786,23.0213203435596)) ;
#107558=CARTESIAN_POINT('',(60.4402651077865,246.84682643861,18.2173423936815)) ;
#107559=CARTESIAN_POINT('Origin',(60.4402651077865,248.040265107786,23.0213203435596)) ;
#107560=CARTESIAN_POINT('',(60.4402651077865,246.182069881617,18.4333348922484)) ;
#107561=CARTESIAN_POINT('Origin',(60.4402651077865,248.040265107786,23.0213203435596)) ;
#107562=CARTESIAN_POINT('',(60.4402651077865,245.420726657553,18.8212586407095)) ;
#107563=CARTESIAN_POINT('Origin',(60.4402651077865,248.040265107786,23.0213203435596)) ;
#107564=CARTESIAN_POINT('',(60.4402651077865,244.85525095499,19.2321007871753)) ;
#107565=CARTESIAN_POINT('Origin',(60.4402651077865,248.040265107786,23.0213203435596)) ;
#107566=CARTESIAN_POINT('',(60.4402651077865,244.251045551402,19.836306190763)) ;
#107567=CARTESIAN_POINT('Origin',(60.4402651077865,248.040265107786,23.0213203435596)) ;
#107568=CARTESIAN_POINT('',(60.4402651077865,243.840203404936,20.4017818933262)) ;
#107569=CARTESIAN_POINT('Origin',(60.4402651077865,248.040265107786,23.0213203435596)) ;
#107570=CARTESIAN_POINT('',(60.4402651077865,243.452279656475,21.1631251173908)) ;
#107571=CARTESIAN_POINT('Origin',(60.4402651077865,248.040265107786,23.0213203435596)) ;
#107572=CARTESIAN_POINT('',(60.4402651077865,243.236287157908,21.8278816743835)) ;
#107573=CARTESIAN_POINT('Origin',(60.4402651077865,248.040265107786,23.0213203435596)) ;
#107574=CARTESIAN_POINT('',(60.4402651077865,243.102617743897,22.6718371395634)) ;
#107575=CARTESIAN_POINT('Origin',(60.4402651077865,248.040265107786,23.0213203435596)) ;
#107576=CARTESIAN_POINT('',(60.4402651077865,243.102617743897,23.3708035475559)) ;
#107577=CARTESIAN_POINT('Origin',(60.4402651077865,248.040265107786,23.0213203435596)) ;
#107578=CARTESIAN_POINT('',(60.4402651077865,243.236287157908,24.2147590127358)) ;
#107579=CARTESIAN_POINT('Origin',(60.4402651077865,248.040265107786,23.0213203435596)) ;
#107580=CARTESIAN_POINT('',(60.4402651077865,243.452279656475,24.8795155697285)) ;
#107581=CARTESIAN_POINT('Origin',(60.4402651077865,248.040265107786,23.0213203435596)) ;
#107582=CARTESIAN_POINT('',(60.4402651077865,243.840203404936,25.6408587937931)) ;
#107583=CARTESIAN_POINT('Origin',(60.4402651077865,248.040265107786,23.0213203435596)) ;
#107584=CARTESIAN_POINT('',(60.4402651077865,244.251045551402,26.2063344963562)) ;
#107585=CARTESIAN_POINT('Origin',(60.4402651077865,248.040265107786,23.0213203435596)) ;
#107586=CARTESIAN_POINT('',(60.4402651077865,244.85525095499,26.8105398999439)) ;
#107587=CARTESIAN_POINT('Origin',(60.4402651077865,248.040265107786,23.0213203435596)) ;
#107588=CARTESIAN_POINT('',(60.4402651077865,245.420726657553,27.2213820464098)) ;
#107589=CARTESIAN_POINT('Origin',(60.4402651077865,248.040265107786,23.0213203435596)) ;
#107590=CARTESIAN_POINT('',(60.4402651077865,246.182069881617,27.6093057948708)) ;
#107591=CARTESIAN_POINT('Origin',(60.4402651077865,248.040265107786,23.0213203435596)) ;
#107592=CARTESIAN_POINT('',(60.4402651077865,246.84682643861,27.8252982934377)) ;
#107593=CARTESIAN_POINT('Origin',(60.4402651077865,248.040265107786,23.0213203435596)) ;
#107594=CARTESIAN_POINT('',(60.4402651077865,247.69078190379,27.9589677074491)) ;
#107595=CARTESIAN_POINT('Origin',(60.4402651077865,248.040265107786,23.0213203435596)) ;
#107596=CARTESIAN_POINT('',(60.4402651077865,248.389748311783,27.9589677074491)) ;
#107597=CARTESIAN_POINT('Origin',(60.4402651077865,248.040265107786,23.0213203435596)) ;
#107598=CARTESIAN_POINT('',(60.4402651077865,249.233703776962,27.8252982934377)) ;
#107599=CARTESIAN_POINT('Origin',(60.4402651077865,248.040265107786,23.0213203435596)) ;
#107600=CARTESIAN_POINT('',(60.4402651077865,249.898460333955,27.6093057948708)) ;
#107601=CARTESIAN_POINT('Origin',(60.4402651077865,248.040265107786,23.0213203435596)) ;
#107602=CARTESIAN_POINT('',(60.4402651077865,250.65980355802,27.2213820464098)) ;
#107603=CARTESIAN_POINT('Origin',(60.4402651077865,248.040265107786,23.0213203435596)) ;
#107604=CARTESIAN_POINT('',(60.4402651077865,251.225279260583,26.8105398999439)) ;
#107605=CARTESIAN_POINT('Origin',(60.4402651077865,248.040265107786,23.0213203435596)) ;
#107606=CARTESIAN_POINT('',(60.4402651077865,251.829484664171,26.2063344963563)) ;
#107607=CARTESIAN_POINT('Origin',(60.4402651077865,248.040265107786,23.0213203435596)) ;
#107608=CARTESIAN_POINT('',(60.4402651077865,252.240326810636,25.6408587937931)) ;
#107609=CARTESIAN_POINT('Origin',(60.4402651077865,248.040265107786,23.0213203435596)) ;
#107610=CARTESIAN_POINT('',(60.4402651077865,252.628250559098,24.8795155697285)) ;
#107611=CARTESIAN_POINT('Origin',(60.4402651077865,248.040265107786,23.0213203435596)) ;
#107612=CARTESIAN_POINT('',(60.4402651077865,252.844243057664,24.2147590127358)) ;
#107613=CARTESIAN_POINT('Origin',(60.4402651077865,248.040265107786,23.0213203435596)) ;
#107614=CARTESIAN_POINT('',(60.4402651077865,252.977912471676,23.3708035475559)) ;
#107615=CARTESIAN_POINT('Origin',(60.4402651077865,248.040265107786,23.0213203435596)) ;
#107616=CARTESIAN_POINT('',(60.4402651077865,252.977912471676,22.6718371395634)) ;
#107617=CARTESIAN_POINT('Origin',(60.4402651077865,248.040265107786,23.0213203435596)) ;
#107618=CARTESIAN_POINT('',(60.4402651077865,252.844243057664,21.8278816743835)) ;
#107619=CARTESIAN_POINT('Origin',(60.4402651077865,248.040265107786,23.0213203435596)) ;
#107620=CARTESIAN_POINT('',(60.4402651077865,252.628250559098,21.1631251173908)) ;
#107621=CARTESIAN_POINT('Origin',(60.4402651077865,248.040265107786,23.0213203435596)) ;
#107622=CARTESIAN_POINT('',(60.4402651077865,252.240326810636,20.4017818933262)) ;
#107623=CARTESIAN_POINT('Origin',(60.4402651077865,248.040265107786,23.0213203435596)) ;
#107624=CARTESIAN_POINT('',(60.4402651077865,251.829484664171,19.836306190763)) ;
#107625=CARTESIAN_POINT('Origin',(60.4402651077865,248.040265107786,23.0213203435596)) ;
#107626=CARTESIAN_POINT('',(60.4402651077865,251.225279260583,19.2321007871753)) ;
#107627=CARTESIAN_POINT('Origin',(60.4402651077865,248.040265107786,23.0213203435596)) ;
#107628=CARTESIAN_POINT('',(60.4402651077865,250.65980355802,18.8212586407095)) ;
#107629=CARTESIAN_POINT('Origin',(60.4402651077865,248.040265107786,23.0213203435596)) ;
#107630=CARTESIAN_POINT('',(60.4402651077865,249.898460333955,18.4333348922483)) ;
#107631=CARTESIAN_POINT('Origin',(60.4402651077865,248.040265107786,23.0213203435596)) ;
#107632=CARTESIAN_POINT('',(60.4402651077865,249.233703776962,18.2173423936815)) ;
#107633=CARTESIAN_POINT('Origin',(60.4402651077865,248.040265107786,23.0213203435596)) ;
#107634=CARTESIAN_POINT('',(60.4402651077865,248.389748311783,18.0836729796702)) ;
#107635=CARTESIAN_POINT('Origin',(60.4402651077865,248.040265107786,23.0213203435596)) ;
#107636=CARTESIAN_POINT('Origin',(60.4402651077865,248.040265107786,23.0213203435596)) ;
#107637=CARTESIAN_POINT('Origin',(60.4402651077865,248.040265107786,23.0213203435596)) ;
#107638=CARTESIAN_POINT('',(60.4402651077865,250.066361548099,17.9165880896072)) ;
#107639=CARTESIAN_POINT('',(60.4402651077865,249.21892856406,20.5247186334439)) ;
#107640=CARTESIAN_POINT('',(60.4402651077865,249.401604991106,17.700595591041)) ;
#107641=CARTESIAN_POINT('Origin',(60.4402651077865,249.739858576849,17.7905095039363)) ;
#107642=CARTESIAN_POINT('',(60.4402651077865,248.445501341285,20.6431800539285)) ;
#107643=CARTESIAN_POINT('Origin',(60.4402651077865,248.040265107786,23.0213203435596)) ;
#107644=CARTESIAN_POINT('',(60.4402651077865,251.544646348192,18.7925297017964)) ;
#107645=CARTESIAN_POINT('',(60.4402651077865,249.932733025005,21.0111380571975)) ;
#107646=CARTESIAN_POINT('',(60.4402651077865,250.979170645629,18.3816875553299)) ;
#107647=CARTESIAN_POINT('Origin',(60.4402651077865,251.273083995395,18.5717268744974)) ;
#107648=CARTESIAN_POINT('',(60.4402651077865,249.160553432798,20.8847994073294)) ;
#107649=CARTESIAN_POINT('Origin',(60.4402651077865,248.040265107786,23.0213203435596)) ;
#107650=CARTESIAN_POINT('',(60.4402651077865,252.679897896016,20.0824148057166)) ;
#107651=CARTESIAN_POINT('',(60.4402651077865,250.461289540614,21.6943281289039)) ;
#107652=CARTESIAN_POINT('',(60.4402651077865,252.26905574955,19.5169391031532)) ;
#107653=CARTESIAN_POINT('Origin',(60.4402651077865,252.489858576849,19.788501455951)) ;
#107654=CARTESIAN_POINT('',(60.4402651077865,249.765943897551,21.3355563159851)) ;
#107655=CARTESIAN_POINT('Origin',(60.4402651077865,248.040265107786,23.0213203435596)) ;
#107656=CARTESIAN_POINT('',(60.4402651077865,253.360989860306,21.6599804602399)) ;
#107657=CARTESIAN_POINT('',(60.4402651077865,250.752859316469,22.5074134442792)) ;
#107658=CARTESIAN_POINT('',(60.4402651077865,253.144997361738,20.9952239032473)) ;
#107659=CARTESIAN_POINT('Origin',(60.4402651077865,253.27107594741,21.3217268744974)) ;
#107660=CARTESIAN_POINT('',(60.4402651077865,250.202412898851,21.9513275530686)) ;
#107661=CARTESIAN_POINT('Origin',(60.4402651077865,248.040265107786,23.0213203435596)) ;
#107662=CARTESIAN_POINT('',(60.4402651077865,253.521252214148,23.3708035475559)) ;
#107663=CARTESIAN_POINT('',(60.4402651077865,250.778901471423,23.3708035475559)) ;
#107664=CARTESIAN_POINT('',(60.4402651077865,253.521252214148,22.6718371395634)) ;
#107665=CARTESIAN_POINT('Origin',(60.4402651077865,253.540265107786,23.0213203435596)) ;
#107666=CARTESIAN_POINT('',(60.4402651077865,250.427235809792,22.6718371395634)) ;
#107667=CARTESIAN_POINT('Origin',(60.4402651077865,248.040265107786,23.0213203435596)) ;
#107668=CARTESIAN_POINT('',(60.4402651077865,253.144997361739,25.0474167838721)) ;
#107669=CARTESIAN_POINT('',(60.4402651077865,250.536866817902,24.1999837998328)) ;
#107670=CARTESIAN_POINT('',(60.4402651077865,253.360989860305,24.3826602268791)) ;
#107671=CARTESIAN_POINT('Origin',(60.4402651077865,253.27107594741,24.7209138126218)) ;
#107672=CARTESIAN_POINT('',(60.4402651077865,250.418405397417,23.426556577058)) ;
#107673=CARTESIAN_POINT('Origin',(60.4402651077865,248.040265107786,23.0213203435596)) ;
#107674=CARTESIAN_POINT('',(60.4402651077865,252.26905574955,26.5257015839662)) ;
#107675=CARTESIAN_POINT('',(60.4402651077865,250.050447394148,24.9137882607786)) ;
#107676=CARTESIAN_POINT('',(60.4402651077865,252.679897896016,25.9602258814029)) ;
#107677=CARTESIAN_POINT('Origin',(60.4402651077865,252.489858576849,26.2541392311682)) ;
#107678=CARTESIAN_POINT('',(60.4402651077865,250.176786044017,24.1416086685709)) ;
#107679=CARTESIAN_POINT('Origin',(60.4402651077865,248.040265107786,23.0213203435596)) ;
#107680=CARTESIAN_POINT('',(60.4402651077865,250.979170645629,27.6609531317894)) ;
#107681=CARTESIAN_POINT('',(60.4402651077865,249.367257322442,25.4423447763876)) ;
#107682=CARTESIAN_POINT('',(60.4402651077865,251.544646348192,27.2501109853232)) ;
#107683=CARTESIAN_POINT('Origin',(60.4402651077865,251.273083995395,27.4709138126218)) ;
#107684=CARTESIAN_POINT('',(60.4402651077865,249.726029135361,24.746999133324)) ;
#107685=CARTESIAN_POINT('Origin',(60.4402651077865,248.040265107786,23.0213203435596)) ;
#107686=CARTESIAN_POINT('',(60.4402651077865,249.401604991106,28.3420450960785)) ;
#107687=CARTESIAN_POINT('',(60.4402651077865,248.554172007067,25.7339145522423)) ;
#107688=CARTESIAN_POINT('',(60.4402651077865,250.066361548098,28.1260525975113)) ;
#107689=CARTESIAN_POINT('Origin',(60.4402651077865,249.739858576849,28.252131183183)) ;
#107690=CARTESIAN_POINT('',(60.4402651077865,249.110257898277,25.1834681346239)) ;
#107691=CARTESIAN_POINT('Origin',(60.4402651077865,248.040265107786,23.0213203435596)) ;
#107692=CARTESIAN_POINT('',(60.4402651077865,247.69078190379,28.5023074499212)) ;
#107693=CARTESIAN_POINT('',(60.4402651077865,247.69078190379,25.759956707196)) ;
#107694=CARTESIAN_POINT('',(60.4402651077865,248.389748311783,28.5023074499214)) ;
#107695=CARTESIAN_POINT('Origin',(60.4402651077865,248.040265107786,28.5213203435596)) ;
#107696=CARTESIAN_POINT('',(60.4402651077865,248.389748311783,25.4082910455649)) ;
#107697=CARTESIAN_POINT('Origin',(60.4402651077865,248.040265107786,23.0213203435596)) ;
#107698=CARTESIAN_POINT('',(60.4402651077865,246.014168667474,28.1260525975118)) ;
#107699=CARTESIAN_POINT('',(60.4402651077865,246.861601651513,25.5179220536754)) ;
#107700=CARTESIAN_POINT('',(60.4402651077865,246.678925224467,28.3420450960783)) ;
#107701=CARTESIAN_POINT('Origin',(60.4402651077865,246.340671638724,28.252131183183)) ;
#107702=CARTESIAN_POINT('',(60.4402651077865,247.635028874288,25.3994606331908)) ;
#107703=CARTESIAN_POINT('Origin',(60.4402651077865,248.040265107786,23.0213203435596)) ;
#107704=CARTESIAN_POINT('',(60.4402651077865,244.53588386738,27.2501109853234)) ;
#107705=CARTESIAN_POINT('',(60.4402651077865,246.147797190567,25.0315026299217)) ;
#107706=CARTESIAN_POINT('',(60.4402651077865,245.101359569943,27.6609531317894)) ;
#107707=CARTESIAN_POINT('Origin',(60.4402651077865,244.807446220178,27.4709138126218)) ;
#107708=CARTESIAN_POINT('',(60.4402651077865,246.919976782775,25.1578412797899)) ;
#107709=CARTESIAN_POINT('Origin',(60.4402651077865,248.040265107786,23.0213203435596)) ;
#107710=CARTESIAN_POINT('',(60.4402651077865,243.400632319557,25.9602258814026)) ;
#107711=CARTESIAN_POINT('',(60.4402651077865,245.619240674958,24.3483125582154)) ;
#107712=CARTESIAN_POINT('',(60.4402651077865,243.811474466023,26.5257015839658)) ;
#107713=CARTESIAN_POINT('Origin',(60.4402651077865,243.590671638724,26.2541392311682)) ;
#107714=CARTESIAN_POINT('',(60.4402651077865,246.314586318022,24.7070843711341)) ;
#107715=CARTESIAN_POINT('Origin',(60.4402651077865,248.040265107786,23.0213203435596)) ;
#107716=CARTESIAN_POINT('',(60.4402651077865,242.719540355267,24.3826602268792)) ;
#107717=CARTESIAN_POINT('',(60.4402651077865,245.327670899104,23.5352272428401)) ;
#107718=CARTESIAN_POINT('',(60.4402651077865,242.935532853835,25.0474167838717)) ;
#107719=CARTESIAN_POINT('Origin',(60.4402651077865,242.809454268163,24.7209138126218)) ;
#107720=CARTESIAN_POINT('',(60.4402651077865,245.878117316722,24.0913131340507)) ;
#107721=CARTESIAN_POINT('Origin',(60.4402651077865,248.040265107786,23.0213203435596)) ;
#107722=CARTESIAN_POINT('',(60.4402651077865,242.559278001424,22.6718371395634)) ;
#107723=CARTESIAN_POINT('',(60.4402651077865,245.30162874415,22.6718371395634)) ;
#107724=CARTESIAN_POINT('',(60.4402651077865,242.559278001425,23.3708035475559)) ;
#107725=CARTESIAN_POINT('Origin',(60.4402651077865,242.540265107786,23.0213203435596)) ;
#107726=CARTESIAN_POINT('',(60.4402651077865,245.653294405781,23.3708035475559)) ;
#107727=CARTESIAN_POINT('Origin',(60.4402651077865,248.040265107786,23.0213203435596)) ;
#107728=CARTESIAN_POINT('',(60.4402651077865,242.935532853834,20.9952239032473)) ;
#107729=CARTESIAN_POINT('',(60.4402651077865,245.543663397671,21.8426568872864)) ;
#107730=CARTESIAN_POINT('',(60.4402651077865,242.719540355268,21.6599804602402)) ;
#107731=CARTESIAN_POINT('Origin',(60.4402651077865,242.809454268163,21.3217268744974)) ;
#107732=CARTESIAN_POINT('',(60.4402651077865,245.662124818155,22.6160841100613)) ;
#107733=CARTESIAN_POINT('Origin',(60.4402651077865,248.040265107786,23.0213203435596)) ;
#107734=CARTESIAN_POINT('',(60.4402651077865,243.811474466023,19.5169391031534)) ;
#107735=CARTESIAN_POINT('',(60.4402651077865,246.030082821424,21.1288524263407)) ;
#107736=CARTESIAN_POINT('',(60.4402651077865,243.400632319557,20.0824148057165)) ;
#107737=CARTESIAN_POINT('Origin',(60.4402651077865,243.590671638724,19.788501455951)) ;
#107738=CARTESIAN_POINT('',(60.4402651077865,245.903744171556,21.9010320185483)) ;
#107739=CARTESIAN_POINT('Origin',(60.4402651077865,248.040265107786,23.0213203435596)) ;
#107740=CARTESIAN_POINT('',(60.4402651077865,245.101359569943,18.3816875553301)) ;
#107741=CARTESIAN_POINT('',(60.4402651077865,246.713272893131,20.6002959107317)) ;
#107742=CARTESIAN_POINT('',(60.4402651077865,244.53588386738,18.7925297017959)) ;
#107743=CARTESIAN_POINT('Origin',(60.4402651077865,244.807446220178,18.5717268744974)) ;
#107744=CARTESIAN_POINT('',(60.4402651077865,246.354501080212,21.2956415537952)) ;
#107745=CARTESIAN_POINT('Origin',(60.4402651077865,248.040265107786,23.0213203435596)) ;
#107746=CARTESIAN_POINT('',(60.4402651077865,246.678925224467,17.7005955910407)) ;
#107747=CARTESIAN_POINT('',(60.4402651077865,247.526358208506,20.3087261348769)) ;
#107748=CARTESIAN_POINT('',(60.4402651077865,246.014168667474,17.9165880896081)) ;
#107749=CARTESIAN_POINT('Origin',(60.4402651077865,246.340671638724,17.7905095039363)) ;
#107750=CARTESIAN_POINT('',(60.4402651077865,246.970272317295,20.8591725524954)) ;
#107751=CARTESIAN_POINT('Origin',(60.4402651077865,248.040265107786,23.0213203435596)) ;
#107752=CARTESIAN_POINT('',(60.4402651077865,248.389748311783,17.5403332371977)) ;
#107753=CARTESIAN_POINT('',(60.4402651077865,248.389748311783,20.2826839799233)) ;
#107754=CARTESIAN_POINT('',(60.4402651077865,247.69078190379,17.5403332371979)) ;
#107755=CARTESIAN_POINT('Origin',(60.4402651077865,248.040265107786,17.5213203435596)) ;
#107756=CARTESIAN_POINT('',(60.4402651077865,247.69078190379,20.6343496415544)) ;
#107757=CARTESIAN_POINT('Origin',(60.5902651077865,248.040265107786,23.0213203435596)) ;
#107758=CARTESIAN_POINT('',(60.5902651077865,246.946891701628,28.0027392774284)) ;
#107759=CARTESIAN_POINT('Ctrl Pts',(60.4402651077865,246.84682643861,27.8252982934377)) ;
#107760=CARTESIAN_POINT('Ctrl Pts',(60.4402651077865,246.847209116359,27.8259879723372)) ;
#107761=CARTESIAN_POINT('Ctrl Pts',(60.440268437892,246.847591853016,27.8266776249678)) ;
#107762=CARTESIAN_POINT('Ctrl Pts',(60.4404467789389,246.857838938126,27.8451382901616)) ;
#107763=CARTESIAN_POINT('Ctrl Pts',(60.4428319502748,246.86777865457,27.8629553332033)) ;
#107764=CARTESIAN_POINT('Ctrl Pts',(60.4520052987552,246.88669215874,27.8966993889314)) ;
#107765=CARTESIAN_POINT('Ctrl Pts',(60.4586423249847,246.895772989479,27.9128241441561)) ;
#107766=CARTESIAN_POINT('Ctrl Pts',(60.4774783235664,246.913652858034,27.9444499271496)) ;
#107767=CARTESIAN_POINT('Ctrl Pts',(60.4902886559451,246.92239313214,27.9598318195758)) ;
#107768=CARTESIAN_POINT('Ctrl Pts',(60.5183067650572,246.935114921148,27.9821554300886)) ;
#107769=CARTESIAN_POINT('Ctrl Pts',(60.5322233323112,246.939674844702,27.9901316702287)) ;
#107770=CARTESIAN_POINT('Ctrl Pts',(60.5612197979218,246.945446722844,28.0002186669547)) ;
#107771=CARTESIAN_POINT('Ctrl Pts',(60.5755858845328,246.946891701628,28.0027392774284)) ;
#107772=CARTESIAN_POINT('Ctrl Pts',(60.5902651077866,246.946891701628,28.0027392774284)) ;
#107773=CARTESIAN_POINT('',(60.5902651077865,247.54078190379,28.096802244712)) ;
#107774=CARTESIAN_POINT('Origin',(60.5902651077865,248.040265107786,23.0213203435596)) ;
#107775=CARTESIAN_POINT('Ctrl Pts',(60.4402651077865,247.69078190379,27.9589677074491)) ;
#107776=CARTESIAN_POINT('Ctrl Pts',(60.4402651077865,247.690204833126,27.9595053771295)) ;
#107777=CARTESIAN_POINT('Ctrl Pts',(60.440268437892,247.68962771455,27.9600430036272)) ;
#107778=CARTESIAN_POINT('Ctrl Pts',(60.4404467789383,247.674177498214,27.9744336161106)) ;
#107779=CARTESIAN_POINT('Ctrl Pts',(60.4428319502738,247.659218497029,27.9883070896971)) ;
#107780=CARTESIAN_POINT('Ctrl Pts',(60.4520052987543,247.630803198961,28.0145549995742)) ;
#107781=CARTESIAN_POINT('Ctrl Pts',(60.4586423249841,247.617183992317,28.0270844220836)) ;
#107782=CARTESIAN_POINT('Ctrl Pts',(60.4774783235664,247.590406322412,28.0516371458428)) ;
#107783=CARTESIAN_POINT('Ctrl Pts',(60.4902886559451,247.577340561604,28.0635653016335)) ;
#107784=CARTESIAN_POINT('Ctrl Pts',(60.5183067650572,247.558343046244,28.0808650678764)) ;
#107785=CARTESIAN_POINT('Ctrl Pts',(60.5322233323112,247.55154150748,28.087041829166)) ;
#107786=CARTESIAN_POINT('Ctrl Pts',(60.5612197979217,247.542935071751,28.0948515246967)) ;
#107787=CARTESIAN_POINT('Ctrl Pts',(60.5755858845327,247.54078190379,28.096802244712)) ;
#107788=CARTESIAN_POINT('Ctrl Pts',(60.5902651077865,247.54078190379,28.096802244712)) ;
#107789=CARTESIAN_POINT('Origin',(60.5902651077865,247.635028874288,25.3994606331908)) ;
#107790=CARTESIAN_POINT('',(60.5902651077865,246.822731508173,28.3848650607978)) ;
#107791=CARTESIAN_POINT('Ctrl Pts',(60.4402651077865,246.678925224467,28.3420450960783)) ;
#107792=CARTESIAN_POINT('Ctrl Pts',(60.4402651077865,246.680324229639,28.3424579870217)) ;
#107793=CARTESIAN_POINT('Ctrl Pts',(60.440286369022,246.681723125547,28.3428709748965)) ;
#107794=CARTESIAN_POINT('Ctrl Pts',(60.4403288850239,246.683121466859,28.343283925702)) ;
#107795=CARTESIAN_POINT('Ctrl Pts',(60.4408750760621,246.701085561798,28.3485889877858)) ;
#107796=CARTESIAN_POINT('Ctrl Pts',(60.4449239452533,246.718788094142,28.3538380651872)) ;
#107797=CARTESIAN_POINT('Ctrl Pts',(60.4522665395981,246.735313540781,28.3587517471949)) ;
#107798=CARTESIAN_POINT('Ctrl Pts',(60.4599211853139,246.752541298897,28.3638742547396)) ;
#107799=CARTESIAN_POINT('Ctrl Pts',(60.4710122117666,246.768167444445,28.3685360408185)) ;
#107800=CARTESIAN_POINT('Ctrl Pts',(60.4849165768426,246.781315020339,28.3724647819378)) ;
#107801=CARTESIAN_POINT('Ctrl Pts',(60.4988172216939,246.794459078493,28.3763924718908)) ;
#107802=CARTESIAN_POINT('Ctrl Pts',(60.5152637963995,246.804874499694,28.3795121161121)) ;
#107803=CARTESIAN_POINT('Ctrl Pts',(60.5333315664699,246.811976821569,28.3816405503696)) ;
#107804=CARTESIAN_POINT('Ctrl Pts',(60.5513971100607,246.81907826823,28.3837687223414)) ;
#107805=CARTESIAN_POINT('Ctrl Pts',(60.5707376338846,246.822731508174,28.3848650607972)) ;
#107806=CARTESIAN_POINT('Ctrl Pts',(60.5902651077865,246.822731508174,28.3848650607972)) ;
#107807=CARTESIAN_POINT('',(60.5902651077865,247.777687351732,25.445813182347)) ;
#107808=CARTESIAN_POINT('Origin',(60.5902651077865,247.69078190379,25.759956707196)) ;
#107809=CARTESIAN_POINT('',(60.5902651077865,247.54078190379,28.4985930708324)) ;
#107810=CARTESIAN_POINT('',(60.5902651077865,247.54078190379,25.759956707196)) ;
#107811=CARTESIAN_POINT('Ctrl Pts',(60.5902651077865,247.54078190379,28.4985930708324)) ;
#107812=CARTESIAN_POINT('Ctrl Pts',(60.5707376338847,247.54078190379,28.4985930708324)) ;
#107813=CARTESIAN_POINT('Ctrl Pts',(60.5513971100608,247.544595128658,28.4986793042264)) ;
#107814=CARTESIAN_POINT('Ctrl Pts',(60.5333315664699,247.552006647086,28.4988497601077)) ;
#107815=CARTESIAN_POINT('Ctrl Pts',(60.5152637963994,247.559419078944,28.4990202369967)) ;
#107816=CARTESIAN_POINT('Ctrl Pts',(60.4988172216937,247.570288756228,28.4992718211856)) ;
#107817=CARTESIAN_POINT('Ctrl Pts',(60.4849165768426,247.58400322133,28.4995981034065)) ;
#107818=CARTESIAN_POINT('Ctrl Pts',(60.4710122117669,247.597721356829,28.4999244729501)) ;
#107819=CARTESIAN_POINT('Ctrl Pts',(60.4599211853139,247.6140232755,28.5003195954534)) ;
#107820=CARTESIAN_POINT('Ctrl Pts',(60.452266539598,247.631990789003,28.5007714713061)) ;
#107821=CARTESIAN_POINT('Ctrl Pts',(60.4449239452531,247.649225833959,28.5012049258647)) ;
#107822=CARTESIAN_POINT('Ctrl Pts',(60.4408750760621,247.667683996822,28.5016831399335)) ;
#107823=CARTESIAN_POINT('Ctrl Pts',(60.4403288850239,247.686408220711,28.5021889366962)) ;
#107824=CARTESIAN_POINT('Ctrl Pts',(60.440286369022,247.687865731145,28.5022283083713)) ;
#107825=CARTESIAN_POINT('Ctrl Pts',(60.4402651077865,247.689323780486,28.50226781617)) ;
#107826=CARTESIAN_POINT('Ctrl Pts',(60.4402651077865,247.69078190379,28.5023074499212)) ;
#107827=CARTESIAN_POINT('Origin',(60.5902651077865,246.861601651513,25.5179220536754)) ;
#107828=CARTESIAN_POINT('Ctrl Pts',(60.4402651077865,246.182069881617,27.6093057948708)) ;
#107829=CARTESIAN_POINT('Ctrl Pts',(60.4402651077865,246.181354905733,27.6096388244826)) ;
#107830=CARTESIAN_POINT('Ctrl Pts',(60.4402684378921,246.180639897624,27.6099717982194)) ;
#107831=CARTESIAN_POINT('Ctrl Pts',(60.4404467789386,246.161498924882,27.6188837045809)) ;
#107832=CARTESIAN_POINT('Ctrl Pts',(60.4428319502743,246.142984930219,27.6274555764537)) ;
#107833=CARTESIAN_POINT('Ctrl Pts',(60.4520052987548,246.107849325612,27.6436380121775)) ;
#107834=CARTESIAN_POINT('Ctrl Pts',(60.4586423249844,246.091024885902,27.6513456347974)) ;
#107835=CARTESIAN_POINT('Ctrl Pts',(60.4774783235664,246.057970599548,27.6664219076506)) ;
#107836=CARTESIAN_POINT('Ctrl Pts',(60.4902886559451,246.04185831974,27.6737287158086)) ;
#107837=CARTESIAN_POINT('Ctrl Pts',(60.5183067650571,246.018444687196,27.6843112161272)) ;
#107838=CARTESIAN_POINT('Ctrl Pts',(60.5322233323112,246.010067315225,27.6880838741351)) ;
#107839=CARTESIAN_POINT('Ctrl Pts',(60.5612197979218,245.999468779803,27.6928518010587)) ;
#107840=CARTESIAN_POINT('Ctrl Pts',(60.5755858845328,245.996818189747,27.694041680549)) ;
#107841=CARTESIAN_POINT('Ctrl Pts',(60.5902651077865,245.996818189747,27.694041680549)) ;
#107842=CARTESIAN_POINT('',(60.5902651077865,245.872657996292,28.0761674639184)) ;
#107843=CARTESIAN_POINT('',(60.5902651077865,246.718943174069,25.4715695045192)) ;
#107844=CARTESIAN_POINT('Ctrl Pts',(60.5902651077865,245.872657996292,28.0761674639184)) ;
#107845=CARTESIAN_POINT('Ctrl Pts',(60.5707376338847,245.872657996292,28.0761674639184)) ;
#107846=CARTESIAN_POINT('Ctrl Pts',(60.5513971100606,245.876257941067,28.0774278280374)) ;
#107847=CARTESIAN_POINT('Ctrl Pts',(60.5333315664698,245.883254040199,28.0798802263625)) ;
#107848=CARTESIAN_POINT('Ctrl Pts',(60.5152637963995,245.890251001563,28.0823329269323)) ;
#107849=CARTESIAN_POINT('Ctrl Pts',(60.4988172216939,245.900510935184,28.0859311127188)) ;
#107850=CARTESIAN_POINT('Ctrl Pts',(60.4849165768426,245.913453339835,28.0904794283364)) ;
#107851=CARTESIAN_POINT('Ctrl Pts',(60.4710122117669,245.926399208258,28.0950289612181)) ;
#107852=CARTESIAN_POINT('Ctrl Pts',(60.4599211853139,245.94178115467,28.1004423149597)) ;
#107853=CARTESIAN_POINT('Ctrl Pts',(60.452266539598,245.958729638151,28.1064243414529)) ;
#107854=CARTESIAN_POINT('Ctrl Pts',(60.4449239452531,245.97498719514,28.1121625030258)) ;
#107855=CARTESIAN_POINT('Ctrl Pts',(60.4408750760621,245.992394174936,28.1183211976404)) ;
#107856=CARTESIAN_POINT('Ctrl Pts',(60.4403288850239,246.010045670283,28.1245883423369)) ;
#107857=CARTESIAN_POINT('Ctrl Pts',(60.440286369022,246.011419678562,28.1250761825186)) ;
#107858=CARTESIAN_POINT('Ctrl Pts',(60.4402651077865,246.012794157307,28.1255643186937)) ;
#107859=CARTESIAN_POINT('Ctrl Pts',(60.4402651077865,246.014168667474,28.1260525975118)) ;
#107860=CARTESIAN_POINT('Origin',(60.5902651077865,248.040265107786,23.0213203435596)) ;
#107861=CARTESIAN_POINT('Ctrl Pts',(60.4402651077865,245.420726657552,27.2213820464094)) ;
#107862=CARTESIAN_POINT('Ctrl Pts',(60.4402651077865,245.420877483217,27.2221562239435)) ;
#107863=CARTESIAN_POINT('Ctrl Pts',(60.440268437892,245.421028373027,27.2229303947057)) ;
#107864=CARTESIAN_POINT('Ctrl Pts',(60.4404467789383,245.425069270821,27.2436540540717)) ;
#107865=CARTESIAN_POINT('Ctrl Pts',(60.4428319502739,245.429016733826,27.2636706102593)) ;
#107866=CARTESIAN_POINT('Ctrl Pts',(60.4520052987543,245.436577058534,27.3016077085599)) ;
#107867=CARTESIAN_POINT('Ctrl Pts',(60.4586423249841,245.440230618388,27.3197493931132)) ;
#107868=CARTESIAN_POINT('Ctrl Pts',(60.4774783235665,245.447462479482,27.3553524833539)) ;
#107869=CARTESIAN_POINT('Ctrl Pts',(60.4902886559452,245.451021707959,27.3726824256129)) ;
#107870=CARTESIAN_POINT('Ctrl Pts',(60.5183067650571,245.45622247327,27.3978446898607)) ;
#107871=CARTESIAN_POINT('Ctrl Pts',(60.5322233323112,245.458094424526,27.4068396388929)) ;
#107872=CARTESIAN_POINT('Ctrl Pts',(60.5612197979217,245.460466753434,27.4182165512943)) ;
#107873=CARTESIAN_POINT('Ctrl Pts',(60.5755858845327,245.461062098449,27.4210603173112)) ;
#107874=CARTESIAN_POINT('Ctrl Pts',(60.5902651077865,245.461062098449,27.4210603173112)) ;
#107875=CARTESIAN_POINT('Origin',(60.5902651077865,246.919976782775,25.1578412797899)) ;
#107876=CARTESIAN_POINT('Ctrl Pts',(60.4402651077865,245.101359569943,27.6609531317894)) ;
#107877=CARTESIAN_POINT('Ctrl Pts',(60.4402651077865,245.102562512611,27.6617781307852)) ;
#107878=CARTESIAN_POINT('Ctrl Pts',(60.440286369022,245.103765321408,27.6626031882028)) ;
#107879=CARTESIAN_POINT('Ctrl Pts',(60.4403288850239,245.104967614208,27.6634280389871)) ;
#107880=CARTESIAN_POINT('Ctrl Pts',(60.4408750760621,245.120413129416,27.6740246634793)) ;
#107881=CARTESIAN_POINT('Ctrl Pts',(60.4449239452533,245.135627184036,27.6844872160823)) ;
#107882=CARTESIAN_POINT('Ctrl Pts',(60.4522665395981,245.149825406502,27.6942670492256)) ;
#107883=CARTESIAN_POINT('Ctrl Pts',(60.4599211853139,245.164627036234,27.7044625134384)) ;
#107884=CARTESIAN_POINT('Ctrl Pts',(60.4710122117667,245.17804781266,27.7137248799967)) ;
#107885=CARTESIAN_POINT('Ctrl Pts',(60.4849165768426,245.189337852615,27.7215241592249)) ;
#107886=CARTESIAN_POINT('Ctrl Pts',(60.4988172216939,245.200624871829,27.7293213516934)) ;
#107887=CARTESIAN_POINT('Ctrl Pts',(60.5152637963994,245.209566502951,27.7355068518133)) ;
#107888=CARTESIAN_POINT('Ctrl Pts',(60.5333315664698,245.215663490095,27.7397258512423)) ;
#107889=CARTESIAN_POINT('Ctrl Pts',(60.5513971100606,245.22175972591,27.7439443307667)) ;
#107890=CARTESIAN_POINT('Ctrl Pts',(60.5707376338847,245.224895376349,27.7461159238267)) ;
#107891=CARTESIAN_POINT('Ctrl Pts',(60.5902651077865,245.22489537635,27.7461159238262)) ;
#107892=CARTESIAN_POINT('Origin',(60.5902651077865,248.554172007067,25.7339145522423)) ;
#107893=CARTESIAN_POINT('',(60.5902651077865,249.133638513944,28.0027392774284)) ;
#107894=CARTESIAN_POINT('',(60.5902651077865,249.257798707399,28.3848650607978)) ;
#107895=CARTESIAN_POINT('',(60.5902651077865,248.411513529623,25.7802671013986)) ;
#107896=CARTESIAN_POINT('Ctrl Pts',(60.5902651077865,249.257798707399,28.3848650607969)) ;
#107897=CARTESIAN_POINT('Ctrl Pts',(60.5707376338847,249.257798707399,28.3848650607969)) ;
#107898=CARTESIAN_POINT('Ctrl Pts',(60.5513971100606,249.261451947343,28.3837687223414)) ;
#107899=CARTESIAN_POINT('Ctrl Pts',(60.5333315664698,249.268553394004,28.3816405503695)) ;
#107900=CARTESIAN_POINT('Ctrl Pts',(60.5152637963994,249.275655715879,28.379512116112)) ;
#107901=CARTESIAN_POINT('Ctrl Pts',(60.4988172216938,249.28607113708,28.3763924718905)) ;
#107902=CARTESIAN_POINT('Ctrl Pts',(60.4849165768427,249.299215195234,28.3724647819375)) ;
#107903=CARTESIAN_POINT('Ctrl Pts',(60.471012211767,249.312362771127,28.3685360408181)) ;
#107904=CARTESIAN_POINT('Ctrl Pts',(60.4599211853138,249.327988916676,28.3638742547393)) ;
#107905=CARTESIAN_POINT('Ctrl Pts',(60.452266539598,249.345216674792,28.3587517471944)) ;
#107906=CARTESIAN_POINT('Ctrl Pts',(60.4449239452532,249.361742121431,28.3538380651865)) ;
#107907=CARTESIAN_POINT('Ctrl Pts',(60.4408750760622,249.379444653775,28.3485889877863)) ;
#107908=CARTESIAN_POINT('Ctrl Pts',(60.4403288850239,249.397408748713,28.3432839257019)) ;
#107909=CARTESIAN_POINT('Ctrl Pts',(60.440286369022,249.398807090025,28.3428709748963)) ;
#107910=CARTESIAN_POINT('Ctrl Pts',(60.4402651077865,249.400205985933,28.342457987022)) ;
#107911=CARTESIAN_POINT('Ctrl Pts',(60.4402651077865,249.401604991106,28.3420450960785)) ;
#107912=CARTESIAN_POINT('Ctrl Pts',(60.4402651077865,249.233703776962,27.8252982934377)) ;
#107913=CARTESIAN_POINT('Ctrl Pts',(60.4402651077865,249.233321099215,27.8259879723341)) ;
#107914=CARTESIAN_POINT('Ctrl Pts',(60.4402684378921,249.232938362557,27.8266776249672)) ;
#107915=CARTESIAN_POINT('Ctrl Pts',(60.4404467789386,249.222691277448,27.8451382901584)) ;
#107916=CARTESIAN_POINT('Ctrl Pts',(60.4428319502743,249.212751561004,27.8629553332008)) ;
#107917=CARTESIAN_POINT('Ctrl Pts',(60.4520052987547,249.193838056834,27.8966993889301)) ;
#107918=CARTESIAN_POINT('Ctrl Pts',(60.4586423249844,249.184757226094,27.9128241441556)) ;
#107919=CARTESIAN_POINT('Ctrl Pts',(60.4774783235664,249.166877357539,27.9444499271496)) ;
#107920=CARTESIAN_POINT('Ctrl Pts',(60.4902886559451,249.158137083433,27.9598318195758)) ;
#107921=CARTESIAN_POINT('Ctrl Pts',(60.5183067650572,249.145415294424,27.9821554300886)) ;
#107922=CARTESIAN_POINT('Ctrl Pts',(60.5322233323113,249.14085537087,27.9901316702288)) ;
#107923=CARTESIAN_POINT('Ctrl Pts',(60.5612197979218,249.135083492728,28.0002186669547)) ;
#107924=CARTESIAN_POINT('Ctrl Pts',(60.5755858845327,249.133638513944,28.0027392774284)) ;
#107925=CARTESIAN_POINT('Ctrl Pts',(60.5902651077865,249.133638513944,28.0027392774284)) ;
#107926=CARTESIAN_POINT('Origin',(60.5902651077865,246.147797190567,25.0315026299217)) ;
#107927=CARTESIAN_POINT('Ctrl Pts',(60.4402651077865,244.85525095499,26.8105398999439)) ;
#107928=CARTESIAN_POINT('Ctrl Pts',(60.4402651077865,244.854468060706,26.8106356902274)) ;
#107929=CARTESIAN_POINT('Ctrl Pts',(60.4402684378921,244.853685153042,26.8107314174129)) ;
#107930=CARTESIAN_POINT('Ctrl Pts',(60.4404467789386,244.832727075669,26.8132922581644)) ;
#107931=CARTESIAN_POINT('Ctrl Pts',(60.4428319502743,244.81247036632,26.8157234537812)) ;
#107932=CARTESIAN_POINT('Ctrl Pts',(60.4520052987548,244.774053772956,26.8202563657947)) ;
#107933=CARTESIAN_POINT('Ctrl Pts',(60.4586423249844,244.75567099356,26.8223877127213)) ;
#107934=CARTESIAN_POINT('Ctrl Pts',(60.4774783235664,244.719575674609,26.8265117640394)) ;
#107935=CARTESIAN_POINT('Ctrl Pts',(60.4902886559451,244.70199405801,26.8284819832727)) ;
#107936=CARTESIAN_POINT('Ctrl Pts',(60.5183067650572,244.676456197767,26.8313113288033)) ;
#107937=CARTESIAN_POINT('Ctrl Pts',(60.5322233323112,244.667323028126,26.832310589478)) ;
#107938=CARTESIAN_POINT('Ctrl Pts',(60.5612197979217,244.655769851502,26.8335700298872)) ;
#107939=CARTESIAN_POINT('Ctrl Pts',(60.5755858845327,244.652881297574,26.8338825951576)) ;
#107940=CARTESIAN_POINT('Ctrl Pts',(60.5902651077865,244.652881297574,26.8338825951576)) ;
#107941=CARTESIAN_POINT('Ctrl Pts',(60.5902651077865,244.416714575474,27.1589382016726)) ;
#107942=CARTESIAN_POINT('Ctrl Pts',(60.5707376338846,244.416714575474,27.1589382016726)) ;
#107943=CARTESIAN_POINT('Ctrl Pts',(60.5513971100607,244.419748852478,27.1612493232954)) ;
#107944=CARTESIAN_POINT('Ctrl Pts',(60.5333315664697,244.425644705387,27.1657436062293)) ;
#107945=CARTESIAN_POINT('Ctrl Pts',(60.5152637963991,244.431541284929,27.1702384430589)) ;
#107946=CARTESIAN_POINT('Ctrl Pts',(60.4988172216935,244.440187161099,27.1768310149478)) ;
#107947=CARTESIAN_POINT('Ctrl Pts',(60.4849165768424,244.451090612557,27.1851561431397)) ;
#107948=CARTESIAN_POINT('Ctrl Pts',(60.4710122117667,244.461996982103,27.1934834993826)) ;
#107949=CARTESIAN_POINT('Ctrl Pts',(60.4599211853136,244.474953264169,27.2033851875814)) ;
#107950=CARTESIAN_POINT('Ctrl Pts',(60.4522665395979,244.489223681977,27.2143118022826)) ;
#107951=CARTESIAN_POINT('Ctrl Pts',(60.4449239452532,244.502912348048,27.2247929796344)) ;
#107952=CARTESIAN_POINT('Ctrl Pts',(60.4408750760621,244.51756422831,27.2360292988605)) ;
#107953=CARTESIAN_POINT('Ctrl Pts',(60.4403288850239,244.532415143768,27.2474443196983)) ;
#107954=CARTESIAN_POINT('Ctrl Pts',(60.440286369022,244.533571152388,27.2483328751903)) ;
#107955=CARTESIAN_POINT('Ctrl Pts',(60.4402651077865,244.534727516982,27.249221857571)) ;
#107956=CARTESIAN_POINT('Ctrl Pts',(60.4402651077865,244.53588386738,27.2501109853234)) ;
#107957=CARTESIAN_POINT('Origin',(60.5902651077865,248.040265107786,23.0213203435596)) ;
#107958=CARTESIAN_POINT('Ctrl Pts',(60.4402651077865,244.251045551402,26.2063344963562)) ;
#107959=CARTESIAN_POINT('Ctrl Pts',(60.4402651077865,244.250949761119,26.2071173906402)) ;
#107960=CARTESIAN_POINT('Ctrl Pts',(60.4402684378921,244.250854033933,26.2079002983041)) ;
#107961=CARTESIAN_POINT('Ctrl Pts',(60.4404467789386,244.248293193181,26.228858375676)) ;
#107962=CARTESIAN_POINT('Ctrl Pts',(60.4428319502743,244.245861997565,26.2491150850256)) ;
#107963=CARTESIAN_POINT('Ctrl Pts',(60.4520052987547,244.241329085551,26.2875316783901)) ;
#107964=CARTESIAN_POINT('Ctrl Pts',(60.4586423249843,244.239197738625,26.3059144577853)) ;
#107965=CARTESIAN_POINT('Ctrl Pts',(60.4774783235665,244.235073687307,26.3420097767375)) ;
#107966=CARTESIAN_POINT('Ctrl Pts',(60.4902886559452,244.233103468073,26.3595913933363)) ;
#107967=CARTESIAN_POINT('Ctrl Pts',(60.5183067650571,244.230274122543,26.3851292535788)) ;
#107968=CARTESIAN_POINT('Ctrl Pts',(60.5322233323112,244.229274861868,26.3942624232202)) ;
#107969=CARTESIAN_POINT('Ctrl Pts',(60.5612197979218,244.228015421459,26.4058155998437)) ;
#107970=CARTESIAN_POINT('Ctrl Pts',(60.5755858845328,244.227702856188,26.4087041537722)) ;
#107971=CARTESIAN_POINT('Ctrl Pts',(60.5902651077865,244.227702856188,26.4087041537722)) ;
#107972=CARTESIAN_POINT('Origin',(60.5902651077865,246.314586318022,24.7070843711341)) ;
#107973=CARTESIAN_POINT('Ctrl Pts',(60.4402651077865,243.811474466023,26.5257015839658)) ;
#107974=CARTESIAN_POINT('Ctrl Pts',(60.4402651077865,243.812363593775,26.5268579343639)) ;
#107975=CARTESIAN_POINT('Ctrl Pts',(60.440286369022,243.813252576155,26.5280142989582)) ;
#107976=CARTESIAN_POINT('Ctrl Pts',(60.4403288850239,243.814141131647,26.5291703075783)) ;
#107977=CARTESIAN_POINT('Ctrl Pts',(60.4408750760621,243.82555615249,26.5440212230314)) ;
#107978=CARTESIAN_POINT('Ctrl Pts',(60.4449239452531,243.83679247171,26.5586731032986)) ;
#107979=CARTESIAN_POINT('Ctrl Pts',(60.452266539598,243.847273649062,26.5723617693696)) ;
#107980=CARTESIAN_POINT('Ctrl Pts',(60.4599211853137,243.858200263764,26.5866321871774)) ;
#107981=CARTESIAN_POINT('Ctrl Pts',(60.4710122117667,243.868101951963,26.599588469243)) ;
#107982=CARTESIAN_POINT('Ctrl Pts',(60.4849165768426,243.876429308206,26.6104948387886)) ;
#107983=CARTESIAN_POINT('Ctrl Pts',(60.498817221694,243.884754436398,26.6213982902475)) ;
#107984=CARTESIAN_POINT('Ctrl Pts',(60.5152637963994,243.891347008287,26.6300441664173)) ;
#107985=CARTESIAN_POINT('Ctrl Pts',(60.5333315664698,243.895841845116,26.6359407459585)) ;
#107986=CARTESIAN_POINT('Ctrl Pts',(60.5513971100606,243.90033612805,26.6418365988681)) ;
#107987=CARTESIAN_POINT('Ctrl Pts',(60.5707376338848,243.902647249673,26.6448708758722)) ;
#107988=CARTESIAN_POINT('Ctrl Pts',(60.5902651077865,243.902647249673,26.6448708758723)) ;
#107989=CARTESIAN_POINT('Origin',(60.5902651077865,249.367257322442,25.4423447763876)) ;
#107990=CARTESIAN_POINT('',(60.5902651077865,250.619468117123,27.4210603173112)) ;
#107991=CARTESIAN_POINT('',(60.5902651077865,250.855634839223,27.7461159238265)) ;
#107992=CARTESIAN_POINT('',(60.5902651077865,249.245904773286,25.5305125642315)) ;
#107993=CARTESIAN_POINT('Ctrl Pts',(60.5902651077865,250.855634839223,27.7461159238265)) ;
#107994=CARTESIAN_POINT('Ctrl Pts',(60.5707376338848,250.855634839223,27.7461159238265)) ;
#107995=CARTESIAN_POINT('Ctrl Pts',(60.5513971100609,250.858770489662,27.7439443307668)) ;
#107996=CARTESIAN_POINT('Ctrl Pts',(60.5333315664698,250.864866725478,27.7397258512425)) ;
#107997=CARTESIAN_POINT('Ctrl Pts',(60.5152637963993,250.870963712622,27.7355068518136)) ;
#107998=CARTESIAN_POINT('Ctrl Pts',(60.4988172216938,250.879905343744,27.7293213516936)) ;
#107999=CARTESIAN_POINT('Ctrl Pts',(60.4849165768427,250.891192362958,27.7215241592251)) ;
#108000=CARTESIAN_POINT('Ctrl Pts',(60.471012211767,250.902482402912,27.7137248799968)) ;
#108001=CARTESIAN_POINT('Ctrl Pts',(60.4599211853139,250.915903179339,27.7044625134388)) ;
#108002=CARTESIAN_POINT('Ctrl Pts',(60.4522665395981,250.930704809072,27.6942670492262)) ;
#108003=CARTESIAN_POINT('Ctrl Pts',(60.4449239452533,250.944903031537,27.6844872160832)) ;
#108004=CARTESIAN_POINT('Ctrl Pts',(60.4408750760621,250.960117086155,27.674024663477)) ;
#108005=CARTESIAN_POINT('Ctrl Pts',(60.4403288850239,250.975562601365,27.6634280389875)) ;
#108006=CARTESIAN_POINT('Ctrl Pts',(60.440286369022,250.976764894165,27.6626031882035)) ;
#108007=CARTESIAN_POINT('Ctrl Pts',(60.4402651077865,250.977967702962,27.6617781307852)) ;
#108008=CARTESIAN_POINT('Ctrl Pts',(60.4402651077865,250.979170645629,27.6609531317894)) ;
#108009=CARTESIAN_POINT('Ctrl Pts',(60.4402651077865,250.65980355802,27.2213820464098)) ;
#108010=CARTESIAN_POINT('Ctrl Pts',(60.4402651077865,250.659652732355,27.2221562239442)) ;
#108011=CARTESIAN_POINT('Ctrl Pts',(60.440268437892,250.659501842545,27.2229303947054)) ;
#108012=CARTESIAN_POINT('Ctrl Pts',(60.4404467789383,250.655460944752,27.2436540540713)) ;
#108013=CARTESIAN_POINT('Ctrl Pts',(60.4428319502738,250.651513481747,27.2636706102592)) ;
#108014=CARTESIAN_POINT('Ctrl Pts',(60.4520052987543,250.643953157039,27.3016077085601)) ;
#108015=CARTESIAN_POINT('Ctrl Pts',(60.4586423249841,250.640299597185,27.3197493931132)) ;
#108016=CARTESIAN_POINT('Ctrl Pts',(60.4774783235664,250.633067736091,27.3553524833537)) ;
#108017=CARTESIAN_POINT('Ctrl Pts',(60.4902886559451,250.629508507613,27.3726824256129)) ;
#108018=CARTESIAN_POINT('Ctrl Pts',(60.5183067650571,250.624307742302,27.3978446898607)) ;
#108019=CARTESIAN_POINT('Ctrl Pts',(60.5322233323112,250.622435791047,27.4068396388929)) ;
#108020=CARTESIAN_POINT('Ctrl Pts',(60.5612197979217,250.620063462139,27.4182165512944)) ;
#108021=CARTESIAN_POINT('Ctrl Pts',(60.5755858845327,250.619468117123,27.4210603173112)) ;
#108022=CARTESIAN_POINT('Ctrl Pts',(60.5902651077865,250.619468117123,27.4210603173112)) ;
#108023=CARTESIAN_POINT('Origin',(60.5902651077865,245.619240674958,24.3483125582154)) ;
#108024=CARTESIAN_POINT('Ctrl Pts',(60.4402651077865,243.840203404936,25.6408587937931)) ;
#108025=CARTESIAN_POINT('Ctrl Pts',(60.4402651077865,243.8394292274,25.6407079681278)) ;
#108026=CARTESIAN_POINT('Ctrl Pts',(60.4402684378921,243.838655056638,25.6405570783182)) ;
#108027=CARTESIAN_POINT('Ctrl Pts',(60.4404467789386,243.817931397271,25.6365161805244)) ;
#108028=CARTESIAN_POINT('Ctrl Pts',(60.4428319502743,243.797914841084,25.6325687175194)) ;
#108029=CARTESIAN_POINT('Ctrl Pts',(60.4520052987548,243.759977742785,25.6250083928119)) ;
#108030=CARTESIAN_POINT('Ctrl Pts',(60.4586423249844,243.741836058232,25.621354832958)) ;
#108031=CARTESIAN_POINT('Ctrl Pts',(60.4774783235665,243.706232967992,25.6141229718641)) ;
#108032=CARTESIAN_POINT('Ctrl Pts',(60.4902886559452,243.688903025733,25.6105637433868)) ;
#108033=CARTESIAN_POINT('Ctrl Pts',(60.5183067650571,243.663740761485,25.6053629780756)) ;
#108034=CARTESIAN_POINT('Ctrl Pts',(60.5322233323112,243.654745812453,25.6034910268201)) ;
#108035=CARTESIAN_POINT('Ctrl Pts',(60.5612197979217,243.643368900052,25.6011186979124)) ;
#108036=CARTESIAN_POINT('Ctrl Pts',(60.5755858845327,243.640525134035,25.6005233528966)) ;
#108037=CARTESIAN_POINT('Ctrl Pts',(60.5902651077865,243.640525134035,25.6005233528966)) ;
#108038=CARTESIAN_POINT('Ctrl Pts',(60.5902651077865,243.31546952752,25.836690074996)) ;
#108039=CARTESIAN_POINT('Ctrl Pts',(60.5707376338846,243.315469527519,25.8366900749965)) ;
#108040=CARTESIAN_POINT('Ctrl Pts',(60.5513971100607,243.317641120579,25.8398257254355)) ;
#108041=CARTESIAN_POINT('Ctrl Pts',(60.5333315664698,243.321859600104,25.8459219612512)) ;
#108042=CARTESIAN_POINT('Ctrl Pts',(60.5152637963993,243.326078599533,25.8520189483946)) ;
#108043=CARTESIAN_POINT('Ctrl Pts',(60.4988172216938,243.332264099653,25.8609605795165)) ;
#108044=CARTESIAN_POINT('Ctrl Pts',(60.4849165768425,243.340061292122,25.8722475987304)) ;
#108045=CARTESIAN_POINT('Ctrl Pts',(60.4710122117667,243.34786057135,25.8835376386851)) ;
#108046=CARTESIAN_POINT('Ctrl Pts',(60.4599211853137,243.357122937908,25.8969584151118)) ;
#108047=CARTESIAN_POINT('Ctrl Pts',(60.452266539598,243.367318402121,25.9117600448443)) ;
#108048=CARTESIAN_POINT('Ctrl Pts',(60.4449239452532,243.377098235264,25.9259582673098)) ;
#108049=CARTESIAN_POINT('Ctrl Pts',(60.4408750760621,243.387560787867,25.9411723219294)) ;
#108050=CARTESIAN_POINT('Ctrl Pts',(60.4403288850239,243.398157412359,25.9566178371378)) ;
#108051=CARTESIAN_POINT('Ctrl Pts',(60.440286369022,243.398982263143,25.957820129938)) ;
#108052=CARTESIAN_POINT('Ctrl Pts',(60.4402651077865,243.399807320561,25.9590229387353)) ;
#108053=CARTESIAN_POINT('Ctrl Pts',(60.4402651077865,243.400632319557,25.9602258814026)) ;
#108054=CARTESIAN_POINT('Origin',(60.5902651077865,248.040265107786,23.0213203435596)) ;
#108055=CARTESIAN_POINT('Ctrl Pts',(60.4402651077865,243.452279656475,24.8795155697285)) ;
#108056=CARTESIAN_POINT('Ctrl Pts',(60.4402651077865,243.451946626863,24.8802305456133)) ;
#108057=CARTESIAN_POINT('Ctrl Pts',(60.4402684378921,243.451613653127,24.8809455537216)) ;
#108058=CARTESIAN_POINT('Ctrl Pts',(60.4404467789386,243.442701746765,24.9000865264635)) ;
#108059=CARTESIAN_POINT('Ctrl Pts',(60.4428319502743,243.434129874892,24.9186005211265)) ;
#108060=CARTESIAN_POINT('Ctrl Pts',(60.4520052987548,243.417947439168,24.9537361257336)) ;
#108061=CARTESIAN_POINT('Ctrl Pts',(60.4586423249844,243.410239816549,24.9705605654438)) ;
#108062=CARTESIAN_POINT('Ctrl Pts',(60.4774783235664,243.395163543695,25.0036148517977)) ;
#108063=CARTESIAN_POINT('Ctrl Pts',(60.4902886559451,243.387856735537,25.0197271316054)) ;
#108064=CARTESIAN_POINT('Ctrl Pts',(60.5183067650571,243.377274235219,25.0431407641495)) ;
#108065=CARTESIAN_POINT('Ctrl Pts',(60.5322233323112,243.373501577211,25.051518136121)) ;
#108066=CARTESIAN_POINT('Ctrl Pts',(60.5612197979217,243.368733650287,25.0621166715428)) ;
#108067=CARTESIAN_POINT('Ctrl Pts',(60.5755858845327,243.367543770797,25.0647672615988)) ;
#108068=CARTESIAN_POINT('Ctrl Pts',(60.5902651077865,243.367543770797,25.0647672615988)) ;
#108069=CARTESIAN_POINT('Origin',(60.5902651077865,245.878117316722,24.0913131340507)) ;
#108070=CARTESIAN_POINT('Ctrl Pts',(60.4402651077865,242.935532853835,25.0474167838717)) ;
#108071=CARTESIAN_POINT('Ctrl Pts',(60.4402651077865,242.936021132653,25.0487912940387)) ;
#108072=CARTESIAN_POINT('Ctrl Pts',(60.440286369022,242.936509268827,25.0501657727844)) ;
#108073=CARTESIAN_POINT('Ctrl Pts',(60.4403288850239,242.936997109009,25.0515397810631)) ;
#108074=CARTESIAN_POINT('Ctrl Pts',(60.4408750760621,242.943264253706,25.0691912764098)) ;
#108075=CARTESIAN_POINT('Ctrl Pts',(60.4449239452531,242.949422948319,25.0865982562063)) ;
#108076=CARTESIAN_POINT('Ctrl Pts',(60.452266539598,242.955161109892,25.1028558131956)) ;
#108077=CARTESIAN_POINT('Ctrl Pts',(60.4599211853139,242.961143136386,25.119804296676)) ;
#108078=CARTESIAN_POINT('Ctrl Pts',(60.4710122117669,242.966556490128,25.1351862430876)) ;
#108079=CARTESIAN_POINT('Ctrl Pts',(60.4849165768426,242.97110602301,25.1481321115104)) ;
#108080=CARTESIAN_POINT('Ctrl Pts',(60.4988172216939,242.975654338627,25.1610745161621)) ;
#108081=CARTESIAN_POINT('Ctrl Pts',(60.5152637963994,242.979252524414,25.1713344497827)) ;
#108082=CARTESIAN_POINT('Ctrl Pts',(60.5333315664698,242.981705224984,25.1783314111464)) ;
#108083=CARTESIAN_POINT('Ctrl Pts',(60.5513971100607,242.984157623309,25.185327510279)) ;
#108084=CARTESIAN_POINT('Ctrl Pts',(60.5707376338847,242.985417987428,25.1889274550538)) ;
#108085=CARTESIAN_POINT('Ctrl Pts',(60.5902651077865,242.985417987428,25.1889274550538)) ;
#108086=CARTESIAN_POINT('Origin',(60.5902651077865,250.050447394148,24.9137882607786)) ;
#108087=CARTESIAN_POINT('',(60.5902651077865,251.852827359384,26.4087041537722)) ;
#108088=CARTESIAN_POINT('',(60.5902651077865,252.1778829659,26.6448708758722)) ;
#108089=CARTESIAN_POINT('',(60.5902651077865,249.962279606305,25.0351408099348)) ;
#108090=CARTESIAN_POINT('Ctrl Pts',(60.5902651077865,252.177882965899,26.6448708758719)) ;
#108091=CARTESIAN_POINT('Ctrl Pts',(60.5707376338846,252.177882965899,26.6448708758719)) ;
#108092=CARTESIAN_POINT('Ctrl Pts',(60.5513971100607,252.180194087522,26.6418365988679)) ;
#108093=CARTESIAN_POINT('Ctrl Pts',(60.5333315664698,252.184688370456,26.6359407459586)) ;
#108094=CARTESIAN_POINT('Ctrl Pts',(60.5152637963993,252.189183207286,26.6300441664176)) ;
#108095=CARTESIAN_POINT('Ctrl Pts',(60.4988172216936,252.195775779175,26.6213982902475)) ;
#108096=CARTESIAN_POINT('Ctrl Pts',(60.4849165768425,252.204100907366,26.6104948387886)) ;
#108097=CARTESIAN_POINT('Ctrl Pts',(60.4710122117668,252.212428263609,26.599588469243)) ;
#108098=CARTESIAN_POINT('Ctrl Pts',(60.4599211853138,252.222329951809,26.5866321871782)) ;
#108099=CARTESIAN_POINT('Ctrl Pts',(60.452266539598,252.233256566511,26.5723617693702)) ;
#108100=CARTESIAN_POINT('Ctrl Pts',(60.4449239452532,252.243737743863,26.5586731032993)) ;
#108101=CARTESIAN_POINT('Ctrl Pts',(60.4408750760621,252.254974063087,26.544021223037)) ;
#108102=CARTESIAN_POINT('Ctrl Pts',(60.4403288850239,252.266389083925,26.5291703075782)) ;
#108103=CARTESIAN_POINT('Ctrl Pts',(60.440286369022,252.267277639417,26.5280142989575)) ;
#108104=CARTESIAN_POINT('Ctrl Pts',(60.4402651077865,252.268166621798,26.5268579343646)) ;
#108105=CARTESIAN_POINT('Ctrl Pts',(60.4402651077865,252.26905574955,26.5257015839662)) ;
#108106=CARTESIAN_POINT('Ctrl Pts',(60.4402651077865,251.829484664171,26.2063344963563)) ;
#108107=CARTESIAN_POINT('Ctrl Pts',(60.4402651077865,251.829580454454,26.2071173906402)) ;
#108108=CARTESIAN_POINT('Ctrl Pts',(60.4402684378921,251.82967618164,26.2079002983041)) ;
#108109=CARTESIAN_POINT('Ctrl Pts',(60.4404467789386,251.832237022391,26.2288583756768)) ;
#108110=CARTESIAN_POINT('Ctrl Pts',(60.4428319502743,251.834668218008,26.2491150850258)) ;
#108111=CARTESIAN_POINT('Ctrl Pts',(60.4520052987548,251.839201130021,26.2875316783904)) ;
#108112=CARTESIAN_POINT('Ctrl Pts',(60.4586423249844,251.841332476948,26.3059144577855)) ;
#108113=CARTESIAN_POINT('Ctrl Pts',(60.4774783235664,251.845456528266,26.3420097767374)) ;
#108114=CARTESIAN_POINT('Ctrl Pts',(60.4902886559451,251.847426747499,26.3595913933363)) ;
#108115=CARTESIAN_POINT('Ctrl Pts',(60.5183067650572,251.85025609303,26.3851292535789)) ;
#108116=CARTESIAN_POINT('Ctrl Pts',(60.5322233323112,251.851255353705,26.3942624232203)) ;
#108117=CARTESIAN_POINT('Ctrl Pts',(60.5612197979217,251.852514794114,26.4058155998437)) ;
#108118=CARTESIAN_POINT('Ctrl Pts',(60.5755858845327,251.852827359384,26.4087041537722)) ;
#108119=CARTESIAN_POINT('Ctrl Pts',(60.5902651077865,251.852827359384,26.4087041537722)) ;
#108120=CARTESIAN_POINT('Origin',(60.5902651077865,245.327670899104,23.5352272428401)) ;
#108121=CARTESIAN_POINT('Ctrl Pts',(60.4402651077865,243.236287157908,24.2147590127358)) ;
#108122=CARTESIAN_POINT('Ctrl Pts',(60.4402651077865,243.235597479012,24.2143763349887)) ;
#108123=CARTESIAN_POINT('Ctrl Pts',(60.4402684378921,243.234907826379,24.2139935983299)) ;
#108124=CARTESIAN_POINT('Ctrl Pts',(60.4404467789386,243.216447161187,24.2037465132216)) ;
#108125=CARTESIAN_POINT('Ctrl Pts',(60.4428319502744,243.198630118145,24.1938067967771)) ;
#108126=CARTESIAN_POINT('Ctrl Pts',(60.4520052987547,243.164886062416,24.1748932926071)) ;
#108127=CARTESIAN_POINT('Ctrl Pts',(60.4586423249843,243.14876130719,24.1658124618669)) ;
#108128=CARTESIAN_POINT('Ctrl Pts',(60.4774783235664,243.117135524196,24.1479325933122)) ;
#108129=CARTESIAN_POINT('Ctrl Pts',(60.490288655945,243.10175363177,24.1391923192063)) ;
#108130=CARTESIAN_POINT('Ctrl Pts',(60.5183067650571,243.079430021257,24.1264705301978)) ;
#108131=CARTESIAN_POINT('Ctrl Pts',(60.5322233323112,243.071453781117,24.1219106066435)) ;
#108132=CARTESIAN_POINT('Ctrl Pts',(60.5612197979217,243.061366784391,24.1161387285016)) ;
#108133=CARTESIAN_POINT('Ctrl Pts',(60.5755858845327,243.058846173917,24.1146937497176)) ;
#108134=CARTESIAN_POINT('Ctrl Pts',(60.5902651077865,243.058846173917,24.1146937497176)) ;
#108135=CARTESIAN_POINT('Ctrl Pts',(60.5902651077865,242.676720390548,24.2388539431728)) ;
#108136=CARTESIAN_POINT('Ctrl Pts',(60.5707376338847,242.676720390548,24.2388539431728)) ;
#108137=CARTESIAN_POINT('Ctrl Pts',(60.5513971100608,242.677816729004,24.2425071831162)) ;
#108138=CARTESIAN_POINT('Ctrl Pts',(60.5333315664699,242.679944900976,24.249608629777)) ;
#108139=CARTESIAN_POINT('Ctrl Pts',(60.5152637963994,242.682073335234,24.2567109516523)) ;
#108140=CARTESIAN_POINT('Ctrl Pts',(60.4988172216939,242.685192979455,24.2671263728531)) ;
#108141=CARTESIAN_POINT('Ctrl Pts',(60.4849165768427,242.689120669408,24.2802704310071)) ;
#108142=CARTESIAN_POINT('Ctrl Pts',(60.4710122117669,242.693049410527,24.2934180069008)) ;
#108143=CARTESIAN_POINT('Ctrl Pts',(60.4599211853139,242.697711196606,24.3090441524492)) ;
#108144=CARTESIAN_POINT('Ctrl Pts',(60.4522665395981,242.702833704151,24.3262719105652)) ;
#108145=CARTESIAN_POINT('Ctrl Pts',(60.4449239452532,242.707747386159,24.3427973572042)) ;
#108146=CARTESIAN_POINT('Ctrl Pts',(60.4408750760622,242.71299646356,24.3604998895482)) ;
#108147=CARTESIAN_POINT('Ctrl Pts',(60.4403288850239,242.718301525644,24.3784639844864)) ;
#108148=CARTESIAN_POINT('Ctrl Pts',(60.440286369022,242.718714476449,24.3798623257986)) ;
#108149=CARTESIAN_POINT('Ctrl Pts',(60.4402651077865,242.719127464324,24.3812612217067)) ;
#108150=CARTESIAN_POINT('Ctrl Pts',(60.4402651077865,242.719540355267,24.3826602268792)) ;
#108151=CARTESIAN_POINT('Origin',(60.5902651077865,248.040265107786,23.0213203435596)) ;
#108152=CARTESIAN_POINT('Ctrl Pts',(60.4402651077865,243.102617743897,23.3708035475559)) ;
#108153=CARTESIAN_POINT('Ctrl Pts',(60.4402651077865,243.102080074215,23.3713806182205)) ;
#108154=CARTESIAN_POINT('Ctrl Pts',(60.4402684378921,243.101542447717,23.3719577367977)) ;
#108155=CARTESIAN_POINT('Ctrl Pts',(60.4404467789386,243.087151835233,23.3874079531342)) ;
#108156=CARTESIAN_POINT('Ctrl Pts',(60.4428319502743,243.073278361647,23.4023669543188)) ;
#108157=CARTESIAN_POINT('Ctrl Pts',(60.4520052987548,243.047030451771,23.4307822523853)) ;
#108158=CARTESIAN_POINT('Ctrl Pts',(60.4586423249844,243.034501029262,23.4444014590289)) ;
#108159=CARTESIAN_POINT('Ctrl Pts',(60.4774783235664,243.009948305503,23.4711791289339)) ;
#108160=CARTESIAN_POINT('Ctrl Pts',(60.4902886559451,242.998020149712,23.4842448897419)) ;
#108161=CARTESIAN_POINT('Ctrl Pts',(60.5183067650572,242.98072038347,23.5032424051016)) ;
#108162=CARTESIAN_POINT('Ctrl Pts',(60.5322233323113,242.97454362218,23.5100439438662)) ;
#108163=CARTESIAN_POINT('Ctrl Pts',(60.5612197979217,242.966733926649,23.5186503795949)) ;
#108164=CARTESIAN_POINT('Ctrl Pts',(60.5755858845327,242.964783206634,23.5208035475559)) ;
#108165=CARTESIAN_POINT('Ctrl Pts',(60.5902651077865,242.964783206634,23.5208035475559)) ;
#108166=CARTESIAN_POINT('Origin',(60.5902651077865,245.653294405781,23.3708035475559)) ;
#108167=CARTESIAN_POINT('Ctrl Pts',(60.4402651077865,242.559278001425,23.3708035475559)) ;
#108168=CARTESIAN_POINT('Ctrl Pts',(60.4402651077865,242.559317635176,23.3722616708597)) ;
#108169=CARTESIAN_POINT('Ctrl Pts',(60.440286369022,242.559357142975,23.3737197202007)) ;
#108170=CARTESIAN_POINT('Ctrl Pts',(60.4403288850239,242.55939651465,23.3751772306343)) ;
#108171=CARTESIAN_POINT('Ctrl Pts',(60.4408750760621,242.559902311413,23.3939014545242)) ;
#108172=CARTESIAN_POINT('Ctrl Pts',(60.4449239452532,242.560380525479,23.4123596173871)) ;
#108173=CARTESIAN_POINT('Ctrl Pts',(60.4522665395981,242.560813980038,23.4295946623433)) ;
#108174=CARTESIAN_POINT('Ctrl Pts',(60.4599211853139,242.561265855891,23.4475621758458)) ;
#108175=CARTESIAN_POINT('Ctrl Pts',(60.4710122117669,242.561660978396,23.4638640945168)) ;
#108176=CARTESIAN_POINT('Ctrl Pts',(60.4849165768427,242.561987347939,23.4775822300163)) ;
#108177=CARTESIAN_POINT('Ctrl Pts',(60.498817221694,242.56231363016,23.4912966951184)) ;
#108178=CARTESIAN_POINT('Ctrl Pts',(60.5152637963995,242.562565214349,23.5021663724021)) ;
#108179=CARTESIAN_POINT('Ctrl Pts',(60.5333315664699,242.562735691238,23.5095788042595)) ;
#108180=CARTESIAN_POINT('Ctrl Pts',(60.5513971100607,242.56290614712,23.5169903226877)) ;
#108181=CARTESIAN_POINT('Ctrl Pts',(60.5707376338847,242.562992380514,23.5208035475559)) ;
#108182=CARTESIAN_POINT('Ctrl Pts',(60.5902651077865,242.562992380514,23.5208035475559)) ;
#108183=CARTESIAN_POINT('Origin',(60.5902651077865,250.536866817902,24.1999837998328)) ;
#108184=CARTESIAN_POINT('',(60.5902651077865,252.712986444776,25.0647672615988)) ;
#108185=CARTESIAN_POINT('',(60.5902651077865,253.095112228145,25.188927455054)) ;
#108186=CARTESIAN_POINT('',(60.5902651077865,250.490514268746,24.3426422772771)) ;
#108187=CARTESIAN_POINT('Ctrl Pts',(60.5902651077865,253.095112228145,25.1889274550539)) ;
#108188=CARTESIAN_POINT('Ctrl Pts',(60.5707376338848,253.095112228145,25.1889274550539)) ;
#108189=CARTESIAN_POINT('Ctrl Pts',(60.5513971100608,253.096372592264,25.1853275102792)) ;
#108190=CARTESIAN_POINT('Ctrl Pts',(60.5333315664699,253.098824990589,25.1783314111465)) ;
#108191=CARTESIAN_POINT('Ctrl Pts',(60.5152637963995,253.101277691159,25.1713344497829)) ;
#108192=CARTESIAN_POINT('Ctrl Pts',(60.4988172216938,253.104875876946,25.1610745161622)) ;
#108193=CARTESIAN_POINT('Ctrl Pts',(60.4849165768426,253.109424192563,25.1481321115104)) ;
#108194=CARTESIAN_POINT('Ctrl Pts',(60.4710122117668,253.113973725445,25.1351862430876)) ;
#108195=CARTESIAN_POINT('Ctrl Pts',(60.4599211853139,253.119387079187,25.119804296676)) ;
#108196=CARTESIAN_POINT('Ctrl Pts',(60.452266539598,253.125369105681,25.1028558131957)) ;
#108197=CARTESIAN_POINT('Ctrl Pts',(60.4449239452531,253.131107267254,25.0865982562064)) ;
#108198=CARTESIAN_POINT('Ctrl Pts',(60.4408750760621,253.137265961864,25.0691912764081)) ;
#108199=CARTESIAN_POINT('Ctrl Pts',(60.4403288850239,253.143533106564,25.051539781063)) ;
#108200=CARTESIAN_POINT('Ctrl Pts',(60.440286369022,253.144020946746,25.0501657727844)) ;
#108201=CARTESIAN_POINT('Ctrl Pts',(60.4402651077865,253.144509082921,25.0487912940391)) ;
#108202=CARTESIAN_POINT('Ctrl Pts',(60.4402651077865,253.144997361739,25.0474167838722)) ;
#108203=CARTESIAN_POINT('Ctrl Pts',(60.4402651077865,252.628250559098,24.8795155697285)) ;
#108204=CARTESIAN_POINT('Ctrl Pts',(60.4402651077865,252.62858358871,24.8802305456146)) ;
#108205=CARTESIAN_POINT('Ctrl Pts',(60.4402684378921,252.628916562447,24.8809455537241)) ;
#108206=CARTESIAN_POINT('Ctrl Pts',(60.4404467789389,252.637828468809,24.9000865264659)) ;
#108207=CARTESIAN_POINT('Ctrl Pts',(60.4428319502748,252.646400340681,24.9186005211289)) ;
#108208=CARTESIAN_POINT('Ctrl Pts',(60.4520052987552,252.662582776405,24.9537361257345)) ;
#108209=CARTESIAN_POINT('Ctrl Pts',(60.4586423249846,252.670290399024,24.9705605654442)) ;
#108210=CARTESIAN_POINT('Ctrl Pts',(60.4774783235664,252.685366671877,25.0036148517979)) ;
#108211=CARTESIAN_POINT('Ctrl Pts',(60.4902886559451,252.692673480035,25.0197271316054)) ;
#108212=CARTESIAN_POINT('Ctrl Pts',(60.5183067650571,252.703255980354,25.0431407641494)) ;
#108213=CARTESIAN_POINT('Ctrl Pts',(60.5322233323112,252.707028638362,25.051518136121)) ;
#108214=CARTESIAN_POINT('Ctrl Pts',(60.5612197979217,252.711796565285,25.0621166715428)) ;
#108215=CARTESIAN_POINT('Ctrl Pts',(60.5755858845327,252.712986444776,25.0647672615988)) ;
#108216=CARTESIAN_POINT('Ctrl Pts',(60.5902651077865,252.712986444776,25.0647672615988)) ;
#108217=CARTESIAN_POINT('Origin',(60.5902651077865,245.30162874415,22.6718371395634)) ;
#108218=CARTESIAN_POINT('Ctrl Pts',(60.4402651077865,243.102617743897,22.6718371395634)) ;
#108219=CARTESIAN_POINT('Ctrl Pts',(60.4402651077865,243.102080074216,22.6712600688998)) ;
#108220=CARTESIAN_POINT('Ctrl Pts',(60.440268437892,243.101542447719,22.6706829503236)) ;
#108221=CARTESIAN_POINT('Ctrl Pts',(60.4404467789383,243.087151835235,22.6552327339874)) ;
#108222=CARTESIAN_POINT('Ctrl Pts',(60.4428319502739,243.073278361649,22.6402737328024)) ;
#108223=CARTESIAN_POINT('Ctrl Pts',(60.4520052987543,243.047030451772,22.611858434735)) ;
#108224=CARTESIAN_POINT('Ctrl Pts',(60.4586423249841,243.034501029262,22.5982392280909)) ;
#108225=CARTESIAN_POINT('Ctrl Pts',(60.4774783235664,243.009948305503,22.5714615581854)) ;
#108226=CARTESIAN_POINT('Ctrl Pts',(60.4902886559451,242.998020149712,22.5583957973774)) ;
#108227=CARTESIAN_POINT('Ctrl Pts',(60.5183067650572,242.98072038347,22.5393982820177)) ;
#108228=CARTESIAN_POINT('Ctrl Pts',(60.5322233323112,242.97454362218,22.5325967432531)) ;
#108229=CARTESIAN_POINT('Ctrl Pts',(60.5612197979217,242.966733926649,22.5239903075244)) ;
#108230=CARTESIAN_POINT('Ctrl Pts',(60.5755858845327,242.964783206634,22.5218371395634)) ;
#108231=CARTESIAN_POINT('Ctrl Pts',(60.5902651077865,242.964783206634,22.5218371395634)) ;
#108232=CARTESIAN_POINT('Ctrl Pts',(60.5902651077865,242.562992380513,22.5218371395634)) ;
#108233=CARTESIAN_POINT('Ctrl Pts',(60.5707376338847,242.562992380513,22.5218371395634)) ;
#108234=CARTESIAN_POINT('Ctrl Pts',(60.5513971100607,242.562906147119,22.5256503644316)) ;
#108235=CARTESIAN_POINT('Ctrl Pts',(60.5333315664699,242.562735691238,22.5330618828598)) ;
#108236=CARTESIAN_POINT('Ctrl Pts',(60.5152637963995,242.562565214349,22.5404743147172)) ;
#108237=CARTESIAN_POINT('Ctrl Pts',(60.498817221694,242.56231363016,22.5513439920009)) ;
#108238=CARTESIAN_POINT('Ctrl Pts',(60.4849165768426,242.561987347939,22.5650584571031)) ;
#108239=CARTESIAN_POINT('Ctrl Pts',(60.4710122117667,242.561660978396,22.5787765926026)) ;
#108240=CARTESIAN_POINT('Ctrl Pts',(60.4599211853138,242.561265855892,22.5950785112737)) ;
#108241=CARTESIAN_POINT('Ctrl Pts',(60.452266539598,242.56081398004,22.6130460247761)) ;
#108242=CARTESIAN_POINT('Ctrl Pts',(60.4449239452532,242.560380525481,22.6302810697323)) ;
#108243=CARTESIAN_POINT('Ctrl Pts',(60.4408750760621,242.559902311412,22.6487392325954)) ;
#108244=CARTESIAN_POINT('Ctrl Pts',(60.4403288850239,242.559396514649,22.6674634564849)) ;
#108245=CARTESIAN_POINT('Ctrl Pts',(60.440286369022,242.559357142974,22.6689209669185)) ;
#108246=CARTESIAN_POINT('Ctrl Pts',(60.4402651077865,242.559317635176,22.6703790162596)) ;
#108247=CARTESIAN_POINT('Ctrl Pts',(60.4402651077865,242.559278001424,22.6718371395634)) ;
#108248=CARTESIAN_POINT('Origin',(60.5902651077865,248.040265107786,23.0213203435596)) ;
#108249=CARTESIAN_POINT('Ctrl Pts',(60.4402651077865,243.236287157908,21.8278816743835)) ;
#108250=CARTESIAN_POINT('Ctrl Pts',(60.4402651077865,243.235597479012,21.8282643521305)) ;
#108251=CARTESIAN_POINT('Ctrl Pts',(60.4402684378921,243.234907826379,21.8286470887893)) ;
#108252=CARTESIAN_POINT('Ctrl Pts',(60.4404467789386,243.216447161187,21.8388941738976)) ;
#108253=CARTESIAN_POINT('Ctrl Pts',(60.4428319502744,243.198630118145,21.8488338903421)) ;
#108254=CARTESIAN_POINT('Ctrl Pts',(60.4520052987547,243.164886062416,21.8677473945122)) ;
#108255=CARTESIAN_POINT('Ctrl Pts',(60.4586423249844,243.14876130719,21.8768282252524)) ;
#108256=CARTESIAN_POINT('Ctrl Pts',(60.4774783235664,243.117135524196,21.8947080938071)) ;
#108257=CARTESIAN_POINT('Ctrl Pts',(60.4902886559451,243.10175363177,21.903448367913)) ;
#108258=CARTESIAN_POINT('Ctrl Pts',(60.5183067650572,243.079430021257,21.9161701569215)) ;
#108259=CARTESIAN_POINT('Ctrl Pts',(60.5322233323112,243.071453781117,21.9207300804757)) ;
#108260=CARTESIAN_POINT('Ctrl Pts',(60.5612197979217,243.061366784391,21.9265019586177)) ;
#108261=CARTESIAN_POINT('Ctrl Pts',(60.5755858845327,243.058846173917,21.9279469374017)) ;
#108262=CARTESIAN_POINT('Ctrl Pts',(60.5902651077865,243.058846173917,21.9279469374017)) ;
#108263=CARTESIAN_POINT('Origin',(60.5902651077865,245.662124818155,22.6160841100613)) ;
#108264=CARTESIAN_POINT('Ctrl Pts',(60.4402651077865,242.719540355268,21.6599804602402)) ;
#108265=CARTESIAN_POINT('Ctrl Pts',(60.4402651077865,242.719127464324,21.6613794654127)) ;
#108266=CARTESIAN_POINT('Ctrl Pts',(60.440286369022,242.71871447645,21.6627783613207)) ;
#108267=CARTESIAN_POINT('Ctrl Pts',(60.4403288850239,242.718301525644,21.6641767026329)) ;
#108268=CARTESIAN_POINT('Ctrl Pts',(60.4408750760621,242.71299646356,21.6821407975714)) ;
#108269=CARTESIAN_POINT('Ctrl Pts',(60.4449239452532,242.707747386159,21.6998433299151)) ;
#108270=CARTESIAN_POINT('Ctrl Pts',(60.452266539598,242.702833704151,21.716368776554)) ;
#108271=CARTESIAN_POINT('Ctrl Pts',(60.4599211853138,242.697711196606,21.7335965346699)) ;
#108272=CARTESIAN_POINT('Ctrl Pts',(60.4710122117667,242.693049410527,21.7492226802185)) ;
#108273=CARTESIAN_POINT('Ctrl Pts',(60.4849165768426,242.689120669408,21.7623702561122)) ;
#108274=CARTESIAN_POINT('Ctrl Pts',(60.4988172216939,242.685192979455,21.7755143142664)) ;
#108275=CARTESIAN_POINT('Ctrl Pts',(60.5152637963995,242.682073335233,21.7859297354669)) ;
#108276=CARTESIAN_POINT('Ctrl Pts',(60.5333315664699,242.679944900976,21.7930320573423)) ;
#108277=CARTESIAN_POINT('Ctrl Pts',(60.5513971100607,242.677816729004,21.8001335040032)) ;
#108278=CARTESIAN_POINT('Ctrl Pts',(60.5707376338847,242.676720390548,21.8037867439466)) ;
#108279=CARTESIAN_POINT('Ctrl Pts',(60.5902651077865,242.676720390548,21.8037867439466)) ;
#108280=CARTESIAN_POINT('Origin',(60.5902651077865,250.778901471423,23.3708035475559)) ;
#108281=CARTESIAN_POINT('',(60.5902651077865,253.115747008939,23.5208035475559)) ;
#108282=CARTESIAN_POINT('',(60.5902651077865,253.517537835059,23.5208035475559)) ;
#108283=CARTESIAN_POINT('',(60.5902651077865,250.778901471423,23.5208035475559)) ;
#108284=CARTESIAN_POINT('Ctrl Pts',(60.5902651077865,253.517537835059,23.5208035475559)) ;
#108285=CARTESIAN_POINT('Ctrl Pts',(60.5707376338847,253.517537835059,23.5208035475559)) ;
#108286=CARTESIAN_POINT('Ctrl Pts',(60.5513971100607,253.517624068453,23.5169903226877)) ;
#108287=CARTESIAN_POINT('Ctrl Pts',(60.5333315664699,253.517794524334,23.5095788042595)) ;
#108288=CARTESIAN_POINT('Ctrl Pts',(60.5152637963995,253.517965001223,23.5021663724021)) ;
#108289=CARTESIAN_POINT('Ctrl Pts',(60.498817221694,253.518216585412,23.4912966951184)) ;
#108290=CARTESIAN_POINT('Ctrl Pts',(60.4849165768426,253.518542867633,23.4775822300162)) ;
#108291=CARTESIAN_POINT('Ctrl Pts',(60.4710122117667,253.518869237177,23.4638640945167)) ;
#108292=CARTESIAN_POINT('Ctrl Pts',(60.4599211853138,253.51926435968,23.4475621758456)) ;
#108293=CARTESIAN_POINT('Ctrl Pts',(60.452266539598,253.519716235533,23.4295946623432)) ;
#108294=CARTESIAN_POINT('Ctrl Pts',(60.4449239452532,253.520149690091,23.412359617387)) ;
#108295=CARTESIAN_POINT('Ctrl Pts',(60.4408750760621,253.52062790416,23.393901454524)) ;
#108296=CARTESIAN_POINT('Ctrl Pts',(60.4403288850239,253.521133700923,23.3751772306343)) ;
#108297=CARTESIAN_POINT('Ctrl Pts',(60.440286369022,253.521173072598,23.3737197202007)) ;
#108298=CARTESIAN_POINT('Ctrl Pts',(60.4402651077865,253.521212580397,23.3722616708597)) ;
#108299=CARTESIAN_POINT('Ctrl Pts',(60.4402651077865,253.521252214148,23.3708035475559)) ;
#108300=CARTESIAN_POINT('Ctrl Pts',(60.4402651077865,252.977912471676,23.3708035475559)) ;
#108301=CARTESIAN_POINT('Ctrl Pts',(60.4402651077865,252.978450141356,23.3713806182195)) ;
#108302=CARTESIAN_POINT('Ctrl Pts',(60.440268437892,252.978987767854,23.3719577367957)) ;
#108303=CARTESIAN_POINT('Ctrl Pts',(60.4404467789383,252.993378380338,23.3874079531319)) ;
#108304=CARTESIAN_POINT('Ctrl Pts',(60.4428319502739,253.007251853924,23.4023669543169)) ;
#108305=CARTESIAN_POINT('Ctrl Pts',(60.4520052987543,253.033499763801,23.4307822523842)) ;
#108306=CARTESIAN_POINT('Ctrl Pts',(60.4586423249841,253.04602918631,23.4444014590284)) ;
#108307=CARTESIAN_POINT('Ctrl Pts',(60.4774783235664,253.07058191007,23.4711791289339)) ;
#108308=CARTESIAN_POINT('Ctrl Pts',(60.4902886559451,253.08251006586,23.4842448897419)) ;
#108309=CARTESIAN_POINT('Ctrl Pts',(60.5183067650572,253.099809832103,23.5032424051016)) ;
#108310=CARTESIAN_POINT('Ctrl Pts',(60.5322233323112,253.105986593393,23.5100439438662)) ;
#108311=CARTESIAN_POINT('Ctrl Pts',(60.5612197979217,253.113796288923,23.5186503795949)) ;
#108312=CARTESIAN_POINT('Ctrl Pts',(60.5755858845327,253.115747008939,23.5208035475559)) ;
#108313=CARTESIAN_POINT('Ctrl Pts',(60.5902651077865,253.115747008939,23.5208035475559)) ;
#108314=CARTESIAN_POINT('Origin',(60.5902651077865,245.543663397671,21.8426568872864)) ;
#108315=CARTESIAN_POINT('Ctrl Pts',(60.4402651077865,243.452279656475,21.1631251173908)) ;
#108316=CARTESIAN_POINT('Ctrl Pts',(60.4402651077865,243.451946626863,21.162410141506)) ;
#108317=CARTESIAN_POINT('Ctrl Pts',(60.4402684378921,243.451613653127,21.1616951333977)) ;
#108318=CARTESIAN_POINT('Ctrl Pts',(60.4404467789386,243.442701746765,21.1425541606558)) ;
#108319=CARTESIAN_POINT('Ctrl Pts',(60.4428319502743,243.434129874892,21.1240401659927)) ;
#108320=CARTESIAN_POINT('Ctrl Pts',(60.4520052987547,243.417947439169,21.0889045613858)) ;
#108321=CARTESIAN_POINT('Ctrl Pts',(60.4586423249843,243.410239816549,21.0720801216756)) ;
#108322=CARTESIAN_POINT('Ctrl Pts',(60.4774783235664,243.395163543695,21.0390258353215)) ;
#108323=CARTESIAN_POINT('Ctrl Pts',(60.4902886559451,243.387856735537,21.0229135555139)) ;
#108324=CARTESIAN_POINT('Ctrl Pts',(60.5183067650571,243.377274235219,20.9994999229698)) ;
#108325=CARTESIAN_POINT('Ctrl Pts',(60.5322233323112,243.373501577211,20.9911225509982)) ;
#108326=CARTESIAN_POINT('Ctrl Pts',(60.5612197979217,243.368733650287,20.9805240155765)) ;
#108327=CARTESIAN_POINT('Ctrl Pts',(60.5755858845327,243.367543770797,20.9778734255204)) ;
#108328=CARTESIAN_POINT('Ctrl Pts',(60.5902651077865,243.367543770797,20.9778734255204)) ;
#108329=CARTESIAN_POINT('Ctrl Pts',(60.5902651077865,242.985417987427,20.853713232065)) ;
#108330=CARTESIAN_POINT('Ctrl Pts',(60.5707376338848,242.985417987427,20.853713232065)) ;
#108331=CARTESIAN_POINT('Ctrl Pts',(60.5513971100606,242.984157623308,20.8573131768398)) ;
#108332=CARTESIAN_POINT('Ctrl Pts',(60.5333315664698,242.981705224983,20.8643092759726)) ;
#108333=CARTESIAN_POINT('Ctrl Pts',(60.5152637963994,242.979252524414,20.8713062373364)) ;
#108334=CARTESIAN_POINT('Ctrl Pts',(60.4988172216939,242.975654338627,20.881566170957)) ;
#108335=CARTESIAN_POINT('Ctrl Pts',(60.4849165768425,242.97110602301,20.8945085756088)) ;
#108336=CARTESIAN_POINT('Ctrl Pts',(60.4710122117666,242.966556490128,20.9074544440317)) ;
#108337=CARTESIAN_POINT('Ctrl Pts',(60.4599211853137,242.961143136386,20.9228363904435)) ;
#108338=CARTESIAN_POINT('Ctrl Pts',(60.452266539598,242.955161109893,20.9397848739239)) ;
#108339=CARTESIAN_POINT('Ctrl Pts',(60.4449239452531,242.94942294832,20.9560424309132)) ;
#108340=CARTESIAN_POINT('Ctrl Pts',(60.4408750760621,242.943264253706,20.9734494107093)) ;
#108341=CARTESIAN_POINT('Ctrl Pts',(60.4403288850239,242.936997109009,20.9911009060562)) ;
#108342=CARTESIAN_POINT('Ctrl Pts',(60.440286369022,242.936509268827,20.992474914335)) ;
#108343=CARTESIAN_POINT('Ctrl Pts',(60.4402651077865,242.936021132652,20.9938493930803)) ;
#108344=CARTESIAN_POINT('Ctrl Pts',(60.4402651077865,242.935532853834,20.9952239032473)) ;
#108345=CARTESIAN_POINT('Origin',(60.5902651077865,248.040265107786,23.0213203435596)) ;
#108346=CARTESIAN_POINT('Ctrl Pts',(60.4402651077865,243.840203404936,20.4017818933262)) ;
#108347=CARTESIAN_POINT('Ctrl Pts',(60.4402651077865,243.8394292274,20.4019327189915)) ;
#108348=CARTESIAN_POINT('Ctrl Pts',(60.4402684378921,243.838655056638,20.402083608801)) ;
#108349=CARTESIAN_POINT('Ctrl Pts',(60.4404467789386,243.817931397271,20.4061245065949)) ;
#108350=CARTESIAN_POINT('Ctrl Pts',(60.4428319502743,243.797914841084,20.4100719696)) ;
#108351=CARTESIAN_POINT('Ctrl Pts',(60.4520052987548,243.759977742784,20.4176322943074)) ;
#108352=CARTESIAN_POINT('Ctrl Pts',(60.4586423249845,243.741836058232,20.4212858541613)) ;
#108353=CARTESIAN_POINT('Ctrl Pts',(60.4774783235665,243.706232967992,20.4285177152552)) ;
#108354=CARTESIAN_POINT('Ctrl Pts',(60.4902886559452,243.688903025733,20.4320769437325)) ;
#108355=CARTESIAN_POINT('Ctrl Pts',(60.5183067650571,243.663740761485,20.4372777090437)) ;
#108356=CARTESIAN_POINT('Ctrl Pts',(60.5322233323112,243.654745812453,20.4391496602992)) ;
#108357=CARTESIAN_POINT('Ctrl Pts',(60.5612197979217,243.643368900052,20.4415219892068)) ;
#108358=CARTESIAN_POINT('Ctrl Pts',(60.5755858845327,243.640525134035,20.4421173342227)) ;
#108359=CARTESIAN_POINT('Ctrl Pts',(60.5902651077865,243.640525134035,20.4421173342227)) ;
#108360=CARTESIAN_POINT('Origin',(60.5902651077865,245.903744171556,21.9010320185483)) ;
#108361=CARTESIAN_POINT('Ctrl Pts',(60.4402651077865,243.400632319557,20.0824148057165)) ;
#108362=CARTESIAN_POINT('Ctrl Pts',(60.4402651077865,243.399807320561,20.0836177483838)) ;
#108363=CARTESIAN_POINT('Ctrl Pts',(60.440286369022,243.398982263143,20.0848205571812)) ;
#108364=CARTESIAN_POINT('Ctrl Pts',(60.4403288850239,243.398157412359,20.0860228499813)) ;
#108365=CARTESIAN_POINT('Ctrl Pts',(60.4408750760622,243.387560787866,20.1014683651894)) ;
#108366=CARTESIAN_POINT('Ctrl Pts',(60.4449239452533,243.377098235265,20.1166824198105)) ;
#108367=CARTESIAN_POINT('Ctrl Pts',(60.452266539598,243.367318402122,20.1308806422757)) ;
#108368=CARTESIAN_POINT('Ctrl Pts',(60.4599211853137,243.357122937909,20.1456822720077)) ;
#108369=CARTESIAN_POINT('Ctrl Pts',(60.4710122117668,243.347860571349,20.1591030484335)) ;
#108370=CARTESIAN_POINT('Ctrl Pts',(60.4849165768427,243.340061292121,20.1703930883883)) ;
#108371=CARTESIAN_POINT('Ctrl Pts',(60.4988172216941,243.332264099652,20.1816801076022)) ;
#108372=CARTESIAN_POINT('Ctrl Pts',(60.5152637963994,243.326078599533,20.1906217387245)) ;
#108373=CARTESIAN_POINT('Ctrl Pts',(60.5333315664698,243.321859600104,20.1967187258679)) ;
#108374=CARTESIAN_POINT('Ctrl Pts',(60.5513971100607,243.317641120579,20.2028149616835)) ;
#108375=CARTESIAN_POINT('Ctrl Pts',(60.5707376338847,243.315469527519,20.2059506121225)) ;
#108376=CARTESIAN_POINT('Ctrl Pts',(60.5902651077865,243.315469527519,20.2059506121226)) ;
#108377=CARTESIAN_POINT('Origin',(60.5902651077865,250.752859316469,22.5074134442792)) ;
#108378=CARTESIAN_POINT('',(60.5902651077865,253.021684041655,21.9279469374017)) ;
#108379=CARTESIAN_POINT('',(60.5902651077865,253.403809825024,21.8037867439466)) ;
#108380=CARTESIAN_POINT('',(60.5902651077865,250.799211865625,22.6500719217234)) ;
#108381=CARTESIAN_POINT('Ctrl Pts',(60.5902651077865,253.403809825024,21.8037867439468)) ;
#108382=CARTESIAN_POINT('Ctrl Pts',(60.5707376338847,253.403809825025,21.8037867439465)) ;
#108383=CARTESIAN_POINT('Ctrl Pts',(60.5513971100607,253.402713486568,21.8001335040034)) ;
#108384=CARTESIAN_POINT('Ctrl Pts',(60.5333315664699,253.400585314596,21.7930320573425)) ;
#108385=CARTESIAN_POINT('Ctrl Pts',(60.5152637963994,253.398456880339,21.785929735467)) ;
#108386=CARTESIAN_POINT('Ctrl Pts',(60.4988172216939,253.395337236117,21.7755143142665)) ;
#108387=CARTESIAN_POINT('Ctrl Pts',(60.4849165768426,253.391409546164,21.7623702561124)) ;
#108388=CARTESIAN_POINT('Ctrl Pts',(60.4710122117668,253.387480805045,21.7492226802187)) ;
#108389=CARTESIAN_POINT('Ctrl Pts',(60.4599211853139,253.382819018967,21.73359653467)) ;
#108390=CARTESIAN_POINT('Ctrl Pts',(60.452266539598,253.377696511422,21.716368776554)) ;
#108391=CARTESIAN_POINT('Ctrl Pts',(60.4449239452532,253.372782829414,21.6998433299151)) ;
#108392=CARTESIAN_POINT('Ctrl Pts',(60.4408750760622,253.367533752023,21.682140797569)) ;
#108393=CARTESIAN_POINT('Ctrl Pts',(60.4403288850239,253.362228689928,21.6641767026334)) ;
#108394=CARTESIAN_POINT('Ctrl Pts',(60.440286369022,253.361815739121,21.662778361321)) ;
#108395=CARTESIAN_POINT('Ctrl Pts',(60.4402651077865,253.361402751249,21.6613794654128)) ;
#108396=CARTESIAN_POINT('Ctrl Pts',(60.4402651077865,253.360989860306,21.65998046024)) ;
#108397=CARTESIAN_POINT('Ctrl Pts',(60.4402651077865,252.844243057664,21.8278816743835)) ;
#108398=CARTESIAN_POINT('Ctrl Pts',(60.4402651077865,252.844932736563,21.8282643521315)) ;
#108399=CARTESIAN_POINT('Ctrl Pts',(60.440268437892,252.845622389192,21.8286470887883)) ;
#108400=CARTESIAN_POINT('Ctrl Pts',(60.4404467789386,252.864083054386,21.8388941738985)) ;
#108401=CARTESIAN_POINT('Ctrl Pts',(60.4428319502744,252.881900097428,21.8488338903423)) ;
#108402=CARTESIAN_POINT('Ctrl Pts',(60.4520052987548,252.915644153157,21.8677473945122)) ;
#108403=CARTESIAN_POINT('Ctrl Pts',(60.4586423249844,252.931768908382,21.8768282252524)) ;
#108404=CARTESIAN_POINT('Ctrl Pts',(60.4774783235665,252.963394691376,21.8947080938071)) ;
#108405=CARTESIAN_POINT('Ctrl Pts',(60.4902886559452,252.978776583802,21.903448367913)) ;
#108406=CARTESIAN_POINT('Ctrl Pts',(60.5183067650571,253.001100194315,21.9161701569214)) ;
#108407=CARTESIAN_POINT('Ctrl Pts',(60.5322233323112,253.009076434455,21.9207300804757)) ;
#108408=CARTESIAN_POINT('Ctrl Pts',(60.5612197979217,253.019163431181,21.9265019586177)) ;
#108409=CARTESIAN_POINT('Ctrl Pts',(60.5755858845327,253.021684041655,21.9279469374017)) ;
#108410=CARTESIAN_POINT('Ctrl Pts',(60.5902651077865,253.021684041655,21.9279469374017)) ;
#108411=CARTESIAN_POINT('Origin',(60.5902651077865,246.030082821424,21.1288524263407)) ;
#108412=CARTESIAN_POINT('Ctrl Pts',(60.4402651077865,244.251045551402,19.836306190763)) ;
#108413=CARTESIAN_POINT('Ctrl Pts',(60.4402651077865,244.250949761118,19.835523296477)) ;
#108414=CARTESIAN_POINT('Ctrl Pts',(60.440268437892,244.250854033933,19.8347403888173)) ;
#108415=CARTESIAN_POINT('Ctrl Pts',(60.4404467789386,244.248293193182,19.8137823114415)) ;
#108416=CARTESIAN_POINT('Ctrl Pts',(60.4428319502744,244.245861997565,19.7935256020932)) ;
#108417=CARTESIAN_POINT('Ctrl Pts',(60.4520052987548,244.241329085551,19.7551090087287)) ;
#108418=CARTESIAN_POINT('Ctrl Pts',(60.4586423249845,244.239197738625,19.7367262293337)) ;
#108419=CARTESIAN_POINT('Ctrl Pts',(60.4774783235665,244.235073687307,19.7006309103817)) ;
#108420=CARTESIAN_POINT('Ctrl Pts',(60.4902886559452,244.233103468073,19.6830492937829)) ;
#108421=CARTESIAN_POINT('Ctrl Pts',(60.5183067650571,244.230274122543,19.6575114335404)) ;
#108422=CARTESIAN_POINT('Ctrl Pts',(60.5322233323112,244.229274861868,19.648378263899)) ;
#108423=CARTESIAN_POINT('Ctrl Pts',(60.5612197979218,244.228015421459,19.6368250872756)) ;
#108424=CARTESIAN_POINT('Ctrl Pts',(60.5755858845328,244.227702856188,19.633936533347)) ;
#108425=CARTESIAN_POINT('Ctrl Pts',(60.5902651077866,244.227702856188,19.6339365333471)) ;
#108426=CARTESIAN_POINT('Ctrl Pts',(60.5902651077865,243.902647249673,19.3977698112473)) ;
#108427=CARTESIAN_POINT('Ctrl Pts',(60.5707376338847,243.902647249673,19.3977698112472)) ;
#108428=CARTESIAN_POINT('Ctrl Pts',(60.5513971100607,243.90033612805,19.4008040882514)) ;
#108429=CARTESIAN_POINT('Ctrl Pts',(60.5333315664699,243.895841845116,19.4066999411606)) ;
#108430=CARTESIAN_POINT('Ctrl Pts',(60.5152637963995,243.891347008286,19.4125965207015)) ;
#108431=CARTESIAN_POINT('Ctrl Pts',(60.4988172216941,243.884754436398,19.4212423968719)) ;
#108432=CARTESIAN_POINT('Ctrl Pts',(60.4849165768427,243.876429308206,19.4321458483307)) ;
#108433=CARTESIAN_POINT('Ctrl Pts',(60.4710122117668,243.868101951963,19.4430522178763)) ;
#108434=CARTESIAN_POINT('Ctrl Pts',(60.459921185314,243.858200263764,19.4560084999413)) ;
#108435=CARTESIAN_POINT('Ctrl Pts',(60.4522665395982,243.847273649063,19.4702789177496)) ;
#108436=CARTESIAN_POINT('Ctrl Pts',(60.4449239452534,243.836792471711,19.4839675838205)) ;
#108437=CARTESIAN_POINT('Ctrl Pts',(60.4408750760622,243.825556152481,19.4986194640776)) ;
#108438=CARTESIAN_POINT('Ctrl Pts',(60.4403288850239,243.814141131649,19.5134703795415)) ;
#108439=CARTESIAN_POINT('Ctrl Pts',(60.440286369022,243.813252576157,19.5146263881627)) ;
#108440=CARTESIAN_POINT('Ctrl Pts',(60.4402651077865,243.812363593775,19.5157827527548)) ;
#108441=CARTESIAN_POINT('Ctrl Pts',(60.4402651077865,243.811474466023,19.5169391031534)) ;
#108442=CARTESIAN_POINT('Origin',(60.5902651077865,248.040265107786,23.0213203435596)) ;
#108443=CARTESIAN_POINT('Ctrl Pts',(60.4402651077865,244.85525095499,19.2321007871753)) ;
#108444=CARTESIAN_POINT('Ctrl Pts',(60.4402651077865,244.854468060706,19.2320049968919)) ;
#108445=CARTESIAN_POINT('Ctrl Pts',(60.4402684378921,244.853685153042,19.2319092697064)) ;
#108446=CARTESIAN_POINT('Ctrl Pts',(60.4404467789386,244.83272707567,19.2293484289546)) ;
#108447=CARTESIAN_POINT('Ctrl Pts',(60.4428319502743,244.81247036632,19.226917233338)) ;
#108448=CARTESIAN_POINT('Ctrl Pts',(60.4520052987547,244.774053772956,19.2223843213245)) ;
#108449=CARTESIAN_POINT('Ctrl Pts',(60.4586423249843,244.755670993561,19.220252974398)) ;
#108450=CARTESIAN_POINT('Ctrl Pts',(60.4774783235665,244.719575674608,19.2161289230798)) ;
#108451=CARTESIAN_POINT('Ctrl Pts',(60.4902886559452,244.70199405801,19.2141587038466)) ;
#108452=CARTESIAN_POINT('Ctrl Pts',(60.5183067650571,244.676456197767,19.211329358316)) ;
#108453=CARTESIAN_POINT('Ctrl Pts',(60.5322233323112,244.667323028126,19.2103300976413)) ;
#108454=CARTESIAN_POINT('Ctrl Pts',(60.5612197979218,244.655769851502,19.2090706572321)) ;
#108455=CARTESIAN_POINT('Ctrl Pts',(60.5755858845328,244.652881297574,19.2087580919617)) ;
#108456=CARTESIAN_POINT('Ctrl Pts',(60.5902651077865,244.652881297574,19.2087580919617)) ;
#108457=CARTESIAN_POINT('Origin',(60.5902651077865,246.354501080212,21.2956415537952)) ;
#108458=CARTESIAN_POINT('Ctrl Pts',(60.4402651077865,244.53588386738,18.7925297017959)) ;
#108459=CARTESIAN_POINT('Ctrl Pts',(60.4402651077865,244.534727516982,18.7934188295481)) ;
#108460=CARTESIAN_POINT('Ctrl Pts',(60.440286369022,244.533571152388,18.7943078119286)) ;
#108461=CARTESIAN_POINT('Ctrl Pts',(60.4403288850239,244.532415143768,18.7951963674209)) ;
#108462=CARTESIAN_POINT('Ctrl Pts',(60.4408750760621,244.517564228315,18.8066113882632)) ;
#108463=CARTESIAN_POINT('Ctrl Pts',(60.4449239452531,244.502912348048,18.8178477074838)) ;
#108464=CARTESIAN_POINT('Ctrl Pts',(60.452266539598,244.489223681977,18.8283288848361)) ;
#108465=CARTESIAN_POINT('Ctrl Pts',(60.4599211853138,244.474953264169,18.8392554995377)) ;
#108466=CARTESIAN_POINT('Ctrl Pts',(60.471012211767,244.461996982103,18.8491571877367)) ;
#108467=CARTESIAN_POINT('Ctrl Pts',(60.4849165768427,244.451090612558,18.8574845439796)) ;
#108468=CARTESIAN_POINT('Ctrl Pts',(60.4988172216939,244.440187161099,18.8658096721714)) ;
#108469=CARTESIAN_POINT('Ctrl Pts',(60.5152637963994,244.431541284929,18.8724022440603)) ;
#108470=CARTESIAN_POINT('Ctrl Pts',(60.5333315664699,244.425644705388,18.8768970808899)) ;
#108471=CARTESIAN_POINT('Ctrl Pts',(60.5513971100608,244.419748852478,18.8813913638236)) ;
#108472=CARTESIAN_POINT('Ctrl Pts',(60.5707376338847,244.416714575474,18.8837024854465)) ;
#108473=CARTESIAN_POINT('Ctrl Pts',(60.5902651077865,244.416714575474,18.8837024854465)) ;
#108474=CARTESIAN_POINT('Origin',(60.5902651077865,250.461289540614,21.6943281289039)) ;
#108475=CARTESIAN_POINT('',(60.5902651077865,252.440005081538,20.4421173342227)) ;
#108476=CARTESIAN_POINT('',(60.5902651077865,252.765060688053,20.2059506121228)) ;
#108477=CARTESIAN_POINT('',(60.5902651077865,250.549457328458,21.8156806780601)) ;
#108478=CARTESIAN_POINT('Ctrl Pts',(60.5902651077865,252.765060688053,20.2059506121228)) ;
#108479=CARTESIAN_POINT('Ctrl Pts',(60.5707376338847,252.765060688053,20.2059506121228)) ;
#108480=CARTESIAN_POINT('Ctrl Pts',(60.5513971100607,252.762889094993,20.2028149616837)) ;
#108481=CARTESIAN_POINT('Ctrl Pts',(60.5333315664699,252.758670615469,20.1967187258679)) ;
#108482=CARTESIAN_POINT('Ctrl Pts',(60.5152637963996,252.75445161604,20.1906217387244)) ;
#108483=CARTESIAN_POINT('Ctrl Pts',(60.498817221694,252.74826611592,20.1816801076024)) ;
#108484=CARTESIAN_POINT('Ctrl Pts',(60.4849165768427,252.740468923451,20.1703930883885)) ;
#108485=CARTESIAN_POINT('Ctrl Pts',(60.4710122117669,252.732669644223,20.1591030484338)) ;
#108486=CARTESIAN_POINT('Ctrl Pts',(60.4599211853138,252.723407277664,20.1456822720077)) ;
#108487=CARTESIAN_POINT('Ctrl Pts',(60.4522665395981,252.713211813451,20.1308806422753)) ;
#108488=CARTESIAN_POINT('Ctrl Pts',(60.4449239452532,252.703431980308,20.1166824198097)) ;
#108489=CARTESIAN_POINT('Ctrl Pts',(60.4408750760621,252.692969427699,20.1014683651929)) ;
#108490=CARTESIAN_POINT('Ctrl Pts',(60.4403288850239,252.682372803215,20.086022849981)) ;
#108491=CARTESIAN_POINT('Ctrl Pts',(60.440286369022,252.681547952431,20.0848205571807)) ;
#108492=CARTESIAN_POINT('Ctrl Pts',(60.4402651077865,252.680722895011,20.0836177483837)) ;
#108493=CARTESIAN_POINT('Ctrl Pts',(60.4402651077865,252.679897896016,20.0824148057166)) ;
#108494=CARTESIAN_POINT('Ctrl Pts',(60.4402651077865,252.240326810636,20.4017818933262)) ;
#108495=CARTESIAN_POINT('Ctrl Pts',(60.4402651077865,252.241100988172,20.4019327189915)) ;
#108496=CARTESIAN_POINT('Ctrl Pts',(60.4402684378921,252.241875158935,20.402083608801)) ;
#108497=CARTESIAN_POINT('Ctrl Pts',(60.4404467789386,252.262598818301,20.4061245065945)) ;
#108498=CARTESIAN_POINT('Ctrl Pts',(60.4428319502743,252.282615374488,20.4100719695999)) ;
#108499=CARTESIAN_POINT('Ctrl Pts',(60.4520052987548,252.320552472788,20.4176322943074)) ;
#108500=CARTESIAN_POINT('Ctrl Pts',(60.4586423249844,252.338694157341,20.4212858541613)) ;
#108501=CARTESIAN_POINT('Ctrl Pts',(60.4774783235665,252.374297247581,20.4285177152552)) ;
#108502=CARTESIAN_POINT('Ctrl Pts',(60.4902886559452,252.39162718984,20.4320769437325)) ;
#108503=CARTESIAN_POINT('Ctrl Pts',(60.5183067650572,252.416789454087,20.4372777090437)) ;
#108504=CARTESIAN_POINT('Ctrl Pts',(60.5322233323113,252.42578440312,20.4391496602992)) ;
#108505=CARTESIAN_POINT('Ctrl Pts',(60.5612197979218,252.437161315521,20.4415219892068)) ;
#108506=CARTESIAN_POINT('Ctrl Pts',(60.5755858845328,252.440005081538,20.4421173342227)) ;
#108507=CARTESIAN_POINT('Ctrl Pts',(60.5902651077866,252.440005081538,20.4421173342227)) ;
#108508=CARTESIAN_POINT('Origin',(60.5902651077865,246.713272893131,20.6002959107317)) ;
#108509=CARTESIAN_POINT('Ctrl Pts',(60.4402651077865,245.420726657553,18.8212586407095)) ;
#108510=CARTESIAN_POINT('Ctrl Pts',(60.4402651077865,245.420877483218,18.8204844631737)) ;
#108511=CARTESIAN_POINT('Ctrl Pts',(60.4402684378921,245.421028373028,18.8197102924111)) ;
#108512=CARTESIAN_POINT('Ctrl Pts',(60.4404467789386,245.425069270821,18.7989866330451)) ;
#108513=CARTESIAN_POINT('Ctrl Pts',(60.4428319502743,245.429016733827,18.7789700768575)) ;
#108514=CARTESIAN_POINT('Ctrl Pts',(60.4520052987547,245.436577058534,18.7410329785581)) ;
#108515=CARTESIAN_POINT('Ctrl Pts',(60.4586423249843,245.440230618388,18.7228912940055)) ;
#108516=CARTESIAN_POINT('Ctrl Pts',(60.4774783235664,245.447462479482,18.6872882037655)) ;
#108517=CARTESIAN_POINT('Ctrl Pts',(60.4902886559451,245.451021707959,18.6699582615064)) ;
#108518=CARTESIAN_POINT('Ctrl Pts',(60.5183067650571,245.45622247327,18.6447959972586)) ;
#108519=CARTESIAN_POINT('Ctrl Pts',(60.5322233323112,245.458094424526,18.6358010482264)) ;
#108520=CARTESIAN_POINT('Ctrl Pts',(60.5612197979217,245.460466753434,18.6244241358249)) ;
#108521=CARTESIAN_POINT('Ctrl Pts',(60.5755858845327,245.461062098449,18.6215803698081)) ;
#108522=CARTESIAN_POINT('Ctrl Pts',(60.5902651077865,245.461062098449,18.6215803698081)) ;
#108523=CARTESIAN_POINT('Ctrl Pts',(60.5902651077865,245.22489537635,18.2965247632932)) ;
#108524=CARTESIAN_POINT('Ctrl Pts',(60.5707376338848,245.22489537635,18.2965247632932)) ;
#108525=CARTESIAN_POINT('Ctrl Pts',(60.5513971100606,245.22175972591,18.2986963563521)) ;
#108526=CARTESIAN_POINT('Ctrl Pts',(60.5333315664697,245.215663490095,18.3029148358767)) ;
#108527=CARTESIAN_POINT('Ctrl Pts',(60.5152637963993,245.209566502951,18.3071338353058)) ;
#108528=CARTESIAN_POINT('Ctrl Pts',(60.4988172216938,245.200624871829,18.3133193354258)) ;
#108529=CARTESIAN_POINT('Ctrl Pts',(60.4849165768424,245.189337852615,18.3211165278944)) ;
#108530=CARTESIAN_POINT('Ctrl Pts',(60.4710122117664,245.17804781266,18.3289158071227)) ;
#108531=CARTESIAN_POINT('Ctrl Pts',(60.4599211853135,245.164627036234,18.3381781736818)) ;
#108532=CARTESIAN_POINT('Ctrl Pts',(60.4522665395978,245.149825406502,18.3483736378946)) ;
#108533=CARTESIAN_POINT('Ctrl Pts',(60.444923945253,245.135627184036,18.3581534710381)) ;
#108534=CARTESIAN_POINT('Ctrl Pts',(60.440875076062,245.120413129419,18.3686160236467)) ;
#108535=CARTESIAN_POINT('Ctrl Pts',(60.4403288850238,245.104967614207,18.3792126481315)) ;
#108536=CARTESIAN_POINT('Ctrl Pts',(60.440286369022,245.103765321407,18.3800374989151)) ;
#108537=CARTESIAN_POINT('Ctrl Pts',(60.4402651077865,245.10256251261,18.3808625563344)) ;
#108538=CARTESIAN_POINT('Ctrl Pts',(60.4402651077865,245.101359569943,18.3816875553301)) ;
#108539=CARTESIAN_POINT('Origin',(60.5902651077865,248.040265107786,23.0213203435596)) ;
#108540=CARTESIAN_POINT('Ctrl Pts',(60.4402651077865,246.182069881617,18.4333348922484)) ;
#108541=CARTESIAN_POINT('Ctrl Pts',(60.4402651077865,246.181354905733,18.4330018626367)) ;
#108542=CARTESIAN_POINT('Ctrl Pts',(60.4402684378921,246.180639897624,18.4326688888999)) ;
#108543=CARTESIAN_POINT('Ctrl Pts',(60.4404467789386,246.161498924883,18.4237569825383)) ;
#108544=CARTESIAN_POINT('Ctrl Pts',(60.4428319502743,246.142984930219,18.4151851106656)) ;
#108545=CARTESIAN_POINT('Ctrl Pts',(60.4520052987548,246.107849325612,18.3990026749417)) ;
#108546=CARTESIAN_POINT('Ctrl Pts',(60.4586423249844,246.091024885902,18.3912950523219)) ;
#108547=CARTESIAN_POINT('Ctrl Pts',(60.4774783235664,246.057970599548,18.3762187794687)) ;
#108548=CARTESIAN_POINT('Ctrl Pts',(60.4902886559451,246.04185831974,18.3689119713107)) ;
#108549=CARTESIAN_POINT('Ctrl Pts',(60.5183067650572,246.018444687196,18.3583294709921)) ;
#108550=CARTESIAN_POINT('Ctrl Pts',(60.5322233323112,246.010067315225,18.3545568129842)) ;
#108551=CARTESIAN_POINT('Ctrl Pts',(60.5612197979218,245.999468779803,18.3497888860605)) ;
#108552=CARTESIAN_POINT('Ctrl Pts',(60.5755858845328,245.996818189747,18.3485990065702)) ;
#108553=CARTESIAN_POINT('Ctrl Pts',(60.5902651077866,245.996818189747,18.3485990065702)) ;
#108554=CARTESIAN_POINT('Origin',(60.5902651077865,246.970272317295,20.8591725524954)) ;
#108555=CARTESIAN_POINT('Ctrl Pts',(60.4402651077865,246.014168667474,17.9165880896081)) ;
#108556=CARTESIAN_POINT('Ctrl Pts',(60.4402651077865,246.012794157307,17.9170763684262)) ;
#108557=CARTESIAN_POINT('Ctrl Pts',(60.440286369022,246.011419678562,17.9175645046008)) ;
#108558=CARTESIAN_POINT('Ctrl Pts',(60.4403288850238,246.010045670283,17.9180523447825)) ;
#108559=CARTESIAN_POINT('Ctrl Pts',(60.440875076062,245.992394174936,17.9243194894788)) ;
#108560=CARTESIAN_POINT('Ctrl Pts',(60.444923945253,245.97498719514,17.9304781840928)) ;
#108561=CARTESIAN_POINT('Ctrl Pts',(60.4522665395979,245.958729638151,17.9362163456658)) ;
#108562=CARTESIAN_POINT('Ctrl Pts',(60.4599211853138,245.94178115467,17.9421983721592)) ;
#108563=CARTESIAN_POINT('Ctrl Pts',(60.4710122117668,245.926399208258,17.9476117259011)) ;
#108564=CARTESIAN_POINT('Ctrl Pts',(60.4849165768426,245.913453339835,17.9521612587828)) ;
#108565=CARTESIAN_POINT('Ctrl Pts',(60.4988172216937,245.900510935184,17.9567095744005)) ;
#108566=CARTESIAN_POINT('Ctrl Pts',(60.5152637963994,245.890251001563,17.9603077601871)) ;
#108567=CARTESIAN_POINT('Ctrl Pts',(60.5333315664698,245.883254040199,17.9627604607569)) ;
#108568=CARTESIAN_POINT('Ctrl Pts',(60.5513971100606,245.876257941067,17.965212859082)) ;
#108569=CARTESIAN_POINT('Ctrl Pts',(60.5707376338847,245.872657996292,17.966473223201)) ;
#108570=CARTESIAN_POINT('Ctrl Pts',(60.5902651077865,245.872657996292,17.966473223201)) ;
#108571=CARTESIAN_POINT('Origin',(60.5902651077865,249.932733025005,21.0111380571975)) ;
#108572=CARTESIAN_POINT('',(60.5902651077865,251.427648917999,19.2087580919617)) ;
#108573=CARTESIAN_POINT('',(60.5902651077865,251.663815640099,18.8837024854464)) ;
#108574=CARTESIAN_POINT('',(60.5902651077865,250.054085574161,21.0993058450414)) ;
#108575=CARTESIAN_POINT('Ctrl Pts',(60.5902651077865,251.663815640098,18.8837024854471)) ;
#108576=CARTESIAN_POINT('Ctrl Pts',(60.5707376338847,251.663815640098,18.8837024854471)) ;
#108577=CARTESIAN_POINT('Ctrl Pts',(60.5513971100607,251.660781363094,18.8813913638241)) ;
#108578=CARTESIAN_POINT('Ctrl Pts',(60.53333156647,251.654885510185,18.8768970808902)) ;
#108579=CARTESIAN_POINT('Ctrl Pts',(60.5152637963997,251.648988930644,18.8724022440604)) ;
#108580=CARTESIAN_POINT('Ctrl Pts',(60.498817221694,251.640343054474,18.8658096721712)) ;
#108581=CARTESIAN_POINT('Ctrl Pts',(60.4849165768427,251.629439603015,18.8574845439796)) ;
#108582=CARTESIAN_POINT('Ctrl Pts',(60.4710122117668,251.618533233469,18.8491571877369)) ;
#108583=CARTESIAN_POINT('Ctrl Pts',(60.459921185314,251.605576951404,18.8392554995377)) ;
#108584=CARTESIAN_POINT('Ctrl Pts',(60.4522665395982,251.591306533596,18.8283288848364)) ;
#108585=CARTESIAN_POINT('Ctrl Pts',(60.4449239452533,251.577617867525,18.8178477074843)) ;
#108586=CARTESIAN_POINT('Ctrl Pts',(60.4408750760622,251.562965987259,18.8066113882618)) ;
#108587=CARTESIAN_POINT('Ctrl Pts',(60.4403288850239,251.548115071805,18.7951963674209)) ;
#108588=CARTESIAN_POINT('Ctrl Pts',(60.4402863690221,251.546959063185,18.7943078119287)) ;
#108589=CARTESIAN_POINT('Ctrl Pts',(60.4402651077865,251.54580269859,18.7934188295486)) ;
#108590=CARTESIAN_POINT('Ctrl Pts',(60.4402651077865,251.544646348192,18.7925297017964)) ;
#108591=CARTESIAN_POINT('Ctrl Pts',(60.4402651077865,251.225279260583,19.2321007871753)) ;
#108592=CARTESIAN_POINT('Ctrl Pts',(60.4402651077865,251.226062154867,19.2320049968919)) ;
#108593=CARTESIAN_POINT('Ctrl Pts',(60.4402684378921,251.226845062531,19.2319092697064)) ;
#108594=CARTESIAN_POINT('Ctrl Pts',(60.4404467789386,251.247803139903,19.2293484289546)) ;
#108595=CARTESIAN_POINT('Ctrl Pts',(60.4428319502743,251.268059849252,19.226917233338)) ;
#108596=CARTESIAN_POINT('Ctrl Pts',(60.4520052987547,251.306476442617,19.2223843213245)) ;
#108597=CARTESIAN_POINT('Ctrl Pts',(60.4586423249844,251.324859222012,19.220252974398)) ;
#108598=CARTESIAN_POINT('Ctrl Pts',(60.4774783235664,251.360954540964,19.2161289230799)) ;
#108599=CARTESIAN_POINT('Ctrl Pts',(60.4902886559451,251.378536157563,19.2141587038466)) ;
#108600=CARTESIAN_POINT('Ctrl Pts',(60.5183067650571,251.404074017805,19.211329358316)) ;
#108601=CARTESIAN_POINT('Ctrl Pts',(60.5322233323112,251.413207187447,19.2103300976413)) ;
#108602=CARTESIAN_POINT('Ctrl Pts',(60.5612197979217,251.42476036407,19.2090706572321)) ;
#108603=CARTESIAN_POINT('Ctrl Pts',(60.5755858845327,251.427648917999,19.2087580919617)) ;
#108604=CARTESIAN_POINT('Ctrl Pts',(60.5902651077865,251.427648917999,19.2087580919617)) ;
#108605=CARTESIAN_POINT('Origin',(60.5902651077865,247.526358208506,20.3087261348769)) ;
#108606=CARTESIAN_POINT('Ctrl Pts',(60.4402651077865,246.84682643861,18.2173423936815)) ;
#108607=CARTESIAN_POINT('Ctrl Pts',(60.4402651077865,246.847209116357,18.2166527147851)) ;
#108608=CARTESIAN_POINT('Ctrl Pts',(60.4402684378921,246.847591853016,18.2159630621521)) ;
#108609=CARTESIAN_POINT('Ctrl Pts',(60.4404467789386,246.857838938124,18.197502396961)) ;
#108610=CARTESIAN_POINT('Ctrl Pts',(60.4428319502743,246.867778654569,18.1796853539185)) ;
#108611=CARTESIAN_POINT('Ctrl Pts',(60.4520052987548,246.886692158739,18.1459412981889)) ;
#108612=CARTESIAN_POINT('Ctrl Pts',(60.4586423249845,246.895772989479,18.1298165429636)) ;
#108613=CARTESIAN_POINT('Ctrl Pts',(60.4774783235664,246.913652858034,18.0981907599697)) ;
#108614=CARTESIAN_POINT('Ctrl Pts',(60.4902886559451,246.92239313214,18.0828088675435)) ;
#108615=CARTESIAN_POINT('Ctrl Pts',(60.5183067650572,246.935114921148,18.0604852570307)) ;
#108616=CARTESIAN_POINT('Ctrl Pts',(60.5322233323113,246.939674844702,18.0525090168905)) ;
#108617=CARTESIAN_POINT('Ctrl Pts',(60.5612197979218,246.945446722844,18.0424220201645)) ;
#108618=CARTESIAN_POINT('Ctrl Pts',(60.5755858845328,246.946891701628,18.0399014096908)) ;
#108619=CARTESIAN_POINT('Ctrl Pts',(60.5902651077866,246.946891701628,18.0399014096908)) ;
#108620=CARTESIAN_POINT('Ctrl Pts',(60.5902651077865,246.822731508173,17.6577756263214)) ;
#108621=CARTESIAN_POINT('Ctrl Pts',(60.5707376338846,246.822731508173,17.6577756263213)) ;
#108622=CARTESIAN_POINT('Ctrl Pts',(60.5513971100607,246.81907826823,17.6588719647777)) ;
#108623=CARTESIAN_POINT('Ctrl Pts',(60.5333315664699,246.811976821569,17.6610001367495)) ;
#108624=CARTESIAN_POINT('Ctrl Pts',(60.5152637963995,246.804874499694,17.6631285710069)) ;
#108625=CARTESIAN_POINT('Ctrl Pts',(60.4988172216938,246.794459078493,17.6662482152286)) ;
#108626=CARTESIAN_POINT('Ctrl Pts',(60.4849165768425,246.781315020339,17.6701759051817)) ;
#108627=CARTESIAN_POINT('Ctrl Pts',(60.4710122117665,246.768167444445,17.6741046463009)) ;
#108628=CARTESIAN_POINT('Ctrl Pts',(60.4599211853139,246.752541298897,17.6787664323798)) ;
#108629=CARTESIAN_POINT('Ctrl Pts',(60.452266539598,246.735313540781,17.6838889399248)) ;
#108630=CARTESIAN_POINT('Ctrl Pts',(60.4449239452532,246.718788094142,17.6888026219327)) ;
#108631=CARTESIAN_POINT('Ctrl Pts',(60.4408750760621,246.701085561798,17.6940516993334)) ;
#108632=CARTESIAN_POINT('Ctrl Pts',(60.4403288850239,246.683121466859,17.6993567614171)) ;
#108633=CARTESIAN_POINT('Ctrl Pts',(60.440286369022,246.681723125547,17.6997697122226)) ;
#108634=CARTESIAN_POINT('Ctrl Pts',(60.4402651077865,246.680324229639,17.7001827000972)) ;
#108635=CARTESIAN_POINT('Ctrl Pts',(60.4402651077865,246.678925224467,17.7005955910407)) ;
#108636=CARTESIAN_POINT('Origin',(60.5902651077865,248.040265107786,23.0213203435596)) ;
#108637=CARTESIAN_POINT('Ctrl Pts',(60.4402651077865,247.69078190379,18.0836729796702)) ;
#108638=CARTESIAN_POINT('Ctrl Pts',(60.4402651077865,247.690204833125,18.0831353099888)) ;
#108639=CARTESIAN_POINT('Ctrl Pts',(60.4402684378921,247.689627714548,18.0825976834901)) ;
#108640=CARTESIAN_POINT('Ctrl Pts',(60.4404467789386,247.674177498212,18.0682070710063)) ;
#108641=CARTESIAN_POINT('Ctrl Pts',(60.4428319502743,247.659218497027,18.0543335974202)) ;
#108642=CARTESIAN_POINT('Ctrl Pts',(60.4520052987548,247.630803198961,18.0280856875442)) ;
#108643=CARTESIAN_POINT('Ctrl Pts',(60.4586423249844,247.617183992317,18.0155562650352)) ;
#108644=CARTESIAN_POINT('Ctrl Pts',(60.4774783235665,247.590406322412,17.9910035412763)) ;
#108645=CARTESIAN_POINT('Ctrl Pts',(60.4902886559452,247.577340561604,17.9790753854857)) ;
#108646=CARTESIAN_POINT('Ctrl Pts',(60.5183067650572,247.558343046244,17.9617756192428)) ;
#108647=CARTESIAN_POINT('Ctrl Pts',(60.5322233323113,247.55154150748,17.9555988579533)) ;
#108648=CARTESIAN_POINT('Ctrl Pts',(60.5612197979218,247.542935071751,17.9477891624225)) ;
#108649=CARTESIAN_POINT('Ctrl Pts',(60.5755858845328,247.54078190379,17.9458384424072)) ;
#108650=CARTESIAN_POINT('Ctrl Pts',(60.5902651077866,247.54078190379,17.9458384424072)) ;
#108651=CARTESIAN_POINT('Origin',(60.5902651077865,247.69078190379,20.6343496415544)) ;
#108652=CARTESIAN_POINT('Ctrl Pts',(60.4402651077865,247.69078190379,17.5403332371979)) ;
#108653=CARTESIAN_POINT('Ctrl Pts',(60.4402651077865,247.689323780486,17.5403728709491)) ;
#108654=CARTESIAN_POINT('Ctrl Pts',(60.440286369022,247.687865731145,17.5404123787479)) ;
#108655=CARTESIAN_POINT('Ctrl Pts',(60.4403288850239,247.686408220711,17.540451750423)) ;
#108656=CARTESIAN_POINT('Ctrl Pts',(60.4408750760621,247.667683996822,17.5409575471857)) ;
#108657=CARTESIAN_POINT('Ctrl Pts',(60.4449239452531,247.649225833959,17.5414357612546)) ;
#108658=CARTESIAN_POINT('Ctrl Pts',(60.452266539598,247.631990789003,17.5418692158132)) ;
#108659=CARTESIAN_POINT('Ctrl Pts',(60.4599211853139,247.6140232755,17.5423210916658)) ;
#108660=CARTESIAN_POINT('Ctrl Pts',(60.4710122117669,247.597721356829,17.5427162141691)) ;
#108661=CARTESIAN_POINT('Ctrl Pts',(60.4849165768426,247.58400322133,17.5430425837128)) ;
#108662=CARTESIAN_POINT('Ctrl Pts',(60.4988172216937,247.570288756228,17.5433688659337)) ;
#108663=CARTESIAN_POINT('Ctrl Pts',(60.5152637963994,247.559419078944,17.5436204501225)) ;
#108664=CARTESIAN_POINT('Ctrl Pts',(60.5333315664699,247.552006647086,17.5437909270115)) ;
#108665=CARTESIAN_POINT('Ctrl Pts',(60.5513971100608,247.544595128658,17.5439613828928)) ;
#108666=CARTESIAN_POINT('Ctrl Pts',(60.5707376338847,247.54078190379,17.5440476162862)) ;
#108667=CARTESIAN_POINT('Ctrl Pts',(60.5902651077865,247.54078190379,17.5440476162862)) ;
#108668=CARTESIAN_POINT('Origin',(60.5902651077865,249.21892856406,20.5247186334439)) ;
#108669=CARTESIAN_POINT('Ctrl Pts',(60.5902651077865,250.207872219281,17.9664732232009)) ;
#108670=CARTESIAN_POINT('Ctrl Pts',(60.5707376338848,250.207872219281,17.9664732232009)) ;
#108671=CARTESIAN_POINT('Ctrl Pts',(60.5513971100606,250.204272274506,17.9652128590817)) ;
#108672=CARTESIAN_POINT('Ctrl Pts',(60.5333315664697,250.197276175374,17.9627604607566)) ;
#108673=CARTESIAN_POINT('Ctrl Pts',(60.5152637963994,250.19027921401,17.9603077601868)) ;
#108674=CARTESIAN_POINT('Ctrl Pts',(60.4988172216938,250.180019280389,17.9567095744006)) ;
#108675=CARTESIAN_POINT('Ctrl Pts',(60.4849165768424,250.167076875737,17.952161258783)) ;
#108676=CARTESIAN_POINT('Ctrl Pts',(60.4710122117664,250.154131007314,17.9476117259013)) ;
#108677=CARTESIAN_POINT('Ctrl Pts',(60.4599211853138,250.138749060903,17.9421983721593)) ;
#108678=CARTESIAN_POINT('Ctrl Pts',(60.452266539598,250.121800577423,17.9362163456661)) ;
#108679=CARTESIAN_POINT('Ctrl Pts',(60.4449239452531,250.105543020433,17.9304781840933)) ;
#108680=CARTESIAN_POINT('Ctrl Pts',(60.440875076062,250.088136040637,17.9243194894782)) ;
#108681=CARTESIAN_POINT('Ctrl Pts',(60.4403288850239,250.07048454529,17.9180523447823)) ;
#108682=CARTESIAN_POINT('Ctrl Pts',(60.440286369022,250.069110537011,17.9175645046006)) ;
#108683=CARTESIAN_POINT('Ctrl Pts',(60.4402651077865,250.067736058266,17.9170763684254)) ;
#108684=CARTESIAN_POINT('Ctrl Pts',(60.4402651077865,250.066361548099,17.9165880896073)) ;
#108685=CARTESIAN_POINT('Ctrl Pts',(60.4402651077865,249.898460333955,18.4333348922483)) ;
#108686=CARTESIAN_POINT('Ctrl Pts',(60.4402651077865,249.899175309841,18.433001862636)) ;
#108687=CARTESIAN_POINT('Ctrl Pts',(60.4402684378921,249.899890317951,18.4326688888986)) ;
#108688=CARTESIAN_POINT('Ctrl Pts',(60.4404467789389,249.919031290693,18.423756982537)) ;
#108689=CARTESIAN_POINT('Ctrl Pts',(60.4428319502748,249.937545285356,18.4151851106646)) ;
#108690=CARTESIAN_POINT('Ctrl Pts',(60.4520052987553,249.972680889962,18.3990026749411)) ;
#108691=CARTESIAN_POINT('Ctrl Pts',(60.4586423249848,249.989505329671,18.3912950523216)) ;
#108692=CARTESIAN_POINT('Ctrl Pts',(60.4774783235664,250.022559616024,18.3762187794687)) ;
#108693=CARTESIAN_POINT('Ctrl Pts',(60.4902886559451,250.038671895832,18.3689119713107)) ;
#108694=CARTESIAN_POINT('Ctrl Pts',(60.5183067650571,250.062085528376,18.3583294709921)) ;
#108695=CARTESIAN_POINT('Ctrl Pts',(60.5322233323112,250.070462900348,18.3545568129842)) ;
#108696=CARTESIAN_POINT('Ctrl Pts',(60.5612197979218,250.08106143577,18.3497888860605)) ;
#108697=CARTESIAN_POINT('Ctrl Pts',(60.5755858845328,250.083712025826,18.3485990065702)) ;
#108698=CARTESIAN_POINT('Ctrl Pts',(60.5902651077866,250.083712025826,18.3485990065702)) ;
#108699=CARTESIAN_POINT('Origin',(60.5902651077865,248.389748311783,20.2826839799233)) ;
#108700=CARTESIAN_POINT('Ctrl Pts',(60.4402651077865,248.389748311783,18.0836729796702)) ;
#108701=CARTESIAN_POINT('Ctrl Pts',(60.4402651077865,248.390325382447,18.0831353099888)) ;
#108702=CARTESIAN_POINT('Ctrl Pts',(60.4402684378921,248.390902501024,18.0825976834901)) ;
#108703=CARTESIAN_POINT('Ctrl Pts',(60.4404467789386,248.406352717361,18.0682070710062)) ;
#108704=CARTESIAN_POINT('Ctrl Pts',(60.4428319502743,248.421311718545,18.0543335974202)) ;
#108705=CARTESIAN_POINT('Ctrl Pts',(60.4520052987547,248.449727016612,18.0280856875444)) ;
#108706=CARTESIAN_POINT('Ctrl Pts',(60.4586423249843,248.463346223255,18.0155562650353)) ;
#108707=CARTESIAN_POINT('Ctrl Pts',(60.4774783235664,248.490123893161,17.9910035412764)) ;
#108708=CARTESIAN_POINT('Ctrl Pts',(60.4902886559451,248.503189653969,17.9790753854858)) ;
#108709=CARTESIAN_POINT('Ctrl Pts',(60.5183067650571,248.522187169328,17.9617756192429)) ;
#108710=CARTESIAN_POINT('Ctrl Pts',(60.5322233323112,248.528988708093,17.9555988579533)) ;
#108711=CARTESIAN_POINT('Ctrl Pts',(60.5612197979217,248.537595143822,17.9477891624225)) ;
#108712=CARTESIAN_POINT('Ctrl Pts',(60.5755858845327,248.539748311783,17.9458384424072)) ;
#108713=CARTESIAN_POINT('Ctrl Pts',(60.5902651077865,248.539748311783,17.9458384424072)) ;
#108714=CARTESIAN_POINT('Ctrl Pts',(60.5902651077865,248.539748311783,17.5440476162869)) ;
#108715=CARTESIAN_POINT('Ctrl Pts',(60.5707376338848,248.539748311783,17.5440476162869)) ;
#108716=CARTESIAN_POINT('Ctrl Pts',(60.5513971100606,248.535935086915,17.5439613828925)) ;
#108717=CARTESIAN_POINT('Ctrl Pts',(60.5333315664697,248.528523568487,17.5437909270112)) ;
#108718=CARTESIAN_POINT('Ctrl Pts',(60.5152637963993,248.521111136629,17.5436204501222)) ;
#108719=CARTESIAN_POINT('Ctrl Pts',(60.4988172216937,248.510241459345,17.5433688659334)) ;
#108720=CARTESIAN_POINT('Ctrl Pts',(60.4849165768423,248.496526994243,17.5430425837125)) ;
#108721=CARTESIAN_POINT('Ctrl Pts',(60.4710122117664,248.482808858743,17.5427162141689)) ;
#108722=CARTESIAN_POINT('Ctrl Pts',(60.4599211853135,248.466506940072,17.5423210916655)) ;
#108723=CARTESIAN_POINT('Ctrl Pts',(60.4522665395979,248.44853942657,17.5418692158129)) ;
#108724=CARTESIAN_POINT('Ctrl Pts',(60.4449239452532,248.431304381614,17.5414357612543)) ;
#108725=CARTESIAN_POINT('Ctrl Pts',(60.440875076062,248.41284621875,17.5409575471862)) ;
#108726=CARTESIAN_POINT('Ctrl Pts',(60.4403288850238,248.394121994861,17.5404517504227)) ;
#108727=CARTESIAN_POINT('Ctrl Pts',(60.440286369022,248.392664484427,17.5404123787476)) ;
#108728=CARTESIAN_POINT('Ctrl Pts',(60.4402651077865,248.391206435086,17.5403728709489)) ;
#108729=CARTESIAN_POINT('Ctrl Pts',(60.4402651077865,248.389748311783,17.5403332371977)) ;
#108730=CARTESIAN_POINT('Origin',(60.5902651077865,248.040265107786,23.0213203435596)) ;
#108731=CARTESIAN_POINT('Ctrl Pts',(60.4402651077865,249.233703776962,18.2173423936815)) ;
#108732=CARTESIAN_POINT('Ctrl Pts',(60.4402651077865,249.233321099216,18.2166527147863)) ;
#108733=CARTESIAN_POINT('Ctrl Pts',(60.440268437892,249.232938362558,18.2159630621546)) ;
#108734=CARTESIAN_POINT('Ctrl Pts',(60.4404467789383,249.22269127745,18.1975023969641)) ;
#108735=CARTESIAN_POINT('Ctrl Pts',(60.4428319502738,249.212751561005,18.1796853539209)) ;
#108736=CARTESIAN_POINT('Ctrl Pts',(60.4520052987543,249.193838056834,18.1459412981901)) ;
#108737=CARTESIAN_POINT('Ctrl Pts',(60.4586423249841,249.184757226094,18.1298165429642)) ;
#108738=CARTESIAN_POINT('Ctrl Pts',(60.4774783235664,249.166877357539,18.0981907599697)) ;
#108739=CARTESIAN_POINT('Ctrl Pts',(60.4902886559451,249.158137083433,18.0828088675435)) ;
#108740=CARTESIAN_POINT('Ctrl Pts',(60.5183067650571,249.145415294424,18.0604852570307)) ;
#108741=CARTESIAN_POINT('Ctrl Pts',(60.5322233323112,249.14085537087,18.0525090168905)) ;
#108742=CARTESIAN_POINT('Ctrl Pts',(60.5612197979217,249.135083492728,18.0424220201645)) ;
#108743=CARTESIAN_POINT('Ctrl Pts',(60.5755858845327,249.133638513944,18.0399014096908)) ;
#108744=CARTESIAN_POINT('Ctrl Pts',(60.5902651077865,249.133638513944,18.0399014096908)) ;
#108745=CARTESIAN_POINT('Origin',(60.5902651077865,248.445501341285,20.6431800539285)) ;
#108746=CARTESIAN_POINT('Ctrl Pts',(60.4402651077865,249.401604991106,17.700595591041)) ;
#108747=CARTESIAN_POINT('Ctrl Pts',(60.4402651077865,249.400205985933,17.7001827000975)) ;
#108748=CARTESIAN_POINT('Ctrl Pts',(60.440286369022,249.398807090025,17.699769712223)) ;
#108749=CARTESIAN_POINT('Ctrl Pts',(60.4403288850239,249.397408748713,17.6993567614174)) ;
#108750=CARTESIAN_POINT('Ctrl Pts',(60.4408750760622,249.379444653775,17.6940516993328)) ;
#108751=CARTESIAN_POINT('Ctrl Pts',(60.4449239452535,249.361742121431,17.6888026219299)) ;
#108752=CARTESIAN_POINT('Ctrl Pts',(60.4522665395983,249.345216674792,17.6838889399227)) ;
#108753=CARTESIAN_POINT('Ctrl Pts',(60.4599211853141,249.327988916676,17.6787664323785)) ;
#108754=CARTESIAN_POINT('Ctrl Pts',(60.4710122117672,249.312362771127,17.6741046463007)) ;
#108755=CARTESIAN_POINT('Ctrl Pts',(60.4849165768428,249.299215195234,17.6701759051814)) ;
#108756=CARTESIAN_POINT('Ctrl Pts',(60.4988172216939,249.28607113708,17.6662482152284)) ;
#108757=CARTESIAN_POINT('Ctrl Pts',(60.5152637963996,249.275655715879,17.6631285710071)) ;
#108758=CARTESIAN_POINT('Ctrl Pts',(60.5333315664699,249.268553394004,17.6610001367497)) ;
#108759=CARTESIAN_POINT('Ctrl Pts',(60.5513971100607,249.261451947343,17.6588719647779)) ;
#108760=CARTESIAN_POINT('Ctrl Pts',(60.5707376338848,249.2577987074,17.6577756263218)) ;
#108761=CARTESIAN_POINT('Ctrl Pts',(60.5902651077865,249.2577987074,17.6577756263218)) ;
#108762=CARTESIAN_POINT('Origin',(60.5902651077865,249.739858576849,17.7905095039363)) ;
#108763=CARTESIAN_POINT('Origin',(60.5902651077865,248.040265107786,17.5213203435596)) ;
#108764=CARTESIAN_POINT('Origin',(60.5902651077865,248.040265107786,23.0213203435596)) ;
#108765=CARTESIAN_POINT('',(60.5902651077865,250.619468117123,18.6215803698081)) ;
#108766=CARTESIAN_POINT('Origin',(60.5902651077865,248.040265107786,23.0213203435596)) ;
#108767=CARTESIAN_POINT('Ctrl Pts',(60.4402651077865,250.65980355802,18.8212586407095)) ;
#108768=CARTESIAN_POINT('Ctrl Pts',(60.4402651077865,250.659652732354,18.8204844631737)) ;
#108769=CARTESIAN_POINT('Ctrl Pts',(60.4402684378921,250.659501842545,18.8197102924112)) ;
#108770=CARTESIAN_POINT('Ctrl Pts',(60.4404467789386,250.655460944751,18.7989866330445)) ;
#108771=CARTESIAN_POINT('Ctrl Pts',(60.4428319502743,250.651513481746,18.7789700768574)) ;
#108772=CARTESIAN_POINT('Ctrl Pts',(60.4520052987548,250.643953157039,18.7410329785579)) ;
#108773=CARTESIAN_POINT('Ctrl Pts',(60.4586423249844,250.640299597185,18.7228912940054)) ;
#108774=CARTESIAN_POINT('Ctrl Pts',(60.4774783235664,250.633067736091,18.6872882037655)) ;
#108775=CARTESIAN_POINT('Ctrl Pts',(60.4902886559451,250.629508507613,18.6699582615064)) ;
#108776=CARTESIAN_POINT('Ctrl Pts',(60.5183067650571,250.624307742302,18.6447959972585)) ;
#108777=CARTESIAN_POINT('Ctrl Pts',(60.5322233323112,250.622435791047,18.6358010482263)) ;
#108778=CARTESIAN_POINT('Ctrl Pts',(60.5612197979218,250.620063462139,18.6244241358249)) ;
#108779=CARTESIAN_POINT('Ctrl Pts',(60.5755858845328,250.619468117123,18.6215803698081)) ;
#108780=CARTESIAN_POINT('Ctrl Pts',(60.5902651077865,250.619468117123,18.6215803698081)) ;
#108781=CARTESIAN_POINT('Origin',(60.5902651077865,249.160553432798,20.8847994073294)) ;
#108782=CARTESIAN_POINT('',(60.5902651077865,250.855634839223,18.2965247632928)) ;
#108783=CARTESIAN_POINT('',(60.5902651077865,249.039200883641,20.7966316194855)) ;
#108784=CARTESIAN_POINT('Ctrl Pts',(60.4402651077865,250.979170645629,18.3816875553299)) ;
#108785=CARTESIAN_POINT('Ctrl Pts',(60.4402651077865,250.977967702962,18.3808625563341)) ;
#108786=CARTESIAN_POINT('Ctrl Pts',(60.440286369022,250.976764894165,18.3800374989159)) ;
#108787=CARTESIAN_POINT('Ctrl Pts',(60.4403288850239,250.975562601365,18.3792126481319)) ;
#108788=CARTESIAN_POINT('Ctrl Pts',(60.4408750760622,250.960117086155,18.368616023642)) ;
#108789=CARTESIAN_POINT('Ctrl Pts',(60.4449239452534,250.944903031537,18.3581534710365)) ;
#108790=CARTESIAN_POINT('Ctrl Pts',(60.4522665395982,250.930704809071,18.3483736378934)) ;
#108791=CARTESIAN_POINT('Ctrl Pts',(60.459921185314,250.915903179339,18.3381781736808)) ;
#108792=CARTESIAN_POINT('Ctrl Pts',(60.4710122117671,250.902482402912,18.3289158071227)) ;
#108793=CARTESIAN_POINT('Ctrl Pts',(60.4849165768428,250.891192362958,18.3211165278944)) ;
#108794=CARTESIAN_POINT('Ctrl Pts',(60.498817221694,250.879905343744,18.3133193354258)) ;
#108795=CARTESIAN_POINT('Ctrl Pts',(60.5152637963998,250.870963712621,18.3071338353064)) ;
#108796=CARTESIAN_POINT('Ctrl Pts',(60.5333315664701,250.864866725478,18.3029148358775)) ;
#108797=CARTESIAN_POINT('Ctrl Pts',(60.5513971100608,250.858770489662,18.2986963563531)) ;
#108798=CARTESIAN_POINT('Ctrl Pts',(60.5707376338847,250.855634839223,18.2965247632931)) ;
#108799=CARTESIAN_POINT('Ctrl Pts',(60.5902651077865,250.855634839223,18.2965247632931)) ;
#108800=CARTESIAN_POINT('Origin',(60.5902651077865,251.273083995395,18.5717268744974)) ;
#108801=CARTESIAN_POINT('Origin',(60.5902651077865,251.273083995395,18.5717268744974)) ;
#108802=CARTESIAN_POINT('Origin',(60.5902651077865,246.340671638724,17.7905095039363)) ;
#108803=CARTESIAN_POINT('Origin',(60.5902651077865,248.040265107786,23.0213203435596)) ;
#108804=CARTESIAN_POINT('',(60.5902651077865,251.852827359384,19.6339365333471)) ;
#108805=CARTESIAN_POINT('Origin',(60.5902651077865,248.040265107786,23.0213203435596)) ;
#108806=CARTESIAN_POINT('Ctrl Pts',(60.4402651077865,251.829484664171,19.836306190763)) ;
#108807=CARTESIAN_POINT('Ctrl Pts',(60.4402651077865,251.829580454454,19.8355232964805)) ;
#108808=CARTESIAN_POINT('Ctrl Pts',(60.440268437892,251.829676181639,19.8347403888179)) ;
#108809=CARTESIAN_POINT('Ctrl Pts',(60.4404467789383,251.832237022391,19.8137823114479)) ;
#108810=CARTESIAN_POINT('Ctrl Pts',(60.4428319502738,251.834668218008,19.7935256020966)) ;
#108811=CARTESIAN_POINT('Ctrl Pts',(60.4520052987543,251.839201130021,19.7551090087302)) ;
#108812=CARTESIAN_POINT('Ctrl Pts',(60.4586423249841,251.841332476948,19.7367262293345)) ;
#108813=CARTESIAN_POINT('Ctrl Pts',(60.4774783235663,251.845456528266,19.7006309103821)) ;
#108814=CARTESIAN_POINT('Ctrl Pts',(60.490288655945,251.847426747499,19.6830492937831)) ;
#108815=CARTESIAN_POINT('Ctrl Pts',(60.5183067650572,251.85025609303,19.6575114335403)) ;
#108816=CARTESIAN_POINT('Ctrl Pts',(60.5322233323113,251.851255353705,19.648378263899)) ;
#108817=CARTESIAN_POINT('Ctrl Pts',(60.5612197979218,251.852514794114,19.6368250872756)) ;
#108818=CARTESIAN_POINT('Ctrl Pts',(60.5755858845328,251.852827359384,19.6339365333471)) ;
#108819=CARTESIAN_POINT('Ctrl Pts',(60.5902651077865,251.852827359384,19.633936533347)) ;
#108820=CARTESIAN_POINT('Origin',(60.5902651077865,249.765943897551,21.3355563159851)) ;
#108821=CARTESIAN_POINT('',(60.5902651077865,252.1778829659,19.3977698112471)) ;
#108822=CARTESIAN_POINT('',(60.5902651077865,249.677776109707,21.2142037668289)) ;
#108823=CARTESIAN_POINT('Ctrl Pts',(60.4402651077865,252.26905574955,19.5169391031532)) ;
#108824=CARTESIAN_POINT('Ctrl Pts',(60.4402651077865,252.268166621798,19.5157827527552)) ;
#108825=CARTESIAN_POINT('Ctrl Pts',(60.440286369022,252.267277639418,19.5146263881606)) ;
#108826=CARTESIAN_POINT('Ctrl Pts',(60.4403288850239,252.266389083925,19.5134703795409)) ;
#108827=CARTESIAN_POINT('Ctrl Pts',(60.4408750760621,252.254974063079,19.4986194640923)) ;
#108828=CARTESIAN_POINT('Ctrl Pts',(60.4449239452531,252.243737743862,19.4839675838214)) ;
#108829=CARTESIAN_POINT('Ctrl Pts',(60.4522665395981,252.23325656651,19.4702789177502)) ;
#108830=CARTESIAN_POINT('Ctrl Pts',(60.4599211853138,252.222329951808,19.4560084999423)) ;
#108831=CARTESIAN_POINT('Ctrl Pts',(60.4710122117667,252.21242826361,19.4430522178763)) ;
#108832=CARTESIAN_POINT('Ctrl Pts',(60.4849165768426,252.204100907367,19.4321458483306)) ;
#108833=CARTESIAN_POINT('Ctrl Pts',(60.498817221694,252.195775779175,19.4212423968717)) ;
#108834=CARTESIAN_POINT('Ctrl Pts',(60.5152637963995,252.189183207286,19.4125965207019)) ;
#108835=CARTESIAN_POINT('Ctrl Pts',(60.5333315664699,252.184688370457,19.4066999411606)) ;
#108836=CARTESIAN_POINT('Ctrl Pts',(60.5513971100608,252.180194087523,19.4008040882511)) ;
#108837=CARTESIAN_POINT('Ctrl Pts',(60.5707376338848,252.177882965899,19.3977698112477)) ;
#108838=CARTESIAN_POINT('Ctrl Pts',(60.5902651077865,252.177882965899,19.3977698112476)) ;
#108839=CARTESIAN_POINT('Origin',(60.5902651077865,252.489858576849,19.788501455951)) ;
#108840=CARTESIAN_POINT('Origin',(60.5902651077865,252.489858576849,19.788501455951)) ;
#108841=CARTESIAN_POINT('Origin',(60.5902651077865,244.807446220178,18.5717268744974)) ;
#108842=CARTESIAN_POINT('Origin',(60.5902651077865,248.040265107786,23.0213203435596)) ;
#108843=CARTESIAN_POINT('',(60.5902651077865,252.712986444776,20.9778734255204)) ;
#108844=CARTESIAN_POINT('Origin',(60.5902651077865,248.040265107786,23.0213203435596)) ;
#108845=CARTESIAN_POINT('Ctrl Pts',(60.4402651077865,252.628250559098,21.1631251173908)) ;
#108846=CARTESIAN_POINT('Ctrl Pts',(60.4402651077865,252.628583588709,21.162410141506)) ;
#108847=CARTESIAN_POINT('Ctrl Pts',(60.4402684378921,252.628916562446,21.1616951333976)) ;
#108848=CARTESIAN_POINT('Ctrl Pts',(60.4404467789386,252.637828468808,21.1425541606572)) ;
#108849=CARTESIAN_POINT('Ctrl Pts',(60.4428319502743,252.64640034068,21.1240401659929)) ;
#108850=CARTESIAN_POINT('Ctrl Pts',(60.4520052987547,252.662582776404,21.0889045613858)) ;
#108851=CARTESIAN_POINT('Ctrl Pts',(60.4586423249843,252.670290399024,21.0720801216756)) ;
#108852=CARTESIAN_POINT('Ctrl Pts',(60.4774783235664,252.685366671877,21.0390258353215)) ;
#108853=CARTESIAN_POINT('Ctrl Pts',(60.4902886559451,252.692673480035,21.0229135555138)) ;
#108854=CARTESIAN_POINT('Ctrl Pts',(60.5183067650571,252.703255980354,20.9994999229698)) ;
#108855=CARTESIAN_POINT('Ctrl Pts',(60.5322233323112,252.707028638362,20.9911225509982)) ;
#108856=CARTESIAN_POINT('Ctrl Pts',(60.5612197979218,252.711796565285,20.9805240155764)) ;
#108857=CARTESIAN_POINT('Ctrl Pts',(60.5755858845328,252.712986444776,20.9778734255204)) ;
#108858=CARTESIAN_POINT('Ctrl Pts',(60.5902651077866,252.712986444776,20.9778734255204)) ;
#108859=CARTESIAN_POINT('Origin',(60.5902651077865,250.202412898851,21.9513275530686)) ;
#108860=CARTESIAN_POINT('',(60.5902651077865,253.095112228145,20.8537132320653)) ;
#108861=CARTESIAN_POINT('',(60.5902651077865,250.156060349694,21.8086690756243)) ;
#108862=CARTESIAN_POINT('Ctrl Pts',(60.4402651077865,253.144997361738,20.9952239032473)) ;
#108863=CARTESIAN_POINT('Ctrl Pts',(60.4402651077865,253.14450908292,20.9938493930806)) ;
#108864=CARTESIAN_POINT('Ctrl Pts',(60.440286369022,253.144020946746,20.9924749143347)) ;
#108865=CARTESIAN_POINT('Ctrl Pts',(60.4403288850239,253.143533106564,20.9911009060563)) ;
#108866=CARTESIAN_POINT('Ctrl Pts',(60.4408750760621,253.137265961862,20.9734494107126)) ;
#108867=CARTESIAN_POINT('Ctrl Pts',(60.4449239452531,253.131107267255,20.9560424309125)) ;
#108868=CARTESIAN_POINT('Ctrl Pts',(60.4522665395981,253.125369105682,20.9397848739233)) ;
#108869=CARTESIAN_POINT('Ctrl Pts',(60.4599211853139,253.119387079188,20.9228363904431)) ;
#108870=CARTESIAN_POINT('Ctrl Pts',(60.4710122117669,253.113973725445,20.9074544440316)) ;
#108871=CARTESIAN_POINT('Ctrl Pts',(60.4849165768427,253.109424192564,20.8945085756088)) ;
#108872=CARTESIAN_POINT('Ctrl Pts',(60.4988172216941,253.104875876946,20.8815661709571)) ;
#108873=CARTESIAN_POINT('Ctrl Pts',(60.5152637963996,253.101277691159,20.8713062373365)) ;
#108874=CARTESIAN_POINT('Ctrl Pts',(60.53333156647,253.098824990589,20.8643092759729)) ;
#108875=CARTESIAN_POINT('Ctrl Pts',(60.5513971100609,253.096372592264,20.8573131768402)) ;
#108876=CARTESIAN_POINT('Ctrl Pts',(60.5707376338848,253.095112228145,20.8537132320655)) ;
#108877=CARTESIAN_POINT('Ctrl Pts',(60.5902651077865,253.095112228145,20.8537132320655)) ;
#108878=CARTESIAN_POINT('Origin',(60.5902651077865,253.27107594741,21.3217268744974)) ;
#108879=CARTESIAN_POINT('Origin',(60.5902651077865,253.27107594741,21.3217268744974)) ;
#108880=CARTESIAN_POINT('Origin',(60.5902651077865,243.590671638724,19.788501455951)) ;
#108881=CARTESIAN_POINT('Origin',(60.5902651077865,248.040265107786,23.0213203435596)) ;
#108882=CARTESIAN_POINT('',(60.5902651077865,253.115747008939,22.5218371395634)) ;
#108883=CARTESIAN_POINT('Origin',(60.5902651077865,248.040265107786,23.0213203435596)) ;
#108884=CARTESIAN_POINT('Ctrl Pts',(60.4402651077865,252.977912471676,22.6718371395634)) ;
#108885=CARTESIAN_POINT('Ctrl Pts',(60.4402651077865,252.978450141357,22.6712600688988)) ;
#108886=CARTESIAN_POINT('Ctrl Pts',(60.4402684378921,252.978987767856,22.6706829503216)) ;
#108887=CARTESIAN_POINT('Ctrl Pts',(60.4404467789386,252.99337838034,22.655232733985)) ;
#108888=CARTESIAN_POINT('Ctrl Pts',(60.4428319502743,253.007251853926,22.6402737328004)) ;
#108889=CARTESIAN_POINT('Ctrl Pts',(60.4520052987548,253.033499763802,22.611858434734)) ;
#108890=CARTESIAN_POINT('Ctrl Pts',(60.4586423249844,253.046029186311,22.5982392280904)) ;
#108891=CARTESIAN_POINT('Ctrl Pts',(60.4774783235664,253.07058191007,22.5714615581854)) ;
#108892=CARTESIAN_POINT('Ctrl Pts',(60.4902886559451,253.08251006586,22.5583957973774)) ;
#108893=CARTESIAN_POINT('Ctrl Pts',(60.5183067650572,253.099809832103,22.5393982820177)) ;
#108894=CARTESIAN_POINT('Ctrl Pts',(60.5322233323113,253.105986593393,22.5325967432531)) ;
#108895=CARTESIAN_POINT('Ctrl Pts',(60.5612197979217,253.113796288923,22.5239903075244)) ;
#108896=CARTESIAN_POINT('Ctrl Pts',(60.5755858845327,253.115747008939,22.5218371395634)) ;
#108897=CARTESIAN_POINT('Ctrl Pts',(60.5902651077865,253.115747008939,22.5218371395634)) ;
#108898=CARTESIAN_POINT('Origin',(60.5902651077865,250.427235809792,22.6718371395634)) ;
#108899=CARTESIAN_POINT('',(60.5902651077865,253.517537835059,22.5218371395634)) ;
#108900=CARTESIAN_POINT('',(60.5902651077865,250.427235809792,22.5218371395634)) ;
#108901=CARTESIAN_POINT('Ctrl Pts',(60.4402651077865,253.521252214148,22.6718371395634)) ;
#108902=CARTESIAN_POINT('Ctrl Pts',(60.4402651077865,253.521212580397,22.6703790162596)) ;
#108903=CARTESIAN_POINT('Ctrl Pts',(60.440286369022,253.521173072598,22.6689209669186)) ;
#108904=CARTESIAN_POINT('Ctrl Pts',(60.4403288850239,253.521133700923,22.667463456485)) ;
#108905=CARTESIAN_POINT('Ctrl Pts',(60.4408750760621,253.52062790416,22.6487392325954)) ;
#108906=CARTESIAN_POINT('Ctrl Pts',(60.4449239452532,253.520149690092,22.6302810697323)) ;
#108907=CARTESIAN_POINT('Ctrl Pts',(60.452266539598,253.519716235534,22.6130460247761)) ;
#108908=CARTESIAN_POINT('Ctrl Pts',(60.4599211853139,253.519264359681,22.5950785112735)) ;
#108909=CARTESIAN_POINT('Ctrl Pts',(60.4710122117668,253.518869237177,22.5787765926025)) ;
#108910=CARTESIAN_POINT('Ctrl Pts',(60.4849165768426,253.518542867634,22.5650584571031)) ;
#108911=CARTESIAN_POINT('Ctrl Pts',(60.4988172216939,253.518216585413,22.5513439920009)) ;
#108912=CARTESIAN_POINT('Ctrl Pts',(60.5152637963994,253.517965001224,22.5404743147172)) ;
#108913=CARTESIAN_POINT('Ctrl Pts',(60.5333315664698,253.517794524335,22.5330618828598)) ;
#108914=CARTESIAN_POINT('Ctrl Pts',(60.5513971100607,253.517624068453,22.5256503644316)) ;
#108915=CARTESIAN_POINT('Ctrl Pts',(60.5707376338847,253.517537835059,22.5218371395634)) ;
#108916=CARTESIAN_POINT('Ctrl Pts',(60.5902651077865,253.517537835059,22.5218371395634)) ;
#108917=CARTESIAN_POINT('Origin',(60.5902651077865,253.540265107786,23.0213203435596)) ;
#108918=CARTESIAN_POINT('Origin',(60.5902651077865,253.540265107786,23.0213203435596)) ;
#108919=CARTESIAN_POINT('Origin',(60.5902651077865,242.809454268163,21.3217268744974)) ;
#108920=CARTESIAN_POINT('Origin',(60.5902651077865,248.040265107786,23.0213203435596)) ;
#108921=CARTESIAN_POINT('',(60.5902651077865,253.021684041655,24.1146937497175)) ;
#108922=CARTESIAN_POINT('Origin',(60.5902651077865,248.040265107786,23.0213203435596)) ;
#108923=CARTESIAN_POINT('Ctrl Pts',(60.4402651077865,252.844243057664,24.2147590127358)) ;
#108924=CARTESIAN_POINT('Ctrl Pts',(60.4402651077865,252.844932736563,24.2143763349877)) ;
#108925=CARTESIAN_POINT('Ctrl Pts',(60.440268437892,252.845622389192,24.213993598331)) ;
#108926=CARTESIAN_POINT('Ctrl Pts',(60.4404467789386,252.864083054386,24.2037465132206)) ;
#108927=CARTESIAN_POINT('Ctrl Pts',(60.4428319502744,252.881900097428,24.1938067967769)) ;
#108928=CARTESIAN_POINT('Ctrl Pts',(60.4520052987548,252.915644153157,24.1748932926068)) ;
#108929=CARTESIAN_POINT('Ctrl Pts',(60.4586423249845,252.931768908382,24.1658124618668)) ;
#108930=CARTESIAN_POINT('Ctrl Pts',(60.4774783235665,252.963394691376,24.1479325933121)) ;
#108931=CARTESIAN_POINT('Ctrl Pts',(60.4902886559452,252.978776583803,24.1391923192062)) ;
#108932=CARTESIAN_POINT('Ctrl Pts',(60.5183067650572,253.001100194315,24.1264705301978)) ;
#108933=CARTESIAN_POINT('Ctrl Pts',(60.5322233323113,253.009076434455,24.1219106066435)) ;
#108934=CARTESIAN_POINT('Ctrl Pts',(60.5612197979217,253.019163431181,24.1161387285016)) ;
#108935=CARTESIAN_POINT('Ctrl Pts',(60.5755858845327,253.021684041655,24.1146937497175)) ;
#108936=CARTESIAN_POINT('Ctrl Pts',(60.5902651077866,253.021684041655,24.1146937497175)) ;
#108937=CARTESIAN_POINT('Origin',(60.5902651077865,250.418405397417,23.426556577058)) ;
#108938=CARTESIAN_POINT('',(60.5902651077865,253.403809825024,24.2388539431727)) ;
#108939=CARTESIAN_POINT('',(60.5902651077865,250.464757946574,23.2838980996137)) ;
#108940=CARTESIAN_POINT('Ctrl Pts',(60.4402651077865,253.360989860305,24.3826602268791)) ;
#108941=CARTESIAN_POINT('Ctrl Pts',(60.4402651077865,253.361402751249,24.3812612217063)) ;
#108942=CARTESIAN_POINT('Ctrl Pts',(60.440286369022,253.361815739121,24.3798623257983)) ;
#108943=CARTESIAN_POINT('Ctrl Pts',(60.4403288850239,253.362228689928,24.378463984486)) ;
#108944=CARTESIAN_POINT('Ctrl Pts',(60.4408750760622,253.367533752024,24.3604998895503)) ;
#108945=CARTESIAN_POINT('Ctrl Pts',(60.4449239452534,253.372782829414,24.3427973572039)) ;
#108946=CARTESIAN_POINT('Ctrl Pts',(60.4522665395982,253.377696511422,24.3262719105652)) ;
#108947=CARTESIAN_POINT('Ctrl Pts',(60.459921185314,253.382819018967,24.3090441524494)) ;
#108948=CARTESIAN_POINT('Ctrl Pts',(60.4710122117669,253.387480805045,24.2934180069006)) ;
#108949=CARTESIAN_POINT('Ctrl Pts',(60.4849165768428,253.391409546165,24.2802704310071)) ;
#108950=CARTESIAN_POINT('Ctrl Pts',(60.4988172216941,253.395337236118,24.2671263728531)) ;
#108951=CARTESIAN_POINT('Ctrl Pts',(60.5152637963996,253.39845688034,24.2567109516526)) ;
#108952=CARTESIAN_POINT('Ctrl Pts',(60.53333156647,253.400585314597,24.2496086297771)) ;
#108953=CARTESIAN_POINT('Ctrl Pts',(60.5513971100607,253.402713486568,24.2425071831161)) ;
#108954=CARTESIAN_POINT('Ctrl Pts',(60.5707376338847,253.403809825025,24.238853943173)) ;
#108955=CARTESIAN_POINT('Ctrl Pts',(60.5902651077865,253.403809825025,24.238853943173)) ;
#108956=CARTESIAN_POINT('Origin',(60.5902651077865,253.27107594741,24.7209138126218)) ;
#108957=CARTESIAN_POINT('Origin',(60.5902651077865,253.27107594741,24.7209138126218)) ;
#108958=CARTESIAN_POINT('Origin',(60.5902651077865,242.540265107786,23.0213203435596)) ;
#108959=CARTESIAN_POINT('Origin',(60.5902651077865,248.040265107786,23.0213203435596)) ;
#108960=CARTESIAN_POINT('',(60.5902651077865,252.440005081538,25.6005233528965)) ;
#108961=CARTESIAN_POINT('Origin',(60.5902651077865,248.040265107786,23.0213203435596)) ;
#108962=CARTESIAN_POINT('Ctrl Pts',(60.4402651077865,252.240326810636,25.6408587937931)) ;
#108963=CARTESIAN_POINT('Ctrl Pts',(60.4402651077865,252.241100988174,25.6407079681274)) ;
#108964=CARTESIAN_POINT('Ctrl Pts',(60.440268437892,252.241875158933,25.6405570783186)) ;
#108965=CARTESIAN_POINT('Ctrl Pts',(60.4404467789386,252.262598818302,25.6365161805241)) ;
#108966=CARTESIAN_POINT('Ctrl Pts',(60.4428319502744,252.282615374489,25.6325687175193)) ;
#108967=CARTESIAN_POINT('Ctrl Pts',(60.4520052987548,252.320552472788,25.6250083928119)) ;
#108968=CARTESIAN_POINT('Ctrl Pts',(60.4586423249844,252.338694157341,25.621354832958)) ;
#108969=CARTESIAN_POINT('Ctrl Pts',(60.4774783235665,252.374297247581,25.6141229718641)) ;
#108970=CARTESIAN_POINT('Ctrl Pts',(60.4902886559452,252.39162718984,25.6105637433868)) ;
#108971=CARTESIAN_POINT('Ctrl Pts',(60.5183067650571,252.416789454087,25.6053629780756)) ;
#108972=CARTESIAN_POINT('Ctrl Pts',(60.5322233323112,252.42578440312,25.6034910268201)) ;
#108973=CARTESIAN_POINT('Ctrl Pts',(60.5612197979217,252.437161315521,25.6011186979124)) ;
#108974=CARTESIAN_POINT('Ctrl Pts',(60.5755858845327,252.440005081538,25.6005233528966)) ;
#108975=CARTESIAN_POINT('Ctrl Pts',(60.5902651077865,252.440005081538,25.6005233528966)) ;
#108976=CARTESIAN_POINT('Origin',(60.5902651077865,250.176786044017,24.1416086685709)) ;
#108977=CARTESIAN_POINT('',(60.5902651077865,252.765060688053,25.8366900749965)) ;
#108978=CARTESIAN_POINT('',(60.5902651077865,250.26495383186,24.0202561194147)) ;
#108979=CARTESIAN_POINT('Ctrl Pts',(60.4402651077865,252.679897896016,25.9602258814029)) ;
#108980=CARTESIAN_POINT('Ctrl Pts',(60.4402651077865,252.680722895012,25.9590229387354)) ;
#108981=CARTESIAN_POINT('Ctrl Pts',(60.440286369022,252.681547952429,25.9578201299378)) ;
#108982=CARTESIAN_POINT('Ctrl Pts',(60.4403288850239,252.682372803214,25.9566178371377)) ;
#108983=CARTESIAN_POINT('Ctrl Pts',(60.4408750760621,252.692969427709,25.9411723219306)) ;
#108984=CARTESIAN_POINT('Ctrl Pts',(60.4449239452532,252.703431980308,25.9259582673091)) ;
#108985=CARTESIAN_POINT('Ctrl Pts',(60.452266539598,252.713211813452,25.911760044844)) ;
#108986=CARTESIAN_POINT('Ctrl Pts',(60.4599211853139,252.723407277665,25.8969584151117)) ;
#108987=CARTESIAN_POINT('Ctrl Pts',(60.4710122117667,252.732669644223,25.8835376386852)) ;
#108988=CARTESIAN_POINT('Ctrl Pts',(60.4849165768426,252.740468923451,25.8722475987305)) ;
#108989=CARTESIAN_POINT('Ctrl Pts',(60.4988172216939,252.74826611592,25.8609605795167)) ;
#108990=CARTESIAN_POINT('Ctrl Pts',(60.5152637963993,252.75445161604,25.8520189483948)) ;
#108991=CARTESIAN_POINT('Ctrl Pts',(60.5333315664698,252.758670615469,25.8459219612514)) ;
#108992=CARTESIAN_POINT('Ctrl Pts',(60.5513971100607,252.762889094994,25.8398257254357)) ;
#108993=CARTESIAN_POINT('Ctrl Pts',(60.5707376338847,252.765060688054,25.8366900749968)) ;
#108994=CARTESIAN_POINT('Ctrl Pts',(60.5902651077865,252.765060688054,25.8366900749968)) ;
#108995=CARTESIAN_POINT('Origin',(60.5902651077865,252.489858576849,26.2541392311682)) ;
#108996=CARTESIAN_POINT('Origin',(60.5902651077865,252.489858576849,26.2541392311682)) ;
#108997=CARTESIAN_POINT('Origin',(60.5902651077865,242.809454268163,24.7209138126218)) ;
#108998=CARTESIAN_POINT('Origin',(60.5902651077865,248.040265107786,23.0213203435596)) ;
#108999=CARTESIAN_POINT('',(60.5902651077865,251.427648917999,26.8338825951576)) ;
#109000=CARTESIAN_POINT('Origin',(60.5902651077865,248.040265107786,23.0213203435596)) ;
#109001=CARTESIAN_POINT('Ctrl Pts',(60.4402651077865,251.225279260583,26.8105398999439)) ;
#109002=CARTESIAN_POINT('Ctrl Pts',(60.4402651077865,251.22606215487,26.8106356902278)) ;
#109003=CARTESIAN_POINT('Ctrl Pts',(60.440268437892,251.226845062531,26.810731417413)) ;
#109004=CARTESIAN_POINT('Ctrl Pts',(60.4404467789389,251.247803139908,26.8132922581646)) ;
#109005=CARTESIAN_POINT('Ctrl Pts',(60.4428319502749,251.268059849255,26.8157234537816)) ;
#109006=CARTESIAN_POINT('Ctrl Pts',(60.4520052987553,251.306476442619,26.8202563657949)) ;
#109007=CARTESIAN_POINT('Ctrl Pts',(60.4586423249848,251.324859222013,26.8223877127214)) ;
#109008=CARTESIAN_POINT('Ctrl Pts',(60.4774783235664,251.360954540964,26.8265117640394)) ;
#109009=CARTESIAN_POINT('Ctrl Pts',(60.4902886559451,251.378536157563,26.8284819832727)) ;
#109010=CARTESIAN_POINT('Ctrl Pts',(60.5183067650572,251.404074017806,26.8313113288033)) ;
#109011=CARTESIAN_POINT('Ctrl Pts',(60.5322233323113,251.413207187447,26.832310589478)) ;
#109012=CARTESIAN_POINT('Ctrl Pts',(60.5612197979217,251.42476036407,26.8335700298871)) ;
#109013=CARTESIAN_POINT('Ctrl Pts',(60.5755858845327,251.427648917999,26.8338825951576)) ;
#109014=CARTESIAN_POINT('Ctrl Pts',(60.5902651077866,251.427648917999,26.8338825951576)) ;
#109015=CARTESIAN_POINT('Origin',(60.5902651077865,249.726029135361,24.746999133324)) ;
#109016=CARTESIAN_POINT('',(60.5902651077865,251.663815640099,27.1589382016729)) ;
#109017=CARTESIAN_POINT('',(60.5902651077865,249.847381684517,24.6588313454802)) ;
#109018=CARTESIAN_POINT('Ctrl Pts',(60.4402651077865,251.544646348192,27.2501109853232)) ;
#109019=CARTESIAN_POINT('Ctrl Pts',(60.4402651077865,251.545802698591,27.2492218575707)) ;
#109020=CARTESIAN_POINT('Ctrl Pts',(60.440286369022,251.546959063183,27.2483328751888)) ;
#109021=CARTESIAN_POINT('Ctrl Pts',(60.4403288850239,251.548115071804,27.2474443196972)) ;
#109022=CARTESIAN_POINT('Ctrl Pts',(60.4408750760621,251.562965987268,27.2360292988668)) ;
#109023=CARTESIAN_POINT('Ctrl Pts',(60.4449239452532,251.577617867525,27.2247929796352)) ;
#109024=CARTESIAN_POINT('Ctrl Pts',(60.452266539598,251.591306533596,27.2143118022833)) ;
#109025=CARTESIAN_POINT('Ctrl Pts',(60.459921185314,251.605576951405,27.2033851875821)) ;
#109026=CARTESIAN_POINT('Ctrl Pts',(60.4710122117669,251.61853323347,27.1934834993827)) ;
#109027=CARTESIAN_POINT('Ctrl Pts',(60.4849165768426,251.629439603015,27.1851561431399)) ;
#109028=CARTESIAN_POINT('Ctrl Pts',(60.4988172216938,251.640343054474,27.1768310149481)) ;
#109029=CARTESIAN_POINT('Ctrl Pts',(60.5152637963993,251.648988930644,27.1702384430593)) ;
#109030=CARTESIAN_POINT('Ctrl Pts',(60.5333315664697,251.654885510185,27.1657436062293)) ;
#109031=CARTESIAN_POINT('Ctrl Pts',(60.5513971100606,251.660781363094,27.1612493232952)) ;
#109032=CARTESIAN_POINT('Ctrl Pts',(60.5707376338847,251.663815640098,27.1589382016717)) ;
#109033=CARTESIAN_POINT('Ctrl Pts',(60.5902651077865,251.663815640098,27.1589382016716)) ;
#109034=CARTESIAN_POINT('Origin',(60.5902651077865,251.273083995395,27.4709138126218)) ;
#109035=CARTESIAN_POINT('Origin',(60.5902651077865,251.273083995395,27.4709138126218)) ;
#109036=CARTESIAN_POINT('Origin',(60.5902651077865,243.590671638724,26.2541392311682)) ;
#109037=CARTESIAN_POINT('Origin',(60.5902651077865,248.040265107786,23.0213203435596)) ;
#109038=CARTESIAN_POINT('',(60.5902651077865,250.083712025826,27.694041680549)) ;
#109039=CARTESIAN_POINT('Origin',(60.5902651077865,248.040265107786,23.0213203435596)) ;
#109040=CARTESIAN_POINT('Ctrl Pts',(60.4402651077865,249.898460333955,27.6093057948708)) ;
#109041=CARTESIAN_POINT('Ctrl Pts',(60.4402651077865,249.89917530984,27.6096388244826)) ;
#109042=CARTESIAN_POINT('Ctrl Pts',(60.4402684378921,249.899890317948,27.6099717982194)) ;
#109043=CARTESIAN_POINT('Ctrl Pts',(60.4404467789386,249.91903129069,27.6188837045809)) ;
#109044=CARTESIAN_POINT('Ctrl Pts',(60.4428319502743,249.937545285353,27.6274555764535)) ;
#109045=CARTESIAN_POINT('Ctrl Pts',(60.4520052987548,249.97268088996,27.6436380121775)) ;
#109046=CARTESIAN_POINT('Ctrl Pts',(60.4586423249844,249.989505329671,27.6513456347974)) ;
#109047=CARTESIAN_POINT('Ctrl Pts',(60.4774783235665,250.022559616025,27.6664219076506)) ;
#109048=CARTESIAN_POINT('Ctrl Pts',(60.4902886559452,250.038671895832,27.6737287158086)) ;
#109049=CARTESIAN_POINT('Ctrl Pts',(60.5183067650571,250.062085528376,27.6843112161272)) ;
#109050=CARTESIAN_POINT('Ctrl Pts',(60.5322233323112,250.070462900348,27.6880838741351)) ;
#109051=CARTESIAN_POINT('Ctrl Pts',(60.5612197979218,250.08106143577,27.6928518010587)) ;
#109052=CARTESIAN_POINT('Ctrl Pts',(60.5755858845328,250.083712025825,27.6940416805491)) ;
#109053=CARTESIAN_POINT('Ctrl Pts',(60.5902651077866,250.083712025825,27.6940416805491)) ;
#109054=CARTESIAN_POINT('Origin',(60.5902651077865,249.110257898277,25.1834681346239)) ;
#109055=CARTESIAN_POINT('',(60.5902651077865,250.207872219281,28.0761674639184)) ;
#109056=CARTESIAN_POINT('',(60.5902651077865,249.252916375722,25.1371155854676)) ;
#109057=CARTESIAN_POINT('Ctrl Pts',(60.4402651077865,250.066361548098,28.1260525975113)) ;
#109058=CARTESIAN_POINT('Ctrl Pts',(60.4402651077865,250.067736058265,28.1255643186932)) ;
#109059=CARTESIAN_POINT('Ctrl Pts',(60.440286369022,250.069110537011,28.1250761825189)) ;
#109060=CARTESIAN_POINT('Ctrl Pts',(60.4403288850239,250.07048454529,28.1245883423372)) ;
#109061=CARTESIAN_POINT('Ctrl Pts',(60.4408750760621,250.088136040636,28.1183211976397)) ;
#109062=CARTESIAN_POINT('Ctrl Pts',(60.4449239452533,250.105543020433,28.112162503026)) ;
#109063=CARTESIAN_POINT('Ctrl Pts',(60.4522665395981,250.121800577422,28.1064243414531)) ;
#109064=CARTESIAN_POINT('Ctrl Pts',(60.4599211853138,250.138749060902,28.1004423149599)) ;
#109065=CARTESIAN_POINT('Ctrl Pts',(60.4710122117668,250.154131007314,28.095028961218)) ;
#109066=CARTESIAN_POINT('Ctrl Pts',(60.4849165768428,250.167076875737,28.0904794283365)) ;
#109067=CARTESIAN_POINT('Ctrl Pts',(60.4988172216942,250.180019280389,28.085931112719)) ;
#109068=CARTESIAN_POINT('Ctrl Pts',(60.5152637963998,250.190279214009,28.0823329269325)) ;
#109069=CARTESIAN_POINT('Ctrl Pts',(60.5333315664701,250.197276175373,28.0798802263628)) ;
#109070=CARTESIAN_POINT('Ctrl Pts',(60.5513971100608,250.204272274506,28.0774278280377)) ;
#109071=CARTESIAN_POINT('Ctrl Pts',(60.5707376338848,250.20787221928,28.0761674639187)) ;
#109072=CARTESIAN_POINT('Ctrl Pts',(60.5902651077865,250.20787221928,28.0761674639188)) ;
#109073=CARTESIAN_POINT('Origin',(60.5902651077865,249.739858576849,28.252131183183)) ;
#109074=CARTESIAN_POINT('Origin',(60.5902651077865,249.739858576849,28.252131183183)) ;
#109075=CARTESIAN_POINT('Origin',(60.5902651077865,244.807446220178,27.4709138126218)) ;
#109076=CARTESIAN_POINT('Origin',(60.5902651077865,248.040265107786,23.0213203435596)) ;
#109077=CARTESIAN_POINT('',(60.5902651077865,248.539748311783,28.096802244712)) ;
#109078=CARTESIAN_POINT('Origin',(60.5902651077865,248.040265107786,23.0213203435596)) ;
#109079=CARTESIAN_POINT('Ctrl Pts',(60.4402651077865,248.389748311783,27.9589677074491)) ;
#109080=CARTESIAN_POINT('Ctrl Pts',(60.4402651077865,248.390325382447,27.9595053771305)) ;
#109081=CARTESIAN_POINT('Ctrl Pts',(60.4402684378921,248.390902501024,27.9600430036291)) ;
#109082=CARTESIAN_POINT('Ctrl Pts',(60.4404467789386,248.406352717361,27.974433616113)) ;
#109083=CARTESIAN_POINT('Ctrl Pts',(60.4428319502743,248.421311718545,27.9883070896991)) ;
#109084=CARTESIAN_POINT('Ctrl Pts',(60.4520052987548,248.449727016612,28.014554999575)) ;
#109085=CARTESIAN_POINT('Ctrl Pts',(60.4586423249844,248.463346223256,28.027084422084)) ;
#109086=CARTESIAN_POINT('Ctrl Pts',(60.4774783235664,248.490123893161,28.0516371458428)) ;
#109087=CARTESIAN_POINT('Ctrl Pts',(60.4902886559451,248.503189653969,28.0635653016335)) ;
#109088=CARTESIAN_POINT('Ctrl Pts',(60.5183067650572,248.522187169328,28.0808650678765)) ;
#109089=CARTESIAN_POINT('Ctrl Pts',(60.5322233323113,248.528988708093,28.087041829166)) ;
#109090=CARTESIAN_POINT('Ctrl Pts',(60.5612197979217,248.537595143822,28.0948515246968)) ;
#109091=CARTESIAN_POINT('Ctrl Pts',(60.5755858845327,248.539748311783,28.096802244712)) ;
#109092=CARTESIAN_POINT('Ctrl Pts',(60.5902651077865,248.539748311783,28.096802244712)) ;
#109093=CARTESIAN_POINT('Origin',(60.5902651077865,248.389748311783,25.4082910455649)) ;
#109094=CARTESIAN_POINT('',(60.5902651077865,248.539748311783,28.4985930708324)) ;
#109095=CARTESIAN_POINT('',(60.5902651077865,248.539748311783,25.4082910455649)) ;
#109096=CARTESIAN_POINT('Ctrl Pts',(60.4402651077865,248.389748311783,28.5023074499214)) ;
#109097=CARTESIAN_POINT('Ctrl Pts',(60.4402651077865,248.391206435086,28.5022678161702)) ;
#109098=CARTESIAN_POINT('Ctrl Pts',(60.440286369022,248.392664484427,28.5022283083715)) ;
#109099=CARTESIAN_POINT('Ctrl Pts',(60.4403288850238,248.394121994861,28.5021889366964)) ;
#109100=CARTESIAN_POINT('Ctrl Pts',(60.440875076062,248.412846218751,28.501683139933)) ;
#109101=CARTESIAN_POINT('Ctrl Pts',(60.4449239452532,248.431304381614,28.5012049258673)) ;
#109102=CARTESIAN_POINT('Ctrl Pts',(60.4522665395979,248.44853942657,28.5007714713081)) ;
#109103=CARTESIAN_POINT('Ctrl Pts',(60.4599211853135,248.466506940072,28.5003195954549)) ;
#109104=CARTESIAN_POINT('Ctrl Pts',(60.4710122117664,248.482808858743,28.4999244729506)) ;
#109105=CARTESIAN_POINT('Ctrl Pts',(60.4849165768423,248.496526994243,28.499598103407)) ;
#109106=CARTESIAN_POINT('Ctrl Pts',(60.4988172216937,248.510241459345,28.4992718211862)) ;
#109107=CARTESIAN_POINT('Ctrl Pts',(60.5152637963994,248.521111136629,28.4990202369969)) ;
#109108=CARTESIAN_POINT('Ctrl Pts',(60.5333315664697,248.528523568487,28.4988497601079)) ;
#109109=CARTESIAN_POINT('Ctrl Pts',(60.5513971100605,248.535935086915,28.4986793042266)) ;
#109110=CARTESIAN_POINT('Ctrl Pts',(60.5707376338847,248.539748311783,28.4985930708331)) ;
#109111=CARTESIAN_POINT('Ctrl Pts',(60.5902651077865,248.539748311783,28.4985930708331)) ;
#109112=CARTESIAN_POINT('Origin',(60.5902651077865,248.040265107786,28.5213203435596)) ;
#109113=CARTESIAN_POINT('Origin',(60.5902651077865,248.040265107786,28.5213203435596)) ;
#109114=CARTESIAN_POINT('Origin',(60.5902651077865,246.340671638724,28.252131183183)) ;
#109115=CARTESIAN_POINT('Origin',(60.5902651077865,246.340671638724,28.252131183183)) ;
#109116=CARTESIAN_POINT('Origin',(60.4402651077865,248.040265107786,23.0213203435596)) ;
#109117=CARTESIAN_POINT('',(60.4402651077865,247.54078190379,28.096802244712)) ;
#109118=CARTESIAN_POINT('',(60.4402651077865,246.946891701628,28.0027392774284)) ;
#109119=CARTESIAN_POINT('Origin',(60.4402651077865,247.040072839737,27.7159572226947)) ;
#109120=CARTESIAN_POINT('',(60.4402651077865,246.822731508173,28.3848650607978)) ;
#109121=CARTESIAN_POINT('Origin',(60.4402651077865,246.340671638724,28.252131183183)) ;
#109122=CARTESIAN_POINT('',(60.4402651077865,245.872657996292,28.0761674639184)) ;
#109123=CARTESIAN_POINT('Origin',(60.4402651077865,245.872657996292,28.0761674639184)) ;
#109124=CARTESIAN_POINT('Origin',(60.4402651077865,250.442227059934,18.8655317564881)) ;
#109125=CARTESIAN_POINT('',(60.4402651077865,250.619468117123,18.6215803698081)) ;
#109126=CARTESIAN_POINT('',(60.4402651077865,250.855634839223,18.2965247632928)) ;
#109127=CARTESIAN_POINT('Origin',(60.4402651077865,251.663815640099,18.8837024854464)) ;
#109128=CARTESIAN_POINT('',(60.4402651077865,251.663815640099,18.8837024854464)) ;
#109129=CARTESIAN_POINT('',(60.4402651077865,251.427648917999,19.2087580919617)) ;
#109130=CARTESIAN_POINT('Origin',(60.4402651077865,251.273083995395,18.5717268744974)) ;
#109131=CARTESIAN_POINT('Origin',(60.4402651077865,251.608875972704,19.811177590536)) ;
#109132=CARTESIAN_POINT('',(60.4402651077865,251.852827359384,19.6339365333471)) ;
#109133=CARTESIAN_POINT('',(60.4402651077865,252.1778829659,19.3977698112471)) ;
#109134=CARTESIAN_POINT('Origin',(60.4402651077865,252.765060688053,20.2059506121228)) ;
#109135=CARTESIAN_POINT('',(60.4402651077865,252.765060688053,20.2059506121228)) ;
#109136=CARTESIAN_POINT('',(60.4402651077865,252.440005081538,20.4421173342227)) ;
#109137=CARTESIAN_POINT('Origin',(60.4402651077865,252.489858576849,19.788501455951)) ;
#109138=CARTESIAN_POINT('Origin',(60.4402651077865,252.426204390042,21.0710545636296)) ;
#109139=CARTESIAN_POINT('',(60.4402651077865,252.712986444776,20.9778734255204)) ;
#109140=CARTESIAN_POINT('',(60.4402651077865,253.095112228145,20.8537132320653)) ;
#109141=CARTESIAN_POINT('Origin',(60.4402651077865,253.403809825024,21.8037867439466)) ;
#109142=CARTESIAN_POINT('',(60.4402651077865,253.403809825024,21.8037867439466)) ;
#109143=CARTESIAN_POINT('',(60.4402651077865,253.021684041655,21.9279469374017)) ;
#109144=CARTESIAN_POINT('Origin',(60.4402651077865,253.27107594741,21.3217268744974)) ;
#109145=CARTESIAN_POINT('Origin',(60.4402651077865,252.814206511797,22.5218371395634)) ;
#109146=CARTESIAN_POINT('',(60.4402651077865,253.115747008939,22.5218371395634)) ;
#109147=CARTESIAN_POINT('',(60.4402651077865,253.517537835059,22.5218371395634)) ;
#109148=CARTESIAN_POINT('Origin',(60.4402651077865,253.517537835059,23.5208035475559)) ;
#109149=CARTESIAN_POINT('',(60.4402651077865,253.517537835059,23.5208035475559)) ;
#109150=CARTESIAN_POINT('',(60.4402651077865,253.115747008939,23.5208035475559)) ;
#109151=CARTESIAN_POINT('Origin',(60.4402651077865,253.540265107786,23.0213203435596)) ;
#109152=CARTESIAN_POINT('Origin',(60.4402651077865,252.734901986921,24.0215126116084)) ;
#109153=CARTESIAN_POINT('',(60.4402651077865,253.021684041655,24.1146937497175)) ;
#109154=CARTESIAN_POINT('',(60.4402651077865,253.403809825024,24.2388539431727)) ;
#109155=CARTESIAN_POINT('Origin',(60.4402651077865,253.095112228145,25.188927455054)) ;
#109156=CARTESIAN_POINT('',(60.4402651077865,253.095112228145,25.188927455054)) ;
#109157=CARTESIAN_POINT('',(60.4402651077865,252.712986444776,25.0647672615988)) ;
#109158=CARTESIAN_POINT('Origin',(60.4402651077865,253.27107594741,24.7209138126218)) ;
#109159=CARTESIAN_POINT('Origin',(60.4402651077865,252.196053694858,25.4232822957076)) ;
#109160=CARTESIAN_POINT('',(60.4402651077865,252.440005081538,25.6005233528965)) ;
#109161=CARTESIAN_POINT('',(60.4402651077865,252.765060688053,25.8366900749965)) ;
#109162=CARTESIAN_POINT('Origin',(60.4402651077865,252.1778829659,26.6448708758722)) ;
#109163=CARTESIAN_POINT('',(60.4402651077865,252.1778829659,26.6448708758722)) ;
#109164=CARTESIAN_POINT('',(60.4402651077865,251.852827359384,26.4087041537722)) ;
#109165=CARTESIAN_POINT('Origin',(60.4402651077865,252.489858576849,26.2541392311682)) ;
#109166=CARTESIAN_POINT('Origin',(60.4402651077865,251.25040786081,26.5899312084775)) ;
#109167=CARTESIAN_POINT('',(60.4402651077865,251.427648917999,26.8338825951576)) ;
#109168=CARTESIAN_POINT('',(60.4402651077865,251.663815640099,27.1589382016729)) ;
#109169=CARTESIAN_POINT('Origin',(60.4402651077865,250.855634839223,27.7461159238265)) ;
#109170=CARTESIAN_POINT('',(60.4402651077865,250.855634839223,27.7461159238265)) ;
#109171=CARTESIAN_POINT('',(60.4402651077865,250.619468117123,27.4210603173112)) ;
#109172=CARTESIAN_POINT('Origin',(60.4402651077865,251.273083995395,27.4709138126218)) ;
#109173=CARTESIAN_POINT('Origin',(60.4402651077865,249.990530887716,27.4072596258153)) ;
#109174=CARTESIAN_POINT('',(60.4402651077865,250.083712025826,27.694041680549)) ;
#109175=CARTESIAN_POINT('',(60.4402651077865,250.207872219281,28.0761674639184)) ;
#109176=CARTESIAN_POINT('Origin',(60.4402651077865,249.257798707399,28.3848650607978)) ;
#109177=CARTESIAN_POINT('',(60.4402651077865,249.257798707399,28.3848650607978)) ;
#109178=CARTESIAN_POINT('',(60.4402651077865,249.133638513944,28.0027392774284)) ;
#109179=CARTESIAN_POINT('Origin',(60.4402651077865,249.739858576849,28.252131183183)) ;
#109180=CARTESIAN_POINT('Origin',(60.4402651077865,248.539748311783,27.7952617475701)) ;
#109181=CARTESIAN_POINT('',(60.4402651077865,248.539748311783,28.096802244712)) ;
#109182=CARTESIAN_POINT('',(60.4402651077865,248.539748311783,28.4985930708324)) ;
#109183=CARTESIAN_POINT('Origin',(60.4402651077865,247.54078190379,28.4985930708324)) ;
#109184=CARTESIAN_POINT('',(60.4402651077865,247.54078190379,28.4985930708324)) ;
#109185=CARTESIAN_POINT('Origin',(60.4402651077865,248.040265107786,28.5213203435596)) ;
#109186=CARTESIAN_POINT('Origin',(60.4402651077865,248.040265107786,23.0213203435596)) ;
#109187=CARTESIAN_POINT('Origin',(60.4402651077865,248.040265107786,23.0213203435596)) ;
#109188=CARTESIAN_POINT('Origin',(60.4402651077865,248.040265107786,23.0213203435596)) ;
#109189=CARTESIAN_POINT('Origin',(60.4402651077865,248.040265107786,23.0213203435596)) ;
#109190=CARTESIAN_POINT('Origin',(60.4402651077865,248.040265107786,23.0213203435596)) ;
#109191=CARTESIAN_POINT('Origin',(60.4402651077865,248.040265107786,23.0213203435596)) ;
#109192=CARTESIAN_POINT('Origin',(60.4402651077865,248.040265107786,23.0213203435596)) ;
#109193=CARTESIAN_POINT('Origin',(60.4402651077865,248.040265107786,23.0213203435596)) ;
#109194=CARTESIAN_POINT('Origin',(60.4402651077865,248.040265107786,23.0213203435596)) ;
#109195=CARTESIAN_POINT('Origin',(59.9402651077865,248.040265107786,23.0213203435596)) ;
#109196=CARTESIAN_POINT('',(59.9402651077865,250.040265107786,23.0213203435596)) ;
#117145=UNCERTAINTY_MEASURE_WITH_UNIT(LENGTH_MEASURE(0.01),#117171,
'DISTANCE_ACCURACY_VALUE',
'Maximum model space distance between geometric entities at asserted c
onnectivities') ;
#117147=UNCERTAINTY_MEASURE_WITH_UNIT(LENGTH_MEASURE(0.01),#117171,
'DISTANCE_ACCURACY_VALUE',
'Maximum model space distance between geometric entities at asserted c
onnectivities') ;
#117168=(
GEOMETRIC_REPRESENTATION_CONTEXT(3)
GLOBAL_UNCERTAINTY_ASSIGNED_CONTEXT((#117145))
GLOBAL_UNIT_ASSIGNED_CONTEXT((#117171,#117173,#117174))
REPRESENTATION_CONTEXT('','3D')
) ;
#117170=(
GEOMETRIC_REPRESENTATION_CONTEXT(3)
GLOBAL_UNCERTAINTY_ASSIGNED_CONTEXT((#117147))
GLOBAL_UNIT_ASSIGNED_CONTEXT((#117171,#117173,#117174))
REPRESENTATION_CONTEXT('','3D')
) ;
#117171=(
LENGTH_UNIT()
NAMED_UNIT(*)
SI_UNIT(.MILLI.,.METRE.)
) ;
#117173=(
NAMED_UNIT(*)
PLANE_ANGLE_UNIT()
SI_UNIT($,.RADIAN.)
) ;
#117174=(
NAMED_UNIT(*)
SI_UNIT($,.STERADIAN.)
SOLID_ANGLE_UNIT()
) ;
#117195=SHAPE_DEFINITION_REPRESENTATION(#117217,#117260) ;
#117217=PRODUCT_DEFINITION_SHAPE('',$,#117283) ;
#117260=SHAPE_REPRESENTATION('',(#54544),#117168) ;
#117262=PRODUCT_DEFINITION_CONTEXT('part definition',#117330,'design') ;
#117283=PRODUCT_DEFINITION('Knob_Grip_2','Knob_Grip_2',#117305,#117262) ;
#117305=PRODUCT_DEFINITION_FORMATION('',$,#117352) ;
#117330=APPLICATION_CONTEXT(
'Core Data for Automotive Mechanical Design Process') ;
#117331=PRODUCT_CONTEXT('part definition',#117330,'mechanical') ;
#117352=PRODUCT('Knob_Grip_2','Knob_Grip_2',$,(#117331)) ;
#117355=PRESENTATION_STYLE_ASSIGNMENT((#117357)) ;
#117357=SURFACE_STYLE_USAGE(.BOTH.,#117359) ;
#117359=SURFACE_SIDE_STYLE('',(#117361)) ;
#117361=SURFACE_STYLE_FILL_AREA(#117363) ;
#117363=FILL_AREA_STYLE('Opaque(160,160,160)',(#117365)) ;
#117365=FILL_AREA_STYLE_COLOUR('Opaque(160,160,160)',#117367) ;
#117367=COLOUR_RGB('Opaque(160,160,160)', 0.09019608, 0.27058824, 0.51372549) ;
ENDSEC;
END-ISO-10303-21;
